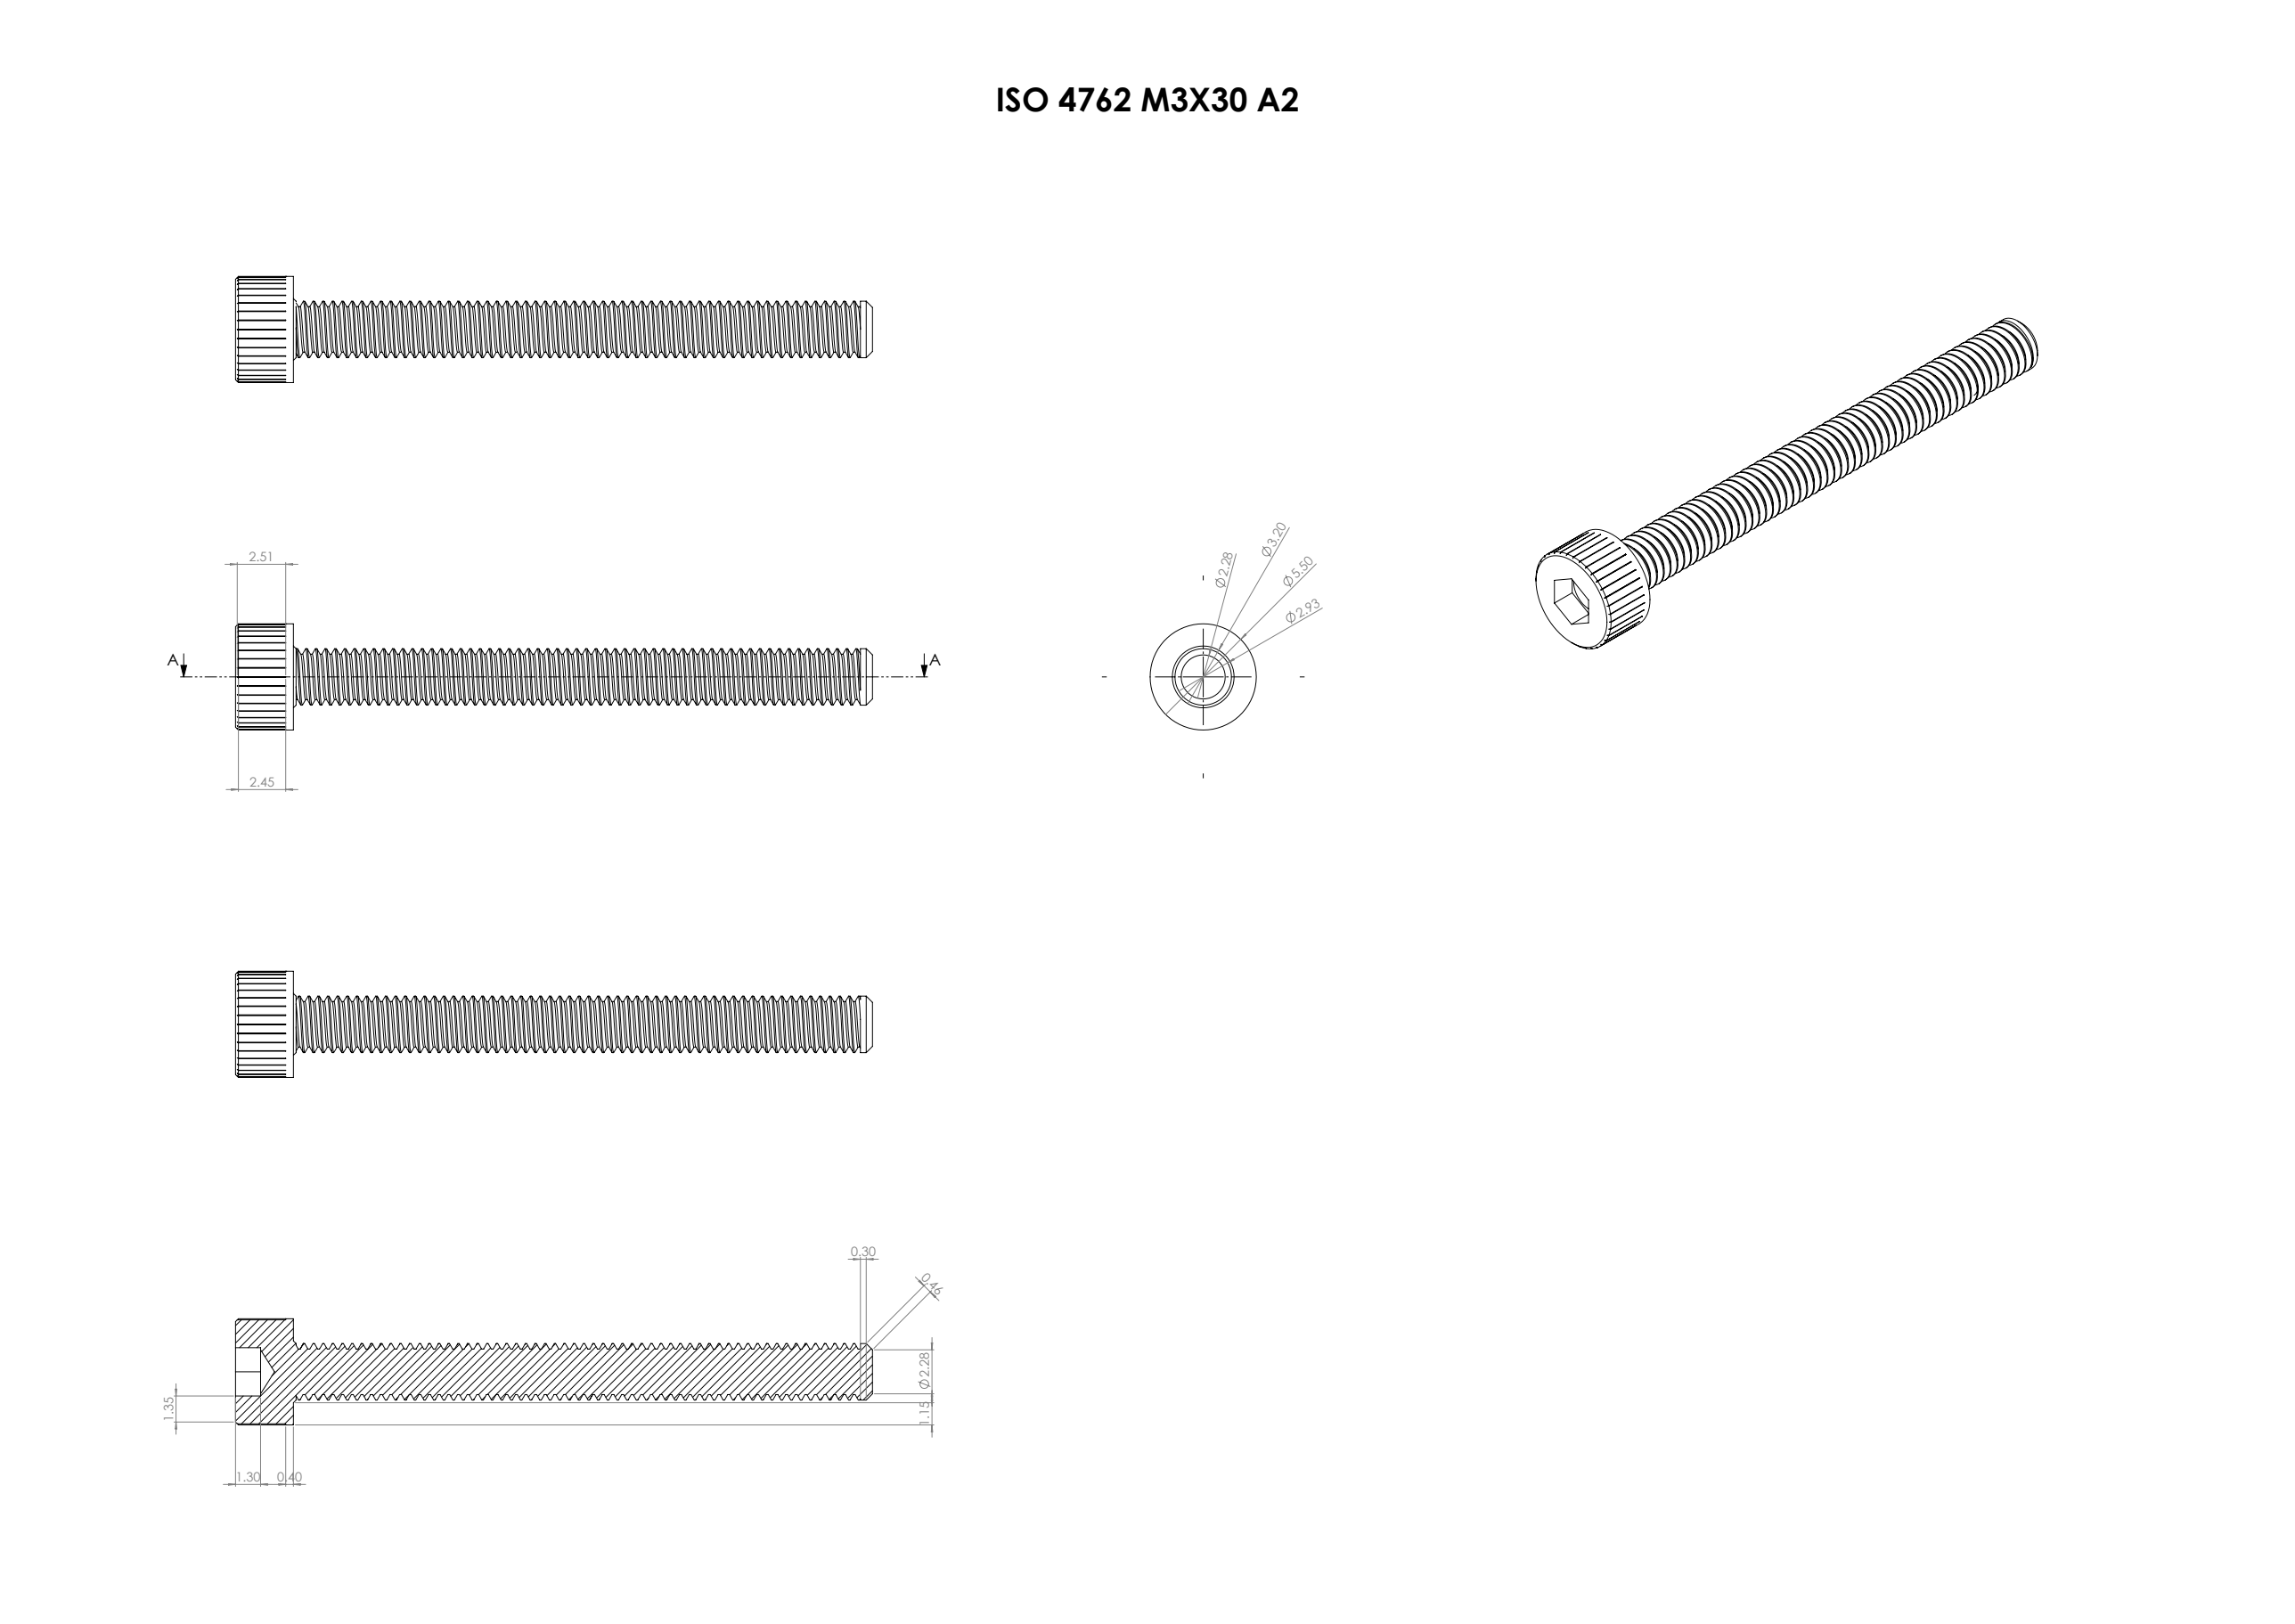
ISO-10303-21;
HEADER;
/* Generated by software containing ST-Developer
 * from STEP Tools, Inc. (www.steptools.com) 
 */

FILE_DESCRIPTION(
/* description */ (''),
/* implementation_level */ '2;1');

FILE_NAME(
/* name */ '15_ISO_4762_M3x30_A2.step',
/* time_stamp */ '2026-10-19T22:59:19-07:00',
/* author */ (''),
/* organization */ (''),
/* preprocessor_version */ 'ST-DEVELOPER v20.2',
/* originating_system */ 'Autodesk Translation Framework v15.15.0.0',
/* authorisation */ '');

FILE_SCHEMA (('AUTOMOTIVE_DESIGN { 1 0 10303 214 3 1 1 }'));
ENDSEC;

DATA;
#10=MECHANICAL_DESIGN_GEOMETRIC_PRESENTATION_REPRESENTATION('',(#925),#53650);
#219=(
BOUNDED_CURVE()
B_SPLINE_CURVE(2,(#49244,#49245,#49246),.UNSPECIFIED.,.F.,.F.)
B_SPLINE_CURVE_WITH_KNOTS((3,3),(0.,0.00848409808460555),.UNSPECIFIED.)
CURVE()
GEOMETRIC_REPRESENTATION_ITEM()
RATIONAL_B_SPLINE_CURVE((1.,1.00016582969981,1.00020138402525))
REPRESENTATION_ITEM('')
);
#220=(
BOUNDED_CURVE()
B_SPLINE_CURVE(2,(#49250,#49251,#49252),.UNSPECIFIED.,.F.,.F.)
B_SPLINE_CURVE_WITH_KNOTS((3,3),(0.0131150022108642,0.0215991002954745),
 .UNSPECIFIED.)
CURVE()
GEOMETRIC_REPRESENTATION_ITEM()
RATIONAL_B_SPLINE_CURVE((1.0002013840307,1.00016582970429,1.))
REPRESENTATION_ITEM('')
);
#221=(
BOUNDED_CURVE()
B_SPLINE_CURVE(2,(#49265,#49266,#49267),.UNSPECIFIED.,.F.,.F.)
B_SPLINE_CURVE_WITH_KNOTS((3,3),(0.,0.0084840980845983),.UNSPECIFIED.)
CURVE()
GEOMETRIC_REPRESENTATION_ITEM()
RATIONAL_B_SPLINE_CURVE((1.,1.00016582970166,1.00020138402749))
REPRESENTATION_ITEM('')
);
#222=(
BOUNDED_CURVE()
B_SPLINE_CURVE(2,(#49271,#49272,#49273),.UNSPECIFIED.,.F.,.F.)
B_SPLINE_CURVE_WITH_KNOTS((3,3),(0.0131150022108621,0.0215991002954745),
 .UNSPECIFIED.)
CURVE()
GEOMETRIC_REPRESENTATION_ITEM()
RATIONAL_B_SPLINE_CURVE((1.00020138404061,1.00016582971246,1.))
REPRESENTATION_ITEM('')
);
#223=(
BOUNDED_CURVE()
B_SPLINE_CURVE(2,(#49286,#49287,#49288),.UNSPECIFIED.,.F.,.F.)
B_SPLINE_CURVE_WITH_KNOTS((3,3),(0.,0.0084840980847528),.UNSPECIFIED.)
CURVE()
GEOMETRIC_REPRESENTATION_ITEM()
RATIONAL_B_SPLINE_CURVE((1.,1.00016582970549,1.00020138403215))
REPRESENTATION_ITEM('')
);
#224=(
BOUNDED_CURVE()
B_SPLINE_CURVE(2,(#49292,#49293,#49294),.UNSPECIFIED.,.F.,.F.)
B_SPLINE_CURVE_WITH_KNOTS((3,3),(0.0131150022108369,0.0215991002954744),
 .UNSPECIFIED.)
CURVE()
GEOMETRIC_REPRESENTATION_ITEM()
RATIONAL_B_SPLINE_CURVE((1.00020138403309,1.00016582970627,1.))
REPRESENTATION_ITEM('')
);
#225=(
BOUNDED_CURVE()
B_SPLINE_CURVE(2,(#49307,#49308,#49309),.UNSPECIFIED.,.F.,.F.)
B_SPLINE_CURVE_WITH_KNOTS((3,3),(0.,0.00848409808456441),.UNSPECIFIED.)
CURVE()
GEOMETRIC_REPRESENTATION_ITEM()
RATIONAL_B_SPLINE_CURVE((1.,1.00016582971128,1.00020138403918))
REPRESENTATION_ITEM('')
);
#226=(
BOUNDED_CURVE()
B_SPLINE_CURVE(2,(#49313,#49314,#49315),.UNSPECIFIED.,.F.,.F.)
B_SPLINE_CURVE_WITH_KNOTS((3,3),(0.0131150022107445,0.0215991002954745),
 .UNSPECIFIED.)
CURVE()
GEOMETRIC_REPRESENTATION_ITEM()
RATIONAL_B_SPLINE_CURVE((1.00020138401994,1.00016582969544,1.))
REPRESENTATION_ITEM('')
);
#227=(
BOUNDED_CURVE()
B_SPLINE_CURVE(2,(#49328,#49329,#49330),.UNSPECIFIED.,.F.,.F.)
B_SPLINE_CURVE_WITH_KNOTS((3,3),(0.,0.00848409808454028),.UNSPECIFIED.)
CURVE()
GEOMETRIC_REPRESENTATION_ITEM()
RATIONAL_B_SPLINE_CURVE((1.,1.00016582970383,1.00020138403013))
REPRESENTATION_ITEM('')
);
#228=(
BOUNDED_CURVE()
B_SPLINE_CURVE(2,(#49334,#49335,#49336),.UNSPECIFIED.,.F.,.F.)
B_SPLINE_CURVE_WITH_KNOTS((3,3),(0.0131150022108609,0.0215991002954744),
 .UNSPECIFIED.)
CURVE()
GEOMETRIC_REPRESENTATION_ITEM()
RATIONAL_B_SPLINE_CURVE((1.00020138403313,1.0001658297063,1.))
REPRESENTATION_ITEM('')
);
#229=(
BOUNDED_CURVE()
B_SPLINE_CURVE(2,(#49349,#49350,#49351),.UNSPECIFIED.,.F.,.F.)
B_SPLINE_CURVE_WITH_KNOTS((3,3),(0.,0.00848409808447202),.UNSPECIFIED.)
CURVE()
GEOMETRIC_REPRESENTATION_ITEM()
RATIONAL_B_SPLINE_CURVE((1.,1.00016582970768,1.00020138403481))
REPRESENTATION_ITEM('')
);
#230=(
BOUNDED_CURVE()
B_SPLINE_CURVE(2,(#49355,#49356,#49357),.UNSPECIFIED.,.F.,.F.)
B_SPLINE_CURVE_WITH_KNOTS((3,3),(0.0131150022108224,0.0215991002954744),
 .UNSPECIFIED.)
CURVE()
GEOMETRIC_REPRESENTATION_ITEM()
RATIONAL_B_SPLINE_CURVE((1.00020138403609,1.00016582970874,1.))
REPRESENTATION_ITEM('')
);
#231=(
BOUNDED_CURVE()
B_SPLINE_CURVE(2,(#49370,#49371,#49372),.UNSPECIFIED.,.F.,.F.)
B_SPLINE_CURVE_WITH_KNOTS((3,3),(0.,0.00848409808427833),.UNSPECIFIED.)
CURVE()
GEOMETRIC_REPRESENTATION_ITEM()
RATIONAL_B_SPLINE_CURVE((1.,1.00016582970634,1.00020138403319))
REPRESENTATION_ITEM('')
);
#232=(
BOUNDED_CURVE()
B_SPLINE_CURVE(2,(#49376,#49377,#49378),.UNSPECIFIED.,.F.,.F.)
B_SPLINE_CURVE_WITH_KNOTS((3,3),(0.013115002210556,0.0215991002954744),
 .UNSPECIFIED.)
CURVE()
GEOMETRIC_REPRESENTATION_ITEM()
RATIONAL_B_SPLINE_CURVE((1.00020138403007,1.00016582970378,1.))
REPRESENTATION_ITEM('')
);
#233=(
BOUNDED_CURVE()
B_SPLINE_CURVE(2,(#49391,#49392,#49393),.UNSPECIFIED.,.F.,.F.)
B_SPLINE_CURVE_WITH_KNOTS((3,3),(0.,0.00848409808441644),.UNSPECIFIED.)
CURVE()
GEOMETRIC_REPRESENTATION_ITEM()
RATIONAL_B_SPLINE_CURVE((1.,1.00016582971078,1.00020138403858))
REPRESENTATION_ITEM('')
);
#234=(
BOUNDED_CURVE()
B_SPLINE_CURVE(2,(#49397,#49398,#49399),.UNSPECIFIED.,.F.,.F.)
B_SPLINE_CURVE_WITH_KNOTS((3,3),(0.0131150022111809,0.0215991002954744),
 .UNSPECIFIED.)
CURVE()
GEOMETRIC_REPRESENTATION_ITEM()
RATIONAL_B_SPLINE_CURVE((1.00020138403856,1.00016582971077,1.))
REPRESENTATION_ITEM('')
);
#235=(
BOUNDED_CURVE()
B_SPLINE_CURVE(2,(#49412,#49413,#49414),.UNSPECIFIED.,.F.,.F.)
B_SPLINE_CURVE_WITH_KNOTS((3,3),(0.,0.00848409808461716),.UNSPECIFIED.)
CURVE()
GEOMETRIC_REPRESENTATION_ITEM()
RATIONAL_B_SPLINE_CURVE((1.,1.00016582970495,1.00020138403149))
REPRESENTATION_ITEM('')
);
#236=(
BOUNDED_CURVE()
B_SPLINE_CURVE(2,(#49418,#49419,#49420),.UNSPECIFIED.,.F.,.F.)
B_SPLINE_CURVE_WITH_KNOTS((3,3),(0.0131150022109262,0.0215991002954744),
 .UNSPECIFIED.)
CURVE()
GEOMETRIC_REPRESENTATION_ITEM()
RATIONAL_B_SPLINE_CURVE((1.00020138404239,1.00016582971392,1.))
REPRESENTATION_ITEM('')
);
#237=(
BOUNDED_CURVE()
B_SPLINE_CURVE(2,(#49433,#49434,#49435),.UNSPECIFIED.,.F.,.F.)
B_SPLINE_CURVE_WITH_KNOTS((3,3),(0.,0.00848409808431464),.UNSPECIFIED.)
CURVE()
GEOMETRIC_REPRESENTATION_ITEM()
RATIONAL_B_SPLINE_CURVE((1.,1.00016582970871,1.00020138403606))
REPRESENTATION_ITEM('')
);
#238=(
BOUNDED_CURVE()
B_SPLINE_CURVE(2,(#49439,#49440,#49441),.UNSPECIFIED.,.F.,.F.)
B_SPLINE_CURVE_WITH_KNOTS((3,3),(0.0131150022106601,0.0215991002954745),
 .UNSPECIFIED.)
CURVE()
GEOMETRIC_REPRESENTATION_ITEM()
RATIONAL_B_SPLINE_CURVE((1.00020138402617,1.00016582970057,1.))
REPRESENTATION_ITEM('')
);
#239=(
BOUNDED_CURVE()
B_SPLINE_CURVE(2,(#49454,#49455,#49456),.UNSPECIFIED.,.F.,.F.)
B_SPLINE_CURVE_WITH_KNOTS((3,3),(0.,0.00848409808479875),.UNSPECIFIED.)
CURVE()
GEOMETRIC_REPRESENTATION_ITEM()
RATIONAL_B_SPLINE_CURVE((1.,1.00016582970535,1.00020138403197))
REPRESENTATION_ITEM('')
);
#240=(
BOUNDED_CURVE()
B_SPLINE_CURVE(2,(#49460,#49461,#49462),.UNSPECIFIED.,.F.,.F.)
B_SPLINE_CURVE_WITH_KNOTS((3,3),(0.0131150022108306,0.0215991002954744),
 .UNSPECIFIED.)
CURVE()
GEOMETRIC_REPRESENTATION_ITEM()
RATIONAL_B_SPLINE_CURVE((1.00020138403405,1.00016582970706,1.))
REPRESENTATION_ITEM('')
);
#241=(
BOUNDED_CURVE()
B_SPLINE_CURVE(2,(#49475,#49476,#49477),.UNSPECIFIED.,.F.,.F.)
B_SPLINE_CURVE_WITH_KNOTS((3,3),(0.,0.0084840980847528),.UNSPECIFIED.)
CURVE()
GEOMETRIC_REPRESENTATION_ITEM()
RATIONAL_B_SPLINE_CURVE((1.,1.00016582970549,1.00020138403215))
REPRESENTATION_ITEM('')
);
#242=(
BOUNDED_CURVE()
B_SPLINE_CURVE(2,(#49481,#49482,#49483),.UNSPECIFIED.,.F.,.F.)
B_SPLINE_CURVE_WITH_KNOTS((3,3),(0.0131150022108369,0.0215991002954744),
 .UNSPECIFIED.)
CURVE()
GEOMETRIC_REPRESENTATION_ITEM()
RATIONAL_B_SPLINE_CURVE((1.00020138403309,1.00016582970627,1.))
REPRESENTATION_ITEM('')
);
#243=(
BOUNDED_CURVE()
B_SPLINE_CURVE(2,(#49496,#49497,#49498),.UNSPECIFIED.,.F.,.F.)
B_SPLINE_CURVE_WITH_KNOTS((3,3),(0.,0.0084840980842322),.UNSPECIFIED.)
CURVE()
GEOMETRIC_REPRESENTATION_ITEM()
RATIONAL_B_SPLINE_CURVE((1.,1.00016582971394,1.00020138404241))
REPRESENTATION_ITEM('')
);
#244=(
BOUNDED_CURVE()
B_SPLINE_CURVE(2,(#49502,#49503,#49504),.UNSPECIFIED.,.F.,.F.)
B_SPLINE_CURVE_WITH_KNOTS((3,3),(0.0131150022105481,0.0215991002954744),
 .UNSPECIFIED.)
CURVE()
GEOMETRIC_REPRESENTATION_ITEM()
RATIONAL_B_SPLINE_CURVE((1.00020138402709,1.00016582970133,1.))
REPRESENTATION_ITEM('')
);
#245=(
BOUNDED_CURVE()
B_SPLINE_CURVE(2,(#49517,#49518,#49519),.UNSPECIFIED.,.F.,.F.)
B_SPLINE_CURVE_WITH_KNOTS((3,3),(0.,0.00848409808414784),.UNSPECIFIED.)
CURVE()
GEOMETRIC_REPRESENTATION_ITEM()
RATIONAL_B_SPLINE_CURVE((1.,1.00016582970969,1.00020138403725))
REPRESENTATION_ITEM('')
);
#246=(
BOUNDED_CURVE()
B_SPLINE_CURVE(2,(#49523,#49524,#49525),.UNSPECIFIED.,.F.,.F.)
B_SPLINE_CURVE_WITH_KNOTS((3,3),(0.0131150022106295,0.0215991002954744),
 .UNSPECIFIED.)
CURVE()
GEOMETRIC_REPRESENTATION_ITEM()
RATIONAL_B_SPLINE_CURVE((1.00020138402686,1.00016582970114,1.))
REPRESENTATION_ITEM('')
);
#247=(
BOUNDED_CURVE()
B_SPLINE_CURVE(2,(#49538,#49539,#49540),.UNSPECIFIED.,.F.,.F.)
B_SPLINE_CURVE_WITH_KNOTS((3,3),(0.,0.00848409808445945),.UNSPECIFIED.)
CURVE()
GEOMETRIC_REPRESENTATION_ITEM()
RATIONAL_B_SPLINE_CURVE((1.,1.00016582971029,1.00020138403798))
REPRESENTATION_ITEM('')
);
#248=(
BOUNDED_CURVE()
B_SPLINE_CURVE(2,(#49544,#49545,#49546),.UNSPECIFIED.,.F.,.F.)
B_SPLINE_CURVE_WITH_KNOTS((3,3),(0.0131150022108553,0.0215991002954744),
 .UNSPECIFIED.)
CURVE()
GEOMETRIC_REPRESENTATION_ITEM()
RATIONAL_B_SPLINE_CURVE((1.00020138402807,1.00016582970213,1.))
REPRESENTATION_ITEM('')
);
#249=(
BOUNDED_CURVE()
B_SPLINE_CURVE(2,(#49559,#49560,#49561),.UNSPECIFIED.,.F.,.F.)
B_SPLINE_CURVE_WITH_KNOTS((3,3),(0.,0.00848409808448244),.UNSPECIFIED.)
CURVE()
GEOMETRIC_REPRESENTATION_ITEM()
RATIONAL_B_SPLINE_CURVE((1.,1.00016582970044,1.00020138402602))
REPRESENTATION_ITEM('')
);
#250=(
BOUNDED_CURVE()
B_SPLINE_CURVE(2,(#49565,#49566,#49567),.UNSPECIFIED.,.F.,.F.)
B_SPLINE_CURVE_WITH_KNOTS((3,3),(0.0131150022107,0.0215991002954745),
 .UNSPECIFIED.)
CURVE()
GEOMETRIC_REPRESENTATION_ITEM()
RATIONAL_B_SPLINE_CURVE((1.00020138402745,1.00016582970163,1.))
REPRESENTATION_ITEM('')
);
#251=(
BOUNDED_CURVE()
B_SPLINE_CURVE(2,(#49580,#49581,#49582),.UNSPECIFIED.,.F.,.F.)
B_SPLINE_CURVE_WITH_KNOTS((3,3),(0.,0.0084840980844404),.UNSPECIFIED.)
CURVE()
GEOMETRIC_REPRESENTATION_ITEM()
RATIONAL_B_SPLINE_CURVE((1.,1.00016582969984,1.00020138402529))
REPRESENTATION_ITEM('')
);
#252=(
BOUNDED_CURVE()
B_SPLINE_CURVE(2,(#49586,#49587,#49588),.UNSPECIFIED.,.F.,.F.)
B_SPLINE_CURVE_WITH_KNOTS((3,3),(0.0131150022109728,0.0215991002954744),
 .UNSPECIFIED.)
CURVE()
GEOMETRIC_REPRESENTATION_ITEM()
RATIONAL_B_SPLINE_CURVE((1.00020138403593,1.0001658297086,1.))
REPRESENTATION_ITEM('')
);
#253=(
BOUNDED_CURVE()
B_SPLINE_CURVE(2,(#49603,#49604,#49605),.UNSPECIFIED.,.F.,.F.)
B_SPLINE_CURVE_WITH_KNOTS((3,3),(0.,0.00848409808461716),.UNSPECIFIED.)
CURVE()
GEOMETRIC_REPRESENTATION_ITEM()
RATIONAL_B_SPLINE_CURVE((1.,1.00016582970494,1.00020138403149))
REPRESENTATION_ITEM('')
);
#254=(
BOUNDED_CURVE()
B_SPLINE_CURVE(2,(#49609,#49610,#49611),.UNSPECIFIED.,.F.,.F.)
B_SPLINE_CURVE_WITH_KNOTS((3,3),(0.0131150022107313,0.0215991002954744),
 .UNSPECIFIED.)
CURVE()
GEOMETRIC_REPRESENTATION_ITEM()
RATIONAL_B_SPLINE_CURVE((1.00020138404435,1.00016582971554,1.))
REPRESENTATION_ITEM('')
);
#255=(
BOUNDED_CURVE()
B_SPLINE_CURVE(2,(#49624,#49625,#49626),.UNSPECIFIED.,.F.,.F.)
B_SPLINE_CURVE_WITH_KNOTS((3,3),(0.,0.0084840980847339),.UNSPECIFIED.)
CURVE()
GEOMETRIC_REPRESENTATION_ITEM()
RATIONAL_B_SPLINE_CURVE((1.,1.00016582970597,1.00020138403273))
REPRESENTATION_ITEM('')
);
#256=(
BOUNDED_CURVE()
B_SPLINE_CURVE(2,(#49630,#49631,#49632),.UNSPECIFIED.,.F.,.F.)
B_SPLINE_CURVE_WITH_KNOTS((3,3),(0.0131150022106966,0.0215991002954744),
 .UNSPECIFIED.)
CURVE()
GEOMETRIC_REPRESENTATION_ITEM()
RATIONAL_B_SPLINE_CURVE((1.00020138403392,1.00016582970695,1.))
REPRESENTATION_ITEM('')
);
#257=(
BOUNDED_CURVE()
B_SPLINE_CURVE(2,(#49645,#49646,#49647),.UNSPECIFIED.,.F.,.F.)
B_SPLINE_CURVE_WITH_KNOTS((3,3),(0.,0.00848409808458664),.UNSPECIFIED.)
CURVE()
GEOMETRIC_REPRESENTATION_ITEM()
RATIONAL_B_SPLINE_CURVE((1.,1.00016582970477,1.00020138403127))
REPRESENTATION_ITEM('')
);
#258=(
BOUNDED_CURVE()
B_SPLINE_CURVE(2,(#49651,#49652,#49653),.UNSPECIFIED.,.F.,.F.)
B_SPLINE_CURVE_WITH_KNOTS((3,3),(0.0131150022108393,0.0215991002954745),
 .UNSPECIFIED.)
CURVE()
GEOMETRIC_REPRESENTATION_ITEM()
RATIONAL_B_SPLINE_CURVE((1.00020138403572,1.00016582970843,1.))
REPRESENTATION_ITEM('')
);
#259=(
BOUNDED_CURVE()
B_SPLINE_CURVE(2,(#49666,#49667,#49668),.UNSPECIFIED.,.F.,.F.)
B_SPLINE_CURVE_WITH_KNOTS((3,3),(0.,0.00848409808463718),.UNSPECIFIED.)
CURVE()
GEOMETRIC_REPRESENTATION_ITEM()
RATIONAL_B_SPLINE_CURVE((1.,1.00016582970055,1.00020138402615))
REPRESENTATION_ITEM('')
);
#260=(
BOUNDED_CURVE()
B_SPLINE_CURVE(2,(#49672,#49673,#49674),.UNSPECIFIED.,.F.,.F.)
B_SPLINE_CURVE_WITH_KNOTS((3,3),(0.013115002211021,0.0215991002954743),
 .UNSPECIFIED.)
CURVE()
GEOMETRIC_REPRESENTATION_ITEM()
RATIONAL_B_SPLINE_CURVE((1.00020138403351,1.00016582970661,1.))
REPRESENTATION_ITEM('')
);
#261=(
BOUNDED_CURVE()
B_SPLINE_CURVE(2,(#49687,#49688,#49689),.UNSPECIFIED.,.F.,.F.)
B_SPLINE_CURVE_WITH_KNOTS((3,3),(0.,0.0084840980842322),.UNSPECIFIED.)
CURVE()
GEOMETRIC_REPRESENTATION_ITEM()
RATIONAL_B_SPLINE_CURVE((1.,1.00016582971394,1.00020138404241))
REPRESENTATION_ITEM('')
);
#262=(
BOUNDED_CURVE()
B_SPLINE_CURVE(2,(#49693,#49694,#49695),.UNSPECIFIED.,.F.,.F.)
B_SPLINE_CURVE_WITH_KNOTS((3,3),(0.0131150022105481,0.0215991002954744),
 .UNSPECIFIED.)
CURVE()
GEOMETRIC_REPRESENTATION_ITEM()
RATIONAL_B_SPLINE_CURVE((1.00020138402709,1.00016582970133,1.))
REPRESENTATION_ITEM('')
);
#263=(
BOUNDED_CURVE()
B_SPLINE_CURVE(2,(#49708,#49709,#49710),.UNSPECIFIED.,.F.,.F.)
B_SPLINE_CURVE_WITH_KNOTS((3,3),(0.,0.00848409808456074),.UNSPECIFIED.)
CURVE()
GEOMETRIC_REPRESENTATION_ITEM()
RATIONAL_B_SPLINE_CURVE((1.,1.00016582970947,1.00020138403699))
REPRESENTATION_ITEM('')
);
#264=(
BOUNDED_CURVE()
B_SPLINE_CURVE(2,(#49714,#49715,#49716),.UNSPECIFIED.,.F.,.F.)
B_SPLINE_CURVE_WITH_KNOTS((3,3),(0.0131150022109338,0.0215991002954745),
 .UNSPECIFIED.)
CURVE()
GEOMETRIC_REPRESENTATION_ITEM()
RATIONAL_B_SPLINE_CURVE((1.00020138403466,1.00016582970756,1.))
REPRESENTATION_ITEM('')
);
#265=(
BOUNDED_CURVE()
B_SPLINE_CURVE(2,(#49729,#49730,#49731),.UNSPECIFIED.,.F.,.F.)
B_SPLINE_CURVE_WITH_KNOTS((3,3),(0.,0.00848409808446819),.UNSPECIFIED.)
CURVE()
GEOMETRIC_REPRESENTATION_ITEM()
RATIONAL_B_SPLINE_CURVE((1.,1.00016582970737,1.00020138403444))
REPRESENTATION_ITEM('')
);
#266=(
BOUNDED_CURVE()
B_SPLINE_CURVE(2,(#49735,#49736,#49737),.UNSPECIFIED.,.F.,.F.)
B_SPLINE_CURVE_WITH_KNOTS((3,3),(0.0131150022107308,0.0215991002954744),
 .UNSPECIFIED.)
CURVE()
GEOMETRIC_REPRESENTATION_ITEM()
RATIONAL_B_SPLINE_CURVE((1.00020138402973,1.0001658297035,1.))
REPRESENTATION_ITEM('')
);
#267=(
BOUNDED_CURVE()
B_SPLINE_CURVE(2,(#49750,#49751,#49752),.UNSPECIFIED.,.F.,.F.)
B_SPLINE_CURVE_WITH_KNOTS((3,3),(0.,0.00848409808448244),.UNSPECIFIED.)
CURVE()
GEOMETRIC_REPRESENTATION_ITEM()
RATIONAL_B_SPLINE_CURVE((1.,1.00016582970044,1.00020138402602))
REPRESENTATION_ITEM('')
);
#268=(
BOUNDED_CURVE()
B_SPLINE_CURVE(2,(#49756,#49757,#49758),.UNSPECIFIED.,.F.,.F.)
B_SPLINE_CURVE_WITH_KNOTS((3,3),(0.0131150022107,0.0215991002954745),
 .UNSPECIFIED.)
CURVE()
GEOMETRIC_REPRESENTATION_ITEM()
RATIONAL_B_SPLINE_CURVE((1.00020138402745,1.00016582970163,1.))
REPRESENTATION_ITEM('')
);
#269=(
BOUNDED_CURVE()
B_SPLINE_CURVE(2,(#49771,#49772,#49773),.UNSPECIFIED.,.F.,.F.)
B_SPLINE_CURVE_WITH_KNOTS((3,3),(0.,0.00848409808441086),.UNSPECIFIED.)
CURVE()
GEOMETRIC_REPRESENTATION_ITEM()
RATIONAL_B_SPLINE_CURVE((1.,1.00016582971069,1.00020138403846))
REPRESENTATION_ITEM('')
);
#270=(
BOUNDED_CURVE()
B_SPLINE_CURVE(2,(#49777,#49778,#49779),.UNSPECIFIED.,.F.,.F.)
B_SPLINE_CURVE_WITH_KNOTS((3,3),(0.0131150022109839,0.0215991002954745),
 .UNSPECIFIED.)
CURVE()
GEOMETRIC_REPRESENTATION_ITEM()
RATIONAL_B_SPLINE_CURVE((1.00020138402514,1.00016582969972,1.))
REPRESENTATION_ITEM('')
);
#271=(
BOUNDED_CURVE()
B_SPLINE_CURVE(2,(#49792,#49793,#49794),.UNSPECIFIED.,.F.,.F.)
B_SPLINE_CURVE_WITH_KNOTS((3,3),(0.,0.00848409808461089),.UNSPECIFIED.)
CURVE()
GEOMETRIC_REPRESENTATION_ITEM()
RATIONAL_B_SPLINE_CURVE((1.,1.00016582970996,1.00020138403757))
REPRESENTATION_ITEM('')
);
#272=(
BOUNDED_CURVE()
B_SPLINE_CURVE(2,(#49798,#49799,#49800),.UNSPECIFIED.,.F.,.F.)
B_SPLINE_CURVE_WITH_KNOTS((3,3),(0.0131150022107081,0.0215991002954744),
 .UNSPECIFIED.)
CURVE()
GEOMETRIC_REPRESENTATION_ITEM()
RATIONAL_B_SPLINE_CURVE((1.00020138403464,1.00016582970754,1.))
REPRESENTATION_ITEM('')
);
#273=(
BOUNDED_CURVE()
B_SPLINE_CURVE(2,(#49813,#49814,#49815),.UNSPECIFIED.,.F.,.F.)
B_SPLINE_CURVE_WITH_KNOTS((3,3),(0.,0.00848409808429742),.UNSPECIFIED.)
CURVE()
GEOMETRIC_REPRESENTATION_ITEM()
RATIONAL_B_SPLINE_CURVE((1.,1.00016582971405,1.00020138404255))
REPRESENTATION_ITEM('')
);
#274=(
BOUNDED_CURVE()
B_SPLINE_CURVE(2,(#49819,#49820,#49821),.UNSPECIFIED.,.F.,.F.)
B_SPLINE_CURVE_WITH_KNOTS((3,3),(0.0131150022109026,0.0215991002954744),
 .UNSPECIFIED.)
CURVE()
GEOMETRIC_REPRESENTATION_ITEM()
RATIONAL_B_SPLINE_CURVE((1.00020138403953,1.00016582971157,1.))
REPRESENTATION_ITEM('')
);
#275=(
BOUNDED_CURVE()
B_SPLINE_CURVE(2,(#49834,#49835,#49836),.UNSPECIFIED.,.F.,.F.)
B_SPLINE_CURVE_WITH_KNOTS((3,3),(0.,0.00848409808458664),.UNSPECIFIED.)
CURVE()
GEOMETRIC_REPRESENTATION_ITEM()
RATIONAL_B_SPLINE_CURVE((1.,1.00016582970477,1.00020138403127))
REPRESENTATION_ITEM('')
);
#276=(
BOUNDED_CURVE()
B_SPLINE_CURVE(2,(#49840,#49841,#49842),.UNSPECIFIED.,.F.,.F.)
B_SPLINE_CURVE_WITH_KNOTS((3,3),(0.0131150022108393,0.0215991002954745),
 .UNSPECIFIED.)
CURVE()
GEOMETRIC_REPRESENTATION_ITEM()
RATIONAL_B_SPLINE_CURVE((1.00020138403572,1.00016582970843,1.))
REPRESENTATION_ITEM('')
);
#277=(
BOUNDED_CURVE()
B_SPLINE_CURVE(2,(#49855,#49856,#49857),.UNSPECIFIED.,.F.,.F.)
B_SPLINE_CURVE_WITH_KNOTS((3,3),(0.,0.00848409808472772),.UNSPECIFIED.)
CURVE()
GEOMETRIC_REPRESENTATION_ITEM()
RATIONAL_B_SPLINE_CURVE((1.,1.00016582970133,1.0002013840271))
REPRESENTATION_ITEM('')
);
#278=(
BOUNDED_CURVE()
B_SPLINE_CURVE(2,(#49861,#49862,#49863),.UNSPECIFIED.,.F.,.F.)
B_SPLINE_CURVE_WITH_KNOTS((3,3),(0.0131150022106421,0.0215991002954744),
 .UNSPECIFIED.)
CURVE()
GEOMETRIC_REPRESENTATION_ITEM()
RATIONAL_B_SPLINE_CURVE((1.00020138403214,1.00016582970549,1.))
REPRESENTATION_ITEM('')
);
#279=(
BOUNDED_CURVE()
B_SPLINE_CURVE(2,(#49876,#49877,#49878),.UNSPECIFIED.,.F.,.F.)
B_SPLINE_CURVE_WITH_KNOTS((3,3),(0.,0.00848409808461495),.UNSPECIFIED.)
CURVE()
GEOMETRIC_REPRESENTATION_ITEM()
RATIONAL_B_SPLINE_CURVE((1.,1.00016582970949,1.000201384037))
REPRESENTATION_ITEM('')
);
#280=(
BOUNDED_CURVE()
B_SPLINE_CURVE(2,(#49882,#49883,#49884),.UNSPECIFIED.,.F.,.F.)
B_SPLINE_CURVE_WITH_KNOTS((3,3),(0.0131150022109445,0.0215991002954744),
 .UNSPECIFIED.)
CURVE()
GEOMETRIC_REPRESENTATION_ITEM()
RATIONAL_B_SPLINE_CURVE((1.00020138402523,1.00016582969979,1.))
REPRESENTATION_ITEM('')
);
#281=(
BOUNDED_CURVE()
B_SPLINE_CURVE(2,(#49897,#49898,#49899),.UNSPECIFIED.,.F.,.F.)
B_SPLINE_CURVE_WITH_KNOTS((3,3),(0.,0.00848409808414784),.UNSPECIFIED.)
CURVE()
GEOMETRIC_REPRESENTATION_ITEM()
RATIONAL_B_SPLINE_CURVE((1.,1.00016582970969,1.00020138403725))
REPRESENTATION_ITEM('')
);
#282=(
BOUNDED_CURVE()
B_SPLINE_CURVE(2,(#49903,#49904,#49905),.UNSPECIFIED.,.F.,.F.)
B_SPLINE_CURVE_WITH_KNOTS((3,3),(0.0131150022106295,0.0215991002954744),
 .UNSPECIFIED.)
CURVE()
GEOMETRIC_REPRESENTATION_ITEM()
RATIONAL_B_SPLINE_CURVE((1.00020138402686,1.00016582970114,1.))
REPRESENTATION_ITEM('')
);
#283=(
BOUNDED_CURVE()
B_SPLINE_CURVE(2,(#49918,#49919,#49920),.UNSPECIFIED.,.F.,.F.)
B_SPLINE_CURVE_WITH_KNOTS((3,3),(0.,0.00848409808467215),.UNSPECIFIED.)
CURVE()
GEOMETRIC_REPRESENTATION_ITEM()
RATIONAL_B_SPLINE_CURVE((1.,1.00016582970831,1.00020138403558))
REPRESENTATION_ITEM('')
);
#284=(
BOUNDED_CURVE()
B_SPLINE_CURVE(2,(#49924,#49925,#49926),.UNSPECIFIED.,.F.,.F.)
B_SPLINE_CURVE_WITH_KNOTS((3,3),(0.0131150022106657,0.0215991002954744),
 .UNSPECIFIED.)
CURVE()
GEOMETRIC_REPRESENTATION_ITEM()
RATIONAL_B_SPLINE_CURVE((1.00020138402665,1.00016582970096,1.))
REPRESENTATION_ITEM('')
);
#285=(
BOUNDED_CURVE()
B_SPLINE_CURVE(2,(#49939,#49940,#49941),.UNSPECIFIED.,.F.,.F.)
B_SPLINE_CURVE_WITH_KNOTS((3,3),(0.,0.00848409808448244),.UNSPECIFIED.)
CURVE()
GEOMETRIC_REPRESENTATION_ITEM()
RATIONAL_B_SPLINE_CURVE((1.,1.00016582970044,1.00020138402602))
REPRESENTATION_ITEM('')
);
#286=(
BOUNDED_CURVE()
B_SPLINE_CURVE(2,(#49945,#49946,#49947),.UNSPECIFIED.,.F.,.F.)
B_SPLINE_CURVE_WITH_KNOTS((3,3),(0.0131150022107,0.0215991002954745),
 .UNSPECIFIED.)
CURVE()
GEOMETRIC_REPRESENTATION_ITEM()
RATIONAL_B_SPLINE_CURVE((1.00020138402745,1.00016582970163,1.))
REPRESENTATION_ITEM('')
);
#287=(
BOUNDED_CURVE()
B_SPLINE_CURVE(2,(#49960,#49961,#49962),.UNSPECIFIED.,.F.,.F.)
B_SPLINE_CURVE_WITH_KNOTS((3,3),(0.,0.00848409808462521),.UNSPECIFIED.)
CURVE()
GEOMETRIC_REPRESENTATION_ITEM()
RATIONAL_B_SPLINE_CURVE((1.,1.00016582970203,1.00020138402795))
REPRESENTATION_ITEM('')
);
#288=(
BOUNDED_CURVE()
B_SPLINE_CURVE(2,(#49966,#49967,#49968),.UNSPECIFIED.,.F.,.F.)
B_SPLINE_CURVE_WITH_KNOTS((3,3),(0.0131150022109901,0.0215991002954744),
 .UNSPECIFIED.)
CURVE()
GEOMETRIC_REPRESENTATION_ITEM()
RATIONAL_B_SPLINE_CURVE((1.00020138403892,1.00016582971107,1.))
REPRESENTATION_ITEM('')
);
#289=(
BOUNDED_CURVE()
B_SPLINE_CURVE(2,(#50021,#50022,#50023),.UNSPECIFIED.,.F.,.F.)
B_SPLINE_CURVE_WITH_KNOTS((3,3),(0.,0.0084840980844225),.UNSPECIFIED.)
CURVE()
GEOMETRIC_REPRESENTATION_ITEM()
RATIONAL_B_SPLINE_CURVE((1.,1.00016582970633,1.00020138403317))
REPRESENTATION_ITEM('')
);
#290=(
BOUNDED_CURVE()
B_SPLINE_CURVE(2,(#50025,#50026,#50027),.UNSPECIFIED.,.F.,.F.)
B_SPLINE_CURVE_WITH_KNOTS((3,3),(0.0131150022108769,0.0215991002954744),
 .UNSPECIFIED.)
CURVE()
GEOMETRIC_REPRESENTATION_ITEM()
RATIONAL_B_SPLINE_CURVE((1.00020138402781,1.00016582970192,1.))
REPRESENTATION_ITEM('')
);
#369=B_SPLINE_SURFACE_WITH_KNOTS('',3,3,((#46095,#46096,#46097,#46098,#46099,
#46100,#46101,#46102,#46103,#46104,#46105,#46106,#46107,#46108,#46109,#46110,
#46111,#46112,#46113,#46114,#46115,#46116,#46117,#46118,#46119,#46120,#46121,
#46122,#46123,#46124,#46125,#46126,#46127,#46128,#46129,#46130,#46131,#46132,
#46133,#46134,#46135,#46136,#46137,#46138,#46139,#46140,#46141,#46142,#46143,
#46144,#46145,#46146,#46147,#46148,#46149,#46150,#46151,#46152,#46153,#46154,
#46155,#46156,#46157,#46158,#46159,#46160,#46161,#46162,#46163,#46164,#46165,
#46166,#46167,#46168,#46169,#46170,#46171,#46172,#46173,#46174,#46175,#46176,
#46177,#46178,#46179,#46180,#46181,#46182,#46183,#46184,#46185,#46186,#46187,
#46188,#46189,#46190,#46191,#46192,#46193,#46194,#46195,#46196,#46197,#46198,
#46199,#46200,#46201,#46202,#46203,#46204,#46205,#46206,#46207,#46208,#46209,
#46210,#46211,#46212,#46213,#46214,#46215,#46216,#46217,#46218,#46219,#46220,
#46221,#46222,#46223,#46224,#46225,#46226,#46227,#46228,#46229,#46230,#46231,
#46232,#46233,#46234,#46235,#46236,#46237,#46238,#46239,#46240,#46241,#46242,
#46243,#46244,#46245,#46246,#46247,#46248,#46249,#46250,#46251,#46252,#46253,
#46254,#46255,#46256,#46257,#46258,#46259,#46260,#46261,#46262,#46263,#46264,
#46265,#46266,#46267,#46268,#46269,#46270,#46271,#46272,#46273,#46274,#46275,
#46276,#46277,#46278,#46279,#46280,#46281,#46282,#46283,#46284,#46285,#46286,
#46287,#46288,#46289,#46290,#46291,#46292,#46293,#46294,#46295,#46296,#46297,
#46298,#46299,#46300,#46301,#46302,#46303,#46304,#46305,#46306,#46307,#46308,
#46309,#46310,#46311,#46312,#46313,#46314,#46315,#46316,#46317,#46318,#46319,
#46320,#46321,#46322,#46323,#46324,#46325,#46326,#46327,#46328,#46329,#46330,
#46331,#46332,#46333,#46334,#46335,#46336,#46337,#46338,#46339,#46340,#46341,
#46342,#46343,#46344,#46345,#46346,#46347,#46348,#46349,#46350,#46351,#46352,
#46353,#46354,#46355,#46356,#46357,#46358,#46359,#46360,#46361,#46362,#46363,
#46364,#46365,#46366,#46367,#46368,#46369,#46370,#46371,#46372,#46373,#46374,
#46375,#46376,#46377,#46378,#46379,#46380,#46381,#46382,#46383,#46384,#46385,
#46386,#46387,#46388,#46389,#46390,#46391,#46392,#46393,#46394,#46395,#46396,
#46397,#46398,#46399,#46400,#46401,#46402,#46403,#46404,#46405,#46406,#46407,
#46408,#46409,#46410,#46411,#46412,#46413,#46414,#46415,#46416,#46417,#46418,
#46419,#46420,#46421,#46422,#46423,#46424,#46425,#46426,#46427,#46428,#46429,
#46430,#46431,#46432,#46433,#46434,#46435,#46436,#46437,#46438,#46439,#46440,
#46441,#46442,#46443,#46444,#46445,#46446,#46447,#46448,#46449,#46450,#46451,
#46452,#46453,#46454,#46455,#46456,#46457,#46458,#46459,#46460,#46461,#46462,
#46463,#46464,#46465,#46466,#46467),(#46468,#46469,#46470,#46471,#46472,
#46473,#46474,#46475,#46476,#46477,#46478,#46479,#46480,#46481,#46482,#46483,
#46484,#46485,#46486,#46487,#46488,#46489,#46490,#46491,#46492,#46493,#46494,
#46495,#46496,#46497,#46498,#46499,#46500,#46501,#46502,#46503,#46504,#46505,
#46506,#46507,#46508,#46509,#46510,#46511,#46512,#46513,#46514,#46515,#46516,
#46517,#46518,#46519,#46520,#46521,#46522,#46523,#46524,#46525,#46526,#46527,
#46528,#46529,#46530,#46531,#46532,#46533,#46534,#46535,#46536,#46537,#46538,
#46539,#46540,#46541,#46542,#46543,#46544,#46545,#46546,#46547,#46548,#46549,
#46550,#46551,#46552,#46553,#46554,#46555,#46556,#46557,#46558,#46559,#46560,
#46561,#46562,#46563,#46564,#46565,#46566,#46567,#46568,#46569,#46570,#46571,
#46572,#46573,#46574,#46575,#46576,#46577,#46578,#46579,#46580,#46581,#46582,
#46583,#46584,#46585,#46586,#46587,#46588,#46589,#46590,#46591,#46592,#46593,
#46594,#46595,#46596,#46597,#46598,#46599,#46600,#46601,#46602,#46603,#46604,
#46605,#46606,#46607,#46608,#46609,#46610,#46611,#46612,#46613,#46614,#46615,
#46616,#46617,#46618,#46619,#46620,#46621,#46622,#46623,#46624,#46625,#46626,
#46627,#46628,#46629,#46630,#46631,#46632,#46633,#46634,#46635,#46636,#46637,
#46638,#46639,#46640,#46641,#46642,#46643,#46644,#46645,#46646,#46647,#46648,
#46649,#46650,#46651,#46652,#46653,#46654,#46655,#46656,#46657,#46658,#46659,
#46660,#46661,#46662,#46663,#46664,#46665,#46666,#46667,#46668,#46669,#46670,
#46671,#46672,#46673,#46674,#46675,#46676,#46677,#46678,#46679,#46680,#46681,
#46682,#46683,#46684,#46685,#46686,#46687,#46688,#46689,#46690,#46691,#46692,
#46693,#46694,#46695,#46696,#46697,#46698,#46699,#46700,#46701,#46702,#46703,
#46704,#46705,#46706,#46707,#46708,#46709,#46710,#46711,#46712,#46713,#46714,
#46715,#46716,#46717,#46718,#46719,#46720,#46721,#46722,#46723,#46724,#46725,
#46726,#46727,#46728,#46729,#46730,#46731,#46732,#46733,#46734,#46735,#46736,
#46737,#46738,#46739,#46740,#46741,#46742,#46743,#46744,#46745,#46746,#46747,
#46748,#46749,#46750,#46751,#46752,#46753,#46754,#46755,#46756,#46757,#46758,
#46759,#46760,#46761,#46762,#46763,#46764,#46765,#46766,#46767,#46768,#46769,
#46770,#46771,#46772,#46773,#46774,#46775,#46776,#46777,#46778,#46779,#46780,
#46781,#46782,#46783,#46784,#46785,#46786,#46787,#46788,#46789,#46790,#46791,
#46792,#46793,#46794,#46795,#46796,#46797,#46798,#46799,#46800,#46801,#46802,
#46803,#46804,#46805,#46806,#46807,#46808,#46809,#46810,#46811,#46812,#46813,
#46814,#46815,#46816,#46817,#46818,#46819,#46820,#46821,#46822,#46823,#46824,
#46825,#46826,#46827,#46828,#46829,#46830,#46831,#46832,#46833,#46834,#46835,
#46836,#46837,#46838,#46839,#46840),(#46841,#46842,#46843,#46844,#46845,
#46846,#46847,#46848,#46849,#46850,#46851,#46852,#46853,#46854,#46855,#46856,
#46857,#46858,#46859,#46860,#46861,#46862,#46863,#46864,#46865,#46866,#46867,
#46868,#46869,#46870,#46871,#46872,#46873,#46874,#46875,#46876,#46877,#46878,
#46879,#46880,#46881,#46882,#46883,#46884,#46885,#46886,#46887,#46888,#46889,
#46890,#46891,#46892,#46893,#46894,#46895,#46896,#46897,#46898,#46899,#46900,
#46901,#46902,#46903,#46904,#46905,#46906,#46907,#46908,#46909,#46910,#46911,
#46912,#46913,#46914,#46915,#46916,#46917,#46918,#46919,#46920,#46921,#46922,
#46923,#46924,#46925,#46926,#46927,#46928,#46929,#46930,#46931,#46932,#46933,
#46934,#46935,#46936,#46937,#46938,#46939,#46940,#46941,#46942,#46943,#46944,
#46945,#46946,#46947,#46948,#46949,#46950,#46951,#46952,#46953,#46954,#46955,
#46956,#46957,#46958,#46959,#46960,#46961,#46962,#46963,#46964,#46965,#46966,
#46967,#46968,#46969,#46970,#46971,#46972,#46973,#46974,#46975,#46976,#46977,
#46978,#46979,#46980,#46981,#46982,#46983,#46984,#46985,#46986,#46987,#46988,
#46989,#46990,#46991,#46992,#46993,#46994,#46995,#46996,#46997,#46998,#46999,
#47000,#47001,#47002,#47003,#47004,#47005,#47006,#47007,#47008,#47009,#47010,
#47011,#47012,#47013,#47014,#47015,#47016,#47017,#47018,#47019,#47020,#47021,
#47022,#47023,#47024,#47025,#47026,#47027,#47028,#47029,#47030,#47031,#47032,
#47033,#47034,#47035,#47036,#47037,#47038,#47039,#47040,#47041,#47042,#47043,
#47044,#47045,#47046,#47047,#47048,#47049,#47050,#47051,#47052,#47053,#47054,
#47055,#47056,#47057,#47058,#47059,#47060,#47061,#47062,#47063,#47064,#47065,
#47066,#47067,#47068,#47069,#47070,#47071,#47072,#47073,#47074,#47075,#47076,
#47077,#47078,#47079,#47080,#47081,#47082,#47083,#47084,#47085,#47086,#47087,
#47088,#47089,#47090,#47091,#47092,#47093,#47094,#47095,#47096,#47097,#47098,
#47099,#47100,#47101,#47102,#47103,#47104,#47105,#47106,#47107,#47108,#47109,
#47110,#47111,#47112,#47113,#47114,#47115,#47116,#47117,#47118,#47119,#47120,
#47121,#47122,#47123,#47124,#47125,#47126,#47127,#47128,#47129,#47130,#47131,
#47132,#47133,#47134,#47135,#47136,#47137,#47138,#47139,#47140,#47141,#47142,
#47143,#47144,#47145,#47146,#47147,#47148,#47149,#47150,#47151,#47152,#47153,
#47154,#47155,#47156,#47157,#47158,#47159,#47160,#47161,#47162,#47163,#47164,
#47165,#47166,#47167,#47168,#47169,#47170,#47171,#47172,#47173,#47174,#47175,
#47176,#47177,#47178,#47179,#47180,#47181,#47182,#47183,#47184,#47185,#47186,
#47187,#47188,#47189,#47190,#47191,#47192,#47193,#47194,#47195,#47196,#47197,
#47198,#47199,#47200,#47201,#47202,#47203,#47204,#47205,#47206,#47207,#47208,
#47209,#47210,#47211,#47212,#47213),(#47214,#47215,#47216,#47217,#47218,
#47219,#47220,#47221,#47222,#47223,#47224,#47225,#47226,#47227,#47228,#47229,
#47230,#47231,#47232,#47233,#47234,#47235,#47236,#47237,#47238,#47239,#47240,
#47241,#47242,#47243,#47244,#47245,#47246,#47247,#47248,#47249,#47250,#47251,
#47252,#47253,#47254,#47255,#47256,#47257,#47258,#47259,#47260,#47261,#47262,
#47263,#47264,#47265,#47266,#47267,#47268,#47269,#47270,#47271,#47272,#47273,
#47274,#47275,#47276,#47277,#47278,#47279,#47280,#47281,#47282,#47283,#47284,
#47285,#47286,#47287,#47288,#47289,#47290,#47291,#47292,#47293,#47294,#47295,
#47296,#47297,#47298,#47299,#47300,#47301,#47302,#47303,#47304,#47305,#47306,
#47307,#47308,#47309,#47310,#47311,#47312,#47313,#47314,#47315,#47316,#47317,
#47318,#47319,#47320,#47321,#47322,#47323,#47324,#47325,#47326,#47327,#47328,
#47329,#47330,#47331,#47332,#47333,#47334,#47335,#47336,#47337,#47338,#47339,
#47340,#47341,#47342,#47343,#47344,#47345,#47346,#47347,#47348,#47349,#47350,
#47351,#47352,#47353,#47354,#47355,#47356,#47357,#47358,#47359,#47360,#47361,
#47362,#47363,#47364,#47365,#47366,#47367,#47368,#47369,#47370,#47371,#47372,
#47373,#47374,#47375,#47376,#47377,#47378,#47379,#47380,#47381,#47382,#47383,
#47384,#47385,#47386,#47387,#47388,#47389,#47390,#47391,#47392,#47393,#47394,
#47395,#47396,#47397,#47398,#47399,#47400,#47401,#47402,#47403,#47404,#47405,
#47406,#47407,#47408,#47409,#47410,#47411,#47412,#47413,#47414,#47415,#47416,
#47417,#47418,#47419,#47420,#47421,#47422,#47423,#47424,#47425,#47426,#47427,
#47428,#47429,#47430,#47431,#47432,#47433,#47434,#47435,#47436,#47437,#47438,
#47439,#47440,#47441,#47442,#47443,#47444,#47445,#47446,#47447,#47448,#47449,
#47450,#47451,#47452,#47453,#47454,#47455,#47456,#47457,#47458,#47459,#47460,
#47461,#47462,#47463,#47464,#47465,#47466,#47467,#47468,#47469,#47470,#47471,
#47472,#47473,#47474,#47475,#47476,#47477,#47478,#47479,#47480,#47481,#47482,
#47483,#47484,#47485,#47486,#47487,#47488,#47489,#47490,#47491,#47492,#47493,
#47494,#47495,#47496,#47497,#47498,#47499,#47500,#47501,#47502,#47503,#47504,
#47505,#47506,#47507,#47508,#47509,#47510,#47511,#47512,#47513,#47514,#47515,
#47516,#47517,#47518,#47519,#47520,#47521,#47522,#47523,#47524,#47525,#47526,
#47527,#47528,#47529,#47530,#47531,#47532,#47533,#47534,#47535,#47536,#47537,
#47538,#47539,#47540,#47541,#47542,#47543,#47544,#47545,#47546,#47547,#47548,
#47549,#47550,#47551,#47552,#47553,#47554,#47555,#47556,#47557,#47558,#47559,
#47560,#47561,#47562,#47563,#47564,#47565,#47566,#47567,#47568,#47569,#47570,
#47571,#47572,#47573,#47574,#47575,#47576,#47577,#47578,#47579,#47580,#47581,
#47582,#47583,#47584,#47585,#47586)),.UNSPECIFIED.,.F.,.F.,.F.,(4,4),(4,
1,1,1,1,1,1,1,1,1,1,1,1,1,1,1,1,1,1,1,1,1,1,1,1,1,1,1,1,1,1,1,1,1,1,1,1,
1,1,1,1,1,1,1,1,1,1,1,1,1,1,1,1,1,1,1,1,1,1,1,1,1,1,1,1,1,1,1,1,1,1,1,1,
1,1,1,1,1,1,1,1,1,1,1,1,1,1,1,1,1,1,1,1,1,1,1,1,1,1,1,1,1,1,1,1,1,1,1,1,
1,1,1,1,1,1,1,1,1,1,1,1,1,1,1,1,1,1,1,1,1,1,1,1,1,1,1,1,1,1,1,1,1,1,1,1,
1,1,1,1,1,1,1,1,1,1,1,1,1,1,1,1,1,1,1,1,1,1,1,1,1,1,1,1,1,1,1,1,1,1,1,1,
1,1,1,1,1,1,1,1,1,1,1,1,1,1,1,1,1,1,1,1,1,1,1,1,1,1,1,1,1,1,1,1,1,1,1,1,
1,1,1,1,1,1,1,1,1,1,1,1,1,1,1,1,1,1,1,1,1,1,1,1,1,1,1,1,1,1,1,1,1,1,1,1,
1,1,1,1,1,1,1,1,1,1,1,1,1,1,1,1,1,1,1,1,1,1,1,1,1,1,1,1,1,1,1,1,1,1,1,1,
1,1,1,1,1,1,1,1,1,1,1,1,1,1,1,1,1,1,1,1,1,1,1,1,1,1,1,1,1,1,1,1,1,1,1,1,
1,1,1,1,1,1,1,1,1,1,1,1,1,1,1,1,1,1,1,1,1,1,1,1,1,1,1,1,1,1,1,1,1,1,1,1,
1,1,1,1,1,1,1,1,1,4),(0.,0.0329955678841869),(12.0719473386168,13.0706334181767,
14.0693194977367,15.0680055772966,16.0666916568566,17.0653777364165,18.0640638159765,
19.0627498955364,20.0614359750964,21.0601220546563,22.0588081342163,23.0574942137762,
24.0561802933362,25.0548663728961,26.0535524524561,27.052238532016,28.050924611576,
29.0496106911359,30.0482967706959,31.0469828502558,32.0456689298158,33.0443550093757,
34.0430410889357,35.0417271684956,36.0404132480556,37.0390993276155,38.0377854071755,
39.0364714867355,40.0351575662954,41.0338436458553,42.0325297254153,43.0312158049753,
44.0299018845352,45.0285879640952,46.0272740436551,47.0259601232151,48.024646202775,
49.023332282335,50.0220183618949,51.0207044414549,52.0193905210148,53.0180766005748,
54.0167626801347,55.0154487596947,56.0141348392546,57.0128209188146,58.0115069983745,
59.0101930779345,60.0088791574944,61.0075652370544,62.0062513166143,63.0049373961743,
64.0036234757342,65.0023095552942,66.0009956348541,66.9996817144141,67.998367793974,
68.997053873534,69.9957399530939,70.9944260326539,71.9931121122139,72.9917981917738,
73.9904842713337,74.9891703508937,75.9878564304536,76.9865425100136,77.9852285895736,
78.9839146691335,79.9826007486935,80.9812868282534,81.9799729078134,82.9786589873733,
83.9773450669333,84.9760311464932,85.9747172260532,86.9734033056131,87.9720893851731,
88.970775464733,89.969461544293,90.9681476238529,91.9668337034129,92.9655197829728,
93.9642058625328,94.9628919420927,95.9615780216527,96.9602641012126,97.9589501807726,
98.9576362603325,99.9563223398925,100.955008419452,101.953694499012,102.952380578572,
103.951066658132,104.949752737692,105.948438817252,106.947124896812,107.945810976372,
108.944497055932,109.943183135492,110.941869215052,111.940555294612,112.939241374172,
113.937927453732,114.936613533292,115.935299612852,116.933985692412,117.932671771972,
118.931357851532,119.930043931092,120.928730010651,121.927416090211,122.926102169771,
123.924788249331,124.923474328891,125.922160408451,126.920846488011,127.919532567571,
128.918218647131,129.916904726691,130.915590806251,131.914276885811,132.912962965371,
133.911649044931,134.910335124491,135.909021204051,136.907707283611,137.906393363171,
138.905079442731,139.903765522291,140.90245160185,141.90113768141,142.89982376097,
143.89850984053,144.89719592009,145.89588199965,146.89456807921,147.89325415877,
148.89194023833,149.89062631789,150.88931239745,151.88799847701,152.88668455657,
153.88537063613,154.88405671569,155.88274279525,156.88142887481,157.88011495437,
158.87880103393,159.87748711349,160.87617319305,161.874859272609,162.873545352169,
163.872231431729,164.870917511289,165.869603590849,166.868289670409,167.866975749969,
168.865661829529,169.864347909089,170.863033988649,171.861720068209,172.860406147769,
173.859092227329,174.857778306889,175.856464386449,176.855150466009,177.853836545569,
178.852522625129,179.851208704689,180.849894784249,181.848580863809,182.847266943368,
183.845953022928,184.844639102488,185.843325182048,186.842011261608,187.840697341168,
188.839383420728,189.838069500288,190.836755579848,191.835441659408,192.834127738968,
193.832813818528,194.831499898088,195.830185977648,196.828872057208,197.827558136768,
198.826244216328,199.824930295888,200.823616375448,201.822302455008,202.820988534567,
203.819674614127,204.818360693687,205.817046773247,206.815732852807,207.814418932367,
208.813105011927,209.811791091487,210.810477171047,211.809163250607,212.807849330167,
213.806535409727,214.805221489287,215.803907568847,216.802593648407,217.801279727967,
218.799965807527,219.798651887087,220.797337966647,221.796024046207,222.794710125767,
223.793396205326,224.792082284886,225.790768364446,226.789454444006,227.788140523566,
228.786826603126,229.785512682686,230.784198762246,231.782884841806,232.781570921366,
233.780257000926,234.778943080486,235.777629160046,236.776315239606,237.775001319166,
238.773687398726,239.772373478286,240.771059557846,241.769745637406,242.768431716966,
243.767117796525,244.765803876085,245.764489955645,246.763176035205,247.761862114765,
248.760548194325,249.759234273885,250.757920353445,251.756606433005,252.755292512565,
253.753978592125,254.752664671685,255.751350751245,256.750036830805,257.748722910365,
258.747408989925,259.746095069485,260.744781149045,261.743467228605,262.742153308165,
263.740839387725,264.739525467284,265.738211546844,266.736897626404,267.735583705964,
268.734269785524,269.732955865084,270.731641944644,271.730328024204,272.729014103764,
273.727700183324,274.726386262884,275.725072342444,276.723758422004,277.722444501564,
278.721130581124,279.719816660684,280.718502740244,281.717188819804,282.715874899364,
283.714560978924,284.713247058484,285.711933138043,286.710619217603,287.709305297163,
288.707991376723,289.706677456283,290.705363535843,291.704049615403,292.702735694963,
293.701421774523,294.700107854083,295.698793933643,296.697480013203,297.696166092763,
298.694852172323,299.693538251883,300.692224331443,301.690910411003,302.689596490563,
303.688282570123,304.686968649683,305.685654729243,306.684340808802,307.683026888362,
308.681712967922,309.680399047482,310.679085127042,311.677771206602,312.676457286162,
313.675143365722,314.673829445282,315.672515524842,316.671201604402,317.669887683962,
318.668573763522,319.667259843082,320.665945922642,321.664632002202,322.663318081762,
323.662004161322,324.660690240882,325.659376320442,326.658062400001,327.656748479561,
328.655434559121,329.654120638681,330.652806718241,331.651492797801,332.650178877361,
333.648864956921,334.647551036481,335.646237116041,336.644923195601,337.643609275161,
338.642295354721,339.640981434281,340.639667513841,341.638353593401,342.637039672961,
343.635725752521,344.634411832081,345.633097911641,346.631783991201,347.63047007076,
348.62915615032,349.62784222988,350.62652830944,351.625214389,352.62390046856,
353.62258654812,354.62127262768,355.61995870724,356.6186447868,357.61733086636,
358.61601694592,359.61470302548,360.61338910504,361.6120751846,362.61076126416,
363.60944734372,364.60813342328,365.60681950284,366.6055055824,367.60419166196,
368.602877741519,369.601563821079,370.600249900639,371.598935980199,372.597622059759,
373.596308139319,374.594994218879,375.593680298439,376.592366377999,377.591052457559,
378.589738537119,379.588424616679,380.587110696239,381.585796775799),
 .UNSPECIFIED.);
#370=B_SPLINE_SURFACE_WITH_KNOTS('',3,3,((#47724,#47725,#47726,#47727,#47728,
#47729,#47730,#47731,#47732,#47733,#47734,#47735,#47736,#47737,#47738,#47739,
#47740,#47741,#47742,#47743,#47744,#47745,#47746,#47747,#47748,#47749,#47750,
#47751,#47752,#47753,#47754,#47755,#47756,#47757,#47758,#47759,#47760,#47761,
#47762,#47763,#47764,#47765,#47766,#47767,#47768,#47769,#47770,#47771,#47772,
#47773,#47774,#47775,#47776,#47777,#47778,#47779,#47780,#47781,#47782,#47783,
#47784,#47785,#47786,#47787,#47788,#47789,#47790,#47791,#47792,#47793,#47794,
#47795,#47796,#47797,#47798,#47799,#47800,#47801,#47802,#47803,#47804,#47805,
#47806,#47807,#47808,#47809,#47810,#47811,#47812,#47813,#47814,#47815,#47816,
#47817,#47818,#47819,#47820,#47821,#47822,#47823,#47824,#47825,#47826,#47827,
#47828,#47829,#47830,#47831,#47832,#47833,#47834,#47835,#47836,#47837,#47838,
#47839,#47840,#47841,#47842,#47843,#47844,#47845,#47846,#47847,#47848,#47849,
#47850,#47851,#47852,#47853,#47854,#47855,#47856,#47857,#47858,#47859,#47860,
#47861,#47862,#47863,#47864,#47865,#47866,#47867,#47868,#47869,#47870,#47871,
#47872,#47873,#47874,#47875,#47876,#47877,#47878,#47879,#47880,#47881,#47882,
#47883,#47884,#47885,#47886,#47887,#47888,#47889,#47890,#47891,#47892,#47893,
#47894,#47895,#47896,#47897,#47898,#47899,#47900,#47901,#47902,#47903,#47904,
#47905,#47906,#47907,#47908,#47909,#47910,#47911,#47912,#47913,#47914,#47915,
#47916,#47917,#47918,#47919,#47920,#47921,#47922,#47923,#47924,#47925,#47926,
#47927,#47928,#47929,#47930,#47931,#47932,#47933,#47934,#47935,#47936,#47937,
#47938,#47939,#47940,#47941,#47942,#47943,#47944,#47945,#47946,#47947,#47948,
#47949,#47950,#47951,#47952,#47953,#47954,#47955,#47956,#47957,#47958,#47959,
#47960,#47961,#47962,#47963,#47964,#47965,#47966,#47967,#47968,#47969,#47970,
#47971,#47972,#47973,#47974,#47975,#47976,#47977,#47978,#47979,#47980,#47981,
#47982,#47983,#47984,#47985,#47986,#47987,#47988,#47989,#47990,#47991,#47992,
#47993,#47994,#47995,#47996,#47997,#47998,#47999,#48000,#48001,#48002,#48003,
#48004,#48005,#48006,#48007,#48008,#48009,#48010,#48011,#48012,#48013,#48014,
#48015,#48016,#48017,#48018,#48019,#48020,#48021,#48022,#48023,#48024,#48025,
#48026,#48027,#48028,#48029,#48030,#48031,#48032,#48033,#48034,#48035,#48036,
#48037,#48038,#48039,#48040,#48041,#48042,#48043,#48044,#48045,#48046,#48047,
#48048,#48049,#48050,#48051,#48052,#48053,#48054,#48055,#48056,#48057,#48058,
#48059,#48060,#48061,#48062,#48063,#48064,#48065,#48066,#48067,#48068,#48069,
#48070,#48071,#48072,#48073,#48074,#48075,#48076,#48077,#48078,#48079,#48080,
#48081,#48082,#48083,#48084,#48085,#48086,#48087,#48088,#48089,#48090,#48091,
#48092,#48093,#48094,#48095,#48096),(#48097,#48098,#48099,#48100,#48101,
#48102,#48103,#48104,#48105,#48106,#48107,#48108,#48109,#48110,#48111,#48112,
#48113,#48114,#48115,#48116,#48117,#48118,#48119,#48120,#48121,#48122,#48123,
#48124,#48125,#48126,#48127,#48128,#48129,#48130,#48131,#48132,#48133,#48134,
#48135,#48136,#48137,#48138,#48139,#48140,#48141,#48142,#48143,#48144,#48145,
#48146,#48147,#48148,#48149,#48150,#48151,#48152,#48153,#48154,#48155,#48156,
#48157,#48158,#48159,#48160,#48161,#48162,#48163,#48164,#48165,#48166,#48167,
#48168,#48169,#48170,#48171,#48172,#48173,#48174,#48175,#48176,#48177,#48178,
#48179,#48180,#48181,#48182,#48183,#48184,#48185,#48186,#48187,#48188,#48189,
#48190,#48191,#48192,#48193,#48194,#48195,#48196,#48197,#48198,#48199,#48200,
#48201,#48202,#48203,#48204,#48205,#48206,#48207,#48208,#48209,#48210,#48211,
#48212,#48213,#48214,#48215,#48216,#48217,#48218,#48219,#48220,#48221,#48222,
#48223,#48224,#48225,#48226,#48227,#48228,#48229,#48230,#48231,#48232,#48233,
#48234,#48235,#48236,#48237,#48238,#48239,#48240,#48241,#48242,#48243,#48244,
#48245,#48246,#48247,#48248,#48249,#48250,#48251,#48252,#48253,#48254,#48255,
#48256,#48257,#48258,#48259,#48260,#48261,#48262,#48263,#48264,#48265,#48266,
#48267,#48268,#48269,#48270,#48271,#48272,#48273,#48274,#48275,#48276,#48277,
#48278,#48279,#48280,#48281,#48282,#48283,#48284,#48285,#48286,#48287,#48288,
#48289,#48290,#48291,#48292,#48293,#48294,#48295,#48296,#48297,#48298,#48299,
#48300,#48301,#48302,#48303,#48304,#48305,#48306,#48307,#48308,#48309,#48310,
#48311,#48312,#48313,#48314,#48315,#48316,#48317,#48318,#48319,#48320,#48321,
#48322,#48323,#48324,#48325,#48326,#48327,#48328,#48329,#48330,#48331,#48332,
#48333,#48334,#48335,#48336,#48337,#48338,#48339,#48340,#48341,#48342,#48343,
#48344,#48345,#48346,#48347,#48348,#48349,#48350,#48351,#48352,#48353,#48354,
#48355,#48356,#48357,#48358,#48359,#48360,#48361,#48362,#48363,#48364,#48365,
#48366,#48367,#48368,#48369,#48370,#48371,#48372,#48373,#48374,#48375,#48376,
#48377,#48378,#48379,#48380,#48381,#48382,#48383,#48384,#48385,#48386,#48387,
#48388,#48389,#48390,#48391,#48392,#48393,#48394,#48395,#48396,#48397,#48398,
#48399,#48400,#48401,#48402,#48403,#48404,#48405,#48406,#48407,#48408,#48409,
#48410,#48411,#48412,#48413,#48414,#48415,#48416,#48417,#48418,#48419,#48420,
#48421,#48422,#48423,#48424,#48425,#48426,#48427,#48428,#48429,#48430,#48431,
#48432,#48433,#48434,#48435,#48436,#48437,#48438,#48439,#48440,#48441,#48442,
#48443,#48444,#48445,#48446,#48447,#48448,#48449,#48450,#48451,#48452,#48453,
#48454,#48455,#48456,#48457,#48458,#48459,#48460,#48461,#48462,#48463,#48464,
#48465,#48466,#48467,#48468,#48469),(#48470,#48471,#48472,#48473,#48474,
#48475,#48476,#48477,#48478,#48479,#48480,#48481,#48482,#48483,#48484,#48485,
#48486,#48487,#48488,#48489,#48490,#48491,#48492,#48493,#48494,#48495,#48496,
#48497,#48498,#48499,#48500,#48501,#48502,#48503,#48504,#48505,#48506,#48507,
#48508,#48509,#48510,#48511,#48512,#48513,#48514,#48515,#48516,#48517,#48518,
#48519,#48520,#48521,#48522,#48523,#48524,#48525,#48526,#48527,#48528,#48529,
#48530,#48531,#48532,#48533,#48534,#48535,#48536,#48537,#48538,#48539,#48540,
#48541,#48542,#48543,#48544,#48545,#48546,#48547,#48548,#48549,#48550,#48551,
#48552,#48553,#48554,#48555,#48556,#48557,#48558,#48559,#48560,#48561,#48562,
#48563,#48564,#48565,#48566,#48567,#48568,#48569,#48570,#48571,#48572,#48573,
#48574,#48575,#48576,#48577,#48578,#48579,#48580,#48581,#48582,#48583,#48584,
#48585,#48586,#48587,#48588,#48589,#48590,#48591,#48592,#48593,#48594,#48595,
#48596,#48597,#48598,#48599,#48600,#48601,#48602,#48603,#48604,#48605,#48606,
#48607,#48608,#48609,#48610,#48611,#48612,#48613,#48614,#48615,#48616,#48617,
#48618,#48619,#48620,#48621,#48622,#48623,#48624,#48625,#48626,#48627,#48628,
#48629,#48630,#48631,#48632,#48633,#48634,#48635,#48636,#48637,#48638,#48639,
#48640,#48641,#48642,#48643,#48644,#48645,#48646,#48647,#48648,#48649,#48650,
#48651,#48652,#48653,#48654,#48655,#48656,#48657,#48658,#48659,#48660,#48661,
#48662,#48663,#48664,#48665,#48666,#48667,#48668,#48669,#48670,#48671,#48672,
#48673,#48674,#48675,#48676,#48677,#48678,#48679,#48680,#48681,#48682,#48683,
#48684,#48685,#48686,#48687,#48688,#48689,#48690,#48691,#48692,#48693,#48694,
#48695,#48696,#48697,#48698,#48699,#48700,#48701,#48702,#48703,#48704,#48705,
#48706,#48707,#48708,#48709,#48710,#48711,#48712,#48713,#48714,#48715,#48716,
#48717,#48718,#48719,#48720,#48721,#48722,#48723,#48724,#48725,#48726,#48727,
#48728,#48729,#48730,#48731,#48732,#48733,#48734,#48735,#48736,#48737,#48738,
#48739,#48740,#48741,#48742,#48743,#48744,#48745,#48746,#48747,#48748,#48749,
#48750,#48751,#48752,#48753,#48754,#48755,#48756,#48757,#48758,#48759,#48760,
#48761,#48762,#48763,#48764,#48765,#48766,#48767,#48768,#48769,#48770,#48771,
#48772,#48773,#48774,#48775,#48776,#48777,#48778,#48779,#48780,#48781,#48782,
#48783,#48784,#48785,#48786,#48787,#48788,#48789,#48790,#48791,#48792,#48793,
#48794,#48795,#48796,#48797,#48798,#48799,#48800,#48801,#48802,#48803,#48804,
#48805,#48806,#48807,#48808,#48809,#48810,#48811,#48812,#48813,#48814,#48815,
#48816,#48817,#48818,#48819,#48820,#48821,#48822,#48823,#48824,#48825,#48826,
#48827,#48828,#48829,#48830,#48831,#48832,#48833,#48834,#48835,#48836,#48837,
#48838,#48839,#48840,#48841,#48842),(#48843,#48844,#48845,#48846,#48847,
#48848,#48849,#48850,#48851,#48852,#48853,#48854,#48855,#48856,#48857,#48858,
#48859,#48860,#48861,#48862,#48863,#48864,#48865,#48866,#48867,#48868,#48869,
#48870,#48871,#48872,#48873,#48874,#48875,#48876,#48877,#48878,#48879,#48880,
#48881,#48882,#48883,#48884,#48885,#48886,#48887,#48888,#48889,#48890,#48891,
#48892,#48893,#48894,#48895,#48896,#48897,#48898,#48899,#48900,#48901,#48902,
#48903,#48904,#48905,#48906,#48907,#48908,#48909,#48910,#48911,#48912,#48913,
#48914,#48915,#48916,#48917,#48918,#48919,#48920,#48921,#48922,#48923,#48924,
#48925,#48926,#48927,#48928,#48929,#48930,#48931,#48932,#48933,#48934,#48935,
#48936,#48937,#48938,#48939,#48940,#48941,#48942,#48943,#48944,#48945,#48946,
#48947,#48948,#48949,#48950,#48951,#48952,#48953,#48954,#48955,#48956,#48957,
#48958,#48959,#48960,#48961,#48962,#48963,#48964,#48965,#48966,#48967,#48968,
#48969,#48970,#48971,#48972,#48973,#48974,#48975,#48976,#48977,#48978,#48979,
#48980,#48981,#48982,#48983,#48984,#48985,#48986,#48987,#48988,#48989,#48990,
#48991,#48992,#48993,#48994,#48995,#48996,#48997,#48998,#48999,#49000,#49001,
#49002,#49003,#49004,#49005,#49006,#49007,#49008,#49009,#49010,#49011,#49012,
#49013,#49014,#49015,#49016,#49017,#49018,#49019,#49020,#49021,#49022,#49023,
#49024,#49025,#49026,#49027,#49028,#49029,#49030,#49031,#49032,#49033,#49034,
#49035,#49036,#49037,#49038,#49039,#49040,#49041,#49042,#49043,#49044,#49045,
#49046,#49047,#49048,#49049,#49050,#49051,#49052,#49053,#49054,#49055,#49056,
#49057,#49058,#49059,#49060,#49061,#49062,#49063,#49064,#49065,#49066,#49067,
#49068,#49069,#49070,#49071,#49072,#49073,#49074,#49075,#49076,#49077,#49078,
#49079,#49080,#49081,#49082,#49083,#49084,#49085,#49086,#49087,#49088,#49089,
#49090,#49091,#49092,#49093,#49094,#49095,#49096,#49097,#49098,#49099,#49100,
#49101,#49102,#49103,#49104,#49105,#49106,#49107,#49108,#49109,#49110,#49111,
#49112,#49113,#49114,#49115,#49116,#49117,#49118,#49119,#49120,#49121,#49122,
#49123,#49124,#49125,#49126,#49127,#49128,#49129,#49130,#49131,#49132,#49133,
#49134,#49135,#49136,#49137,#49138,#49139,#49140,#49141,#49142,#49143,#49144,
#49145,#49146,#49147,#49148,#49149,#49150,#49151,#49152,#49153,#49154,#49155,
#49156,#49157,#49158,#49159,#49160,#49161,#49162,#49163,#49164,#49165,#49166,
#49167,#49168,#49169,#49170,#49171,#49172,#49173,#49174,#49175,#49176,#49177,
#49178,#49179,#49180,#49181,#49182,#49183,#49184,#49185,#49186,#49187,#49188,
#49189,#49190,#49191,#49192,#49193,#49194,#49195,#49196,#49197,#49198,#49199,
#49200,#49201,#49202,#49203,#49204,#49205,#49206,#49207,#49208,#49209,#49210,
#49211,#49212,#49213,#49214,#49215)),.UNSPECIFIED.,.F.,.F.,.F.,(4,4),(4,
1,1,1,1,1,1,1,1,1,1,1,1,1,1,1,1,1,1,1,1,1,1,1,1,1,1,1,1,1,1,1,1,1,1,1,1,
1,1,1,1,1,1,1,1,1,1,1,1,1,1,1,1,1,1,1,1,1,1,1,1,1,1,1,1,1,1,1,1,1,1,1,1,
1,1,1,1,1,1,1,1,1,1,1,1,1,1,1,1,1,1,1,1,1,1,1,1,1,1,1,1,1,1,1,1,1,1,1,1,
1,1,1,1,1,1,1,1,1,1,1,1,1,1,1,1,1,1,1,1,1,1,1,1,1,1,1,1,1,1,1,1,1,1,1,1,
1,1,1,1,1,1,1,1,1,1,1,1,1,1,1,1,1,1,1,1,1,1,1,1,1,1,1,1,1,1,1,1,1,1,1,1,
1,1,1,1,1,1,1,1,1,1,1,1,1,1,1,1,1,1,1,1,1,1,1,1,1,1,1,1,1,1,1,1,1,1,1,1,
1,1,1,1,1,1,1,1,1,1,1,1,1,1,1,1,1,1,1,1,1,1,1,1,1,1,1,1,1,1,1,1,1,1,1,1,
1,1,1,1,1,1,1,1,1,1,1,1,1,1,1,1,1,1,1,1,1,1,1,1,1,1,1,1,1,1,1,1,1,1,1,1,
1,1,1,1,1,1,1,1,1,1,1,1,1,1,1,1,1,1,1,1,1,1,1,1,1,1,1,1,1,1,1,1,1,1,1,1,
1,1,1,1,1,1,1,1,1,1,1,1,1,1,1,1,1,1,1,1,1,1,1,1,1,1,1,1,1,1,1,1,1,1,1,1,
1,1,1,1,1,1,1,1,1,4),(0.,0.0329955678841869),(15.385850931809,16.3845370113689,
17.3832230909289,18.3819091704888,19.3805952500488,20.3792813296087,21.3779674091687,
22.3766534887286,23.3753395682886,24.3740256478485,25.3727117274085,26.3713978069684,
27.3700838865284,28.3687699660883,29.3674560456483,30.3661421252082,31.3648282047682,
32.3635142843282,33.3622003638881,34.3608864434481,35.359572523008,36.358258602568,
37.3569446821279,38.3556307616879,39.3543168412478,40.3530029208078,41.3516890003677,
42.3503750799277,43.3490611594876,44.3477472390476,45.3464333186075,46.3451193981675,
47.3438054777274,48.3424915572874,49.3411776368473,50.3398637164073,51.3385497959672,
52.3372358755272,53.3359219550871,54.3346080346471,55.333294114207,56.331980193767,
57.3306662733269,58.3293523528869,59.3280384324468,60.3267245120068,61.3254105915667,
62.3240966711267,63.3227827506866,64.3214688302466,65.3201549098065,66.3188409893665,
67.3175270689264,68.3162131484864,69.3148992280463,70.3135853076063,71.3122713871662,
72.3109574667262,73.3096435462861,74.3083296258461,75.307015705406,76.305701784966,
77.3043878645259,78.3030739440859,79.3017600236459,80.3004461032058,81.2991321827658,
82.2978182623257,83.2965043418857,84.2951904214456,85.2938765010056,86.2925625805655,
87.2912486601255,88.2899347396854,89.2886208192454,90.2873068988053,91.2859929783653,
92.2846790579252,93.2833651374852,94.2820512170451,95.2807372966051,96.279423376165,
97.278109455725,98.2767955352849,99.2754816148449,100.274167694405,101.272853773965,
102.271539853525,103.270225933085,104.268912012645,105.267598092205,106.266284171765,
107.264970251324,108.263656330884,109.262342410444,110.261028490004,111.259714569564,
112.258400649124,113.257086728684,114.255772808244,115.254458887804,116.253144967364,
117.251831046924,118.250517126484,119.249203206044,120.247889285604,121.246575365164,
122.245261444724,123.243947524284,124.242633603844,125.241319683404,126.240005762964,
127.238691842524,128.237377922083,129.236064001643,130.234750081203,131.233436160763,
132.232122240323,133.230808319883,134.229494399443,135.228180479003,136.226866558563,
137.225552638123,138.224238717683,139.222924797243,140.221610876803,141.220296956363,
142.218983035923,143.217669115483,144.216355195043,145.215041274603,146.213727354163,
147.212413433723,148.211099513282,149.209785592842,150.208471672402,151.207157751962,
152.205843831522,153.204529911082,154.203215990642,155.201902070202,156.200588149762,
157.199274229322,158.197960308882,159.196646388442,160.195332468002,161.194018547562,
162.192704627122,163.191390706682,164.190076786242,165.188762865802,166.187448945362,
167.186135024922,168.184821104482,169.183507184041,170.182193263601,171.180879343161,
172.179565422721,173.178251502281,174.176937581841,175.175623661401,176.174309740961,
177.172995820521,178.171681900081,179.170367979641,180.169054059201,181.167740138761,
182.166426218321,183.165112297881,184.163798377441,185.162484457001,186.161170536561,
187.159856616121,188.158542695681,189.15722877524,190.1559148548,191.15460093436,
192.15328701392,193.15197309348,194.15065917304,195.1493452526,196.14803133216,
197.14671741172,198.14540349128,199.14408957084,200.1427756504,201.14146172996,
202.14014780952,203.13883388908,204.13751996864,205.1362060482,206.13489212776,
207.13357820732,208.13226428688,209.130950366439,210.129636445999,211.128322525559,
212.127008605119,213.125694684679,214.124380764239,215.123066843799,216.121752923359,
217.120439002919,218.119125082479,219.117811162039,220.116497241599,221.115183321159,
222.113869400719,223.112555480279,224.111241559839,225.109927639399,226.108613718959,
227.107299798519,228.105985878079,229.104671957639,230.103358037198,231.102044116758,
232.100730196318,233.099416275878,234.098102355438,235.096788434998,236.095474514558,
237.094160594118,238.092846673678,239.091532753238,240.090218832798,241.088904912358,
242.087590991918,243.086277071478,244.084963151038,245.083649230598,246.082335310158,
247.081021389718,248.079707469278,249.078393548838,250.077079628397,251.075765707957,
252.074451787517,253.073137867077,254.071823946637,255.070510026197,256.069196105757,
257.067882185317,258.066568264877,259.065254344437,260.063940423997,261.062626503557,
262.061312583117,263.059998662677,264.058684742237,265.057370821797,266.056056901357,
267.054742980917,268.053429060477,269.052115140037,270.050801219597,271.049487299156,
272.048173378716,273.046859458276,274.045545537836,275.044231617396,276.042917696956,
277.041603776516,278.040289856076,279.038975935636,280.037662015196,281.036348094756,
282.035034174316,283.033720253876,284.032406333436,285.031092412996,286.029778492556,
287.028464572116,288.027150651676,289.025836731236,290.024522810796,291.023208890355,
292.021894969915,293.020581049475,294.019267129035,295.017953208595,296.016639288155,
297.015325367715,298.014011447275,299.012697526835,300.011383606395,301.010069685955,
302.008755765515,303.007441845075,304.006127924635,305.004814004195,306.003500083755,
307.002186163315,308.000872242875,308.999558322435,309.998244401995,310.996930481555,
311.995616561114,312.994302640674,313.992988720234,314.991674799794,315.990360879354,
316.989046958914,317.987733038474,318.986419118034,319.985105197594,320.983791277154,
321.982477356714,322.981163436274,323.979849515834,324.978535595394,325.977221674954,
326.975907754514,327.974593834074,328.973279913634,329.971965993194,330.970652072754,
331.969338152313,332.968024231873,333.966710311433,334.965396390993,335.964082470553,
336.962768550113,337.961454629673,338.960140709233,339.958826788793,340.957512868353,
341.956198947913,342.954885027473,343.953571107033,344.952257186593,345.950943266153,
346.949629345713,347.948315425273,348.947001504833,349.945687584393,350.944373663953,
351.943059743512,352.941745823072,353.940431902632,354.939117982192,355.937804061752,
356.936490141312,357.935176220872,358.933862300432,359.932548379992,360.931234459552,
361.929920539112,362.928606618672,363.927292698232,364.925978777792,365.924664857352,
366.923350936912,367.922037016472,368.920723096032,369.919409175592,370.918095255152,
371.916781334712,372.915467414271,373.914153493831,374.912839573391,375.911525652951,
376.910211732511,377.908897812071,378.907583891631,379.906269971191,380.904956050751,
381.903642130311,382.902328209871,383.901014289431,384.899700368991),
 .UNSPECIFIED.);
#555=B_SPLINE_CURVE_WITH_KNOTS('',3,(#41667,#41668,#41669,#41670,#41671,
#41672,#41673,#41674,#41675,#41676,#41677,#41678,#41679,#41680,#41681,#41682),
 .UNSPECIFIED.,.F.,.F.,(4,3,3,3,3,4),(-6.60529764332032,-5.99211647735971,
-4.99343039779975,-3.9947443182398,-2.99605823867985,-2.07317267331967),
 .UNSPECIFIED.);
#556=B_SPLINE_CURVE_WITH_KNOTS('',3,(#41690,#41691,#41692,#41693,#41694,
#41695,#41696,#41697,#41698,#41699,#41700,#41701,#41702),.UNSPECIFIED.,
 .F.,.F.,(4,3,3,3,4),(0.,0.998686079559959,1.99737215911992,2.99605823867988,
3.63601592933386),.UNSPECIFIED.);
#557=B_SPLINE_CURVE_WITH_KNOTS('',3,(#41707,#41708,#41709,#41710,#41711,
#41712,#41713,#41714,#41715,#41716,#41717,#41718,#41719,#41720,#41721,#41722,
#41723,#41724,#41725,#41726,#41727,#41728),.UNSPECIFIED.,.F.,.F.,(4,3,3,
3,3,3,3,4),(-12.8884829504999,-11.9842329547194,-10.9855468751595,-9.98686079559951,
-8.98817471603956,-7.98948863647961,-6.99080255691966,-6.60529764332032),
 .UNSPECIFIED.);
#558=B_SPLINE_CURVE_WITH_KNOTS('',3,(#41729,#41730,#41731,#41732,#41733,
#41734,#41735,#41736,#41737,#41738,#41739,#41740,#41741,#41742,#41743,#41744,
#41745,#41746,#41747,#41748,#41749,#41750),.UNSPECIFIED.,.F.,.F.,(4,3,3,
3,3,3,3,4),(3.63601592933386,3.99474431823983,4.99343039779978,5.99211647735973,
6.99080255691967,7.98948863647962,8.98817471603956,9.91920123651348),
 .UNSPECIFIED.);
#559=B_SPLINE_CURVE_WITH_KNOTS('',3,(#41755,#41756,#41757,#41758,#41759,
#41760,#41761,#41762,#41763,#41764,#41765,#41766,#41767,#41768,#41769,#41770,
#41771,#41772,#41773,#41774,#41775,#41776,#41777,#41778,#41779),
 .UNSPECIFIED.,.F.,.F.,(4,3,3,3,3,3,3,3,4),(-19.1716682576795,-18.9750355116391,
-17.9763494320791,-16.9776633525192,-15.9789772729592,-14.9802911933993,
-13.9816051138393,-12.9829190342794,-12.8884829504999),.UNSPECIFIED.);
#560=B_SPLINE_CURVE_WITH_KNOTS('',3,(#41780,#41781,#41782,#41783,#41784,
#41785,#41786,#41787,#41788,#41789,#41790,#41791,#41792,#41793,#41794,#41795,
#41796,#41797,#41798,#41799,#41800,#41801,#41802,#41803,#41804),
 .UNSPECIFIED.,.F.,.F.,(4,3,3,3,3,3,3,3,4),(9.91920123651348,9.9868607955995,
10.9855468751595,11.9842329547194,12.9829190342794,13.9816051138393,14.9802911933993,
15.9789772729592,16.202386543693),.UNSPECIFIED.);
#561=B_SPLINE_CURVE_WITH_KNOTS('',3,(#41809,#41810,#41811,#41812,#41813,
#41814,#41815,#41816,#41817,#41818,#41819,#41820,#41821,#41822,#41823,#41824,
#41825,#41826,#41827,#41828,#41829,#41830),.UNSPECIFIED.,.F.,.F.,(4,3,3,
3,3,3,3,4),(-25.4548535648591,-24.9671519889988,-23.9684659094388,-22.9697798298789,
-21.9710937503189,-20.972407670759,-19.973721591199,-19.1716682576795),
 .UNSPECIFIED.);
#562=B_SPLINE_CURVE_WITH_KNOTS('',3,(#41831,#41832,#41833,#41834,#41835,
#41836,#41837,#41838,#41839,#41840,#41841,#41842,#41843,#41844,#41845,#41846,
#41847,#41848,#41849,#41850,#41851,#41852),.UNSPECIFIED.,.F.,.F.,(4,3,3,
3,3,3,3,4),(16.202386543693,16.9776633525192,17.9763494320791,18.9750355116391,
19.973721591199,20.972407670759,21.9710937503189,22.4855718508726),
 .UNSPECIFIED.);
#563=B_SPLINE_CURVE_WITH_KNOTS('',3,(#41857,#41858,#41859,#41860,#41861,
#41862,#41863,#41864,#41865,#41866,#41867,#41868,#41869,#41870,#41871,#41872,
#41873,#41874,#41875,#41876,#41877,#41878),.UNSPECIFIED.,.F.,.F.,(4,3,3,
3,3,3,3,4),(-31.7380388720387,-30.9592684663585,-29.9605823867985,-28.9618963072386,
-27.9632102276786,-26.9645241481187,-25.9658380685587,-25.4548535648591),
 .UNSPECIFIED.);
#564=B_SPLINE_CURVE_WITH_KNOTS('',3,(#41879,#41880,#41881,#41882,#41883,
#41884,#41885,#41886,#41887,#41888,#41889,#41890,#41891,#41892,#41893,#41894,
#41895,#41896,#41897,#41898,#41899,#41900),.UNSPECIFIED.,.F.,.F.,(4,3,3,
3,3,3,3,4),(22.4855718508726,22.9697798298789,23.9684659094388,24.9671519889988,
25.9658380685587,26.9645241481187,27.9632102276786,28.7687571580522),
 .UNSPECIFIED.);
#565=B_SPLINE_CURVE_WITH_KNOTS('',3,(#41905,#41906,#41907,#41908,#41909,
#41910,#41911,#41912,#41913,#41914,#41915,#41916,#41917,#41918,#41919,#41920,
#41921,#41922,#41923,#41924,#41925,#41926,#41927,#41928,#41929),
 .UNSPECIFIED.,.F.,.F.,(4,3,3,3,3,3,3,3,4),(-38.0212241792183,-37.9500710232781,
-36.9513849437182,-35.9526988641582,-34.9540127845983,-33.9553267050383,
-32.9566406254784,-31.9579545459184,-31.7380388720387),.UNSPECIFIED.);
#566=B_SPLINE_CURVE_WITH_KNOTS('',3,(#41930,#41931,#41932,#41933,#41934,
#41935,#41936,#41937,#41938,#41939,#41940,#41941,#41942,#41943,#41944,#41945,
#41946,#41947,#41948,#41949,#41950,#41951,#41952,#41953,#41954),
 .UNSPECIFIED.,.F.,.F.,(4,3,3,3,3,3,3,3,4),(28.7687571580522,28.9618963072386,
29.9605823867985,30.9592684663585,31.9579545459184,32.9566406254784,33.9553267050383,
34.9540127845983,35.0519424652318),.UNSPECIFIED.);
#567=B_SPLINE_CURVE_WITH_KNOTS('',3,(#41959,#41960,#41961,#41962,#41963,
#41964,#41965,#41966,#41967,#41968,#41969,#41970,#41971,#41972,#41973,#41974,
#41975,#41976,#41977,#41978,#41979,#41980),.UNSPECIFIED.,.F.,.F.,(4,3,3,
3,3,3,3,4),(-44.3044094863979,-43.9421875006378,-42.9435014210779,-41.9448153415179,
-40.946129261958,-39.947443182398,-38.9487571028381,-38.0212241792183),
 .UNSPECIFIED.);
#568=B_SPLINE_CURVE_WITH_KNOTS('',3,(#41981,#41982,#41983,#41984,#41985,
#41986,#41987,#41988,#41989,#41990,#41991,#41992,#41993,#41994,#41995,#41996,
#41997,#41998,#41999,#42000,#42001,#42002),.UNSPECIFIED.,.F.,.F.,(4,3,3,
3,3,3,3,4),(35.0519424652318,35.9526988641582,36.9513849437182,37.9500710232781,
38.9487571028381,39.947443182398,40.946129261958,41.3351277724114),
 .UNSPECIFIED.);
#569=B_SPLINE_CURVE_WITH_KNOTS('',3,(#42007,#42008,#42009,#42010,#42011,
#42012,#42013,#42014,#42015,#42016,#42017,#42018,#42019,#42020,#42021,#42022,
#42023,#42024,#42025,#42026,#42027,#42028),.UNSPECIFIED.,.F.,.F.,(4,3,3,
3,3,3,3,4),(-50.5875947935774,-49.9343039779976,-48.9356178984376,-47.9369318188777,
-46.9382457393177,-45.9395596597578,-44.9408735801978,-44.3044094863979),
 .UNSPECIFIED.);
#570=B_SPLINE_CURVE_WITH_KNOTS('',3,(#42029,#42030,#42031,#42032,#42033,
#42034,#42035,#42036,#42037,#42038,#42039,#42040,#42041,#42042,#42043,#42044,
#42045,#42046,#42047,#42048,#42049,#42050),.UNSPECIFIED.,.F.,.F.,(4,3,3,
3,3,3,3,4),(41.3351277724114,41.9448153415179,42.9435014210779,43.9421875006379,
44.9408735801978,45.9395596597578,46.9382457393177,47.618313079591),
 .UNSPECIFIED.);
#571=B_SPLINE_CURVE_WITH_KNOTS('',3,(#42055,#42056,#42057,#42058,#42059,
#42060,#42061,#42062,#42063,#42064,#42065,#42066,#42067,#42068,#42069,#42070,
#42071,#42072,#42073,#42074,#42075,#42076),.UNSPECIFIED.,.F.,.F.,(4,3,3,
3,3,3,3,4),(-56.8707801007571,-55.9264204553573,-54.9277343757973,-53.9290482962374,
-52.9303622166774,-51.9316761371175,-50.9329900575575,-50.5875947935774),
 .UNSPECIFIED.);
#572=B_SPLINE_CURVE_WITH_KNOTS('',3,(#42077,#42078,#42079,#42080,#42081,
#42082,#42083,#42084,#42085,#42086,#42087,#42088,#42089,#42090,#42091,#42092,
#42093,#42094,#42095,#42096,#42097,#42098),.UNSPECIFIED.,.F.,.F.,(4,3,3,
3,3,3,3,4),(47.618313079591,47.9369318188777,48.9356178984376,49.9343039779976,
50.9329900575575,51.9316761371175,52.9303622166774,53.9014983867706),
 .UNSPECIFIED.);
#573=B_SPLINE_CURVE_WITH_KNOTS('',3,(#42103,#42104,#42105,#42106,#42107,
#42108,#42109,#42110,#42111,#42112,#42113,#42114,#42115,#42116,#42117,#42118,
#42119,#42120,#42121,#42122,#42123,#42124,#42125,#42126,#42127),
 .UNSPECIFIED.,.F.,.F.,(4,3,3,3,3,3,3,3,4),(-63.1539654079367,-62.9172230122769,
-61.918536932717,-60.919850853157,-59.9211647735971,-58.9224786940371,-57.9237926144772,
-56.9251065349172,-56.8707801007571),.UNSPECIFIED.);
#574=B_SPLINE_CURVE_WITH_KNOTS('',3,(#42128,#42129,#42130,#42131,#42132,
#42133,#42134,#42135,#42136,#42137,#42138,#42139,#42140,#42141,#42142,#42143,
#42144,#42145,#42146,#42147,#42148,#42149,#42150,#42151,#42152),
 .UNSPECIFIED.,.F.,.F.,(4,3,3,3,3,3,3,3,4),(53.9014983867706,53.9290482962374,
54.9277343757973,55.9264204553573,56.9251065349172,57.9237926144772,58.9224786940371,
59.9211647735971,60.1846836939502),.UNSPECIFIED.);
#575=B_SPLINE_CURVE_WITH_KNOTS('',3,(#42157,#42158,#42159,#42160,#42161,
#42162,#42163,#42164,#42165,#42166,#42167,#42168,#42169,#42170,#42171,#42172,
#42173,#42174,#42175,#42176,#42177,#42178),.UNSPECIFIED.,.F.,.F.,(4,3,3,
3,3,3,3,4),(-69.4371507151162,-68.9093394896366,-67.9106534100767,-66.9119673305167,
-65.9132812509568,-64.9145951713968,-63.9159090918369,-63.1539654079367),
 .UNSPECIFIED.);
#576=B_SPLINE_CURVE_WITH_KNOTS('',3,(#42179,#42180,#42181,#42182,#42183,
#42184,#42185,#42186,#42187,#42188,#42189,#42190,#42191,#42192,#42193,#42194,
#42195,#42196,#42197,#42198,#42199,#42200),.UNSPECIFIED.,.F.,.F.,(4,3,3,
3,3,3,3,4),(60.1846836939502,60.919850853157,61.918536932717,62.9172230122769,
63.9159090918369,64.9145951713968,65.9132812509568,66.4678690011298),
 .UNSPECIFIED.);
#577=B_SPLINE_CURVE_WITH_KNOTS('',3,(#42205,#42206,#42207,#42208,#42209,
#42210,#42211,#42212,#42213,#42214,#42215,#42216,#42217,#42218,#42219,#42220,
#42221,#42222,#42223,#42224,#42225,#42226),.UNSPECIFIED.,.F.,.F.,(4,3,3,
3,3,3,3,4),(-75.7203360222958,-74.9014559669963,-73.9027698874364,-72.9040838078764,
-71.9053977283165,-70.9067116487565,-69.9080255691966,-69.4371507151162),
 .UNSPECIFIED.);
#578=B_SPLINE_CURVE_WITH_KNOTS('',3,(#42227,#42228,#42229,#42230,#42231,
#42232,#42233,#42234,#42235,#42236,#42237,#42238,#42239,#42240,#42241,#42242,
#42243,#42244,#42245,#42246,#42247,#42248),.UNSPECIFIED.,.F.,.F.,(4,3,3,
3,3,3,3,4),(66.4678690011298,66.9119673305167,67.9106534100767,68.9093394896366,
69.9080255691966,70.9067116487565,71.9053977283165,72.7510543083093),
 .UNSPECIFIED.);
#579=B_SPLINE_CURVE_WITH_KNOTS('',3,(#42253,#42254,#42255,#42256,#42257,
#42258,#42259,#42260,#42261,#42262,#42263,#42264,#42265,#42266,#42267,#42268,
#42269,#42270,#42271,#42272,#42273,#42274,#42275,#42276,#42277),
 .UNSPECIFIED.,.F.,.F.,(4,3,3,3,3,3,3,3,4),(-82.0035213294754,-81.892258523916,
-80.8935724443561,-79.8948863647961,-78.8962002852361,-77.8975142056762,
-76.8988281261162,-75.9001420465563,-75.7203360222958),.UNSPECIFIED.);
#580=B_SPLINE_CURVE_WITH_KNOTS('',3,(#42278,#42279,#42280,#42281,#42282,
#42283,#42284,#42285,#42286,#42287,#42288,#42289,#42290,#42291,#42292,#42293,
#42294,#42295,#42296,#42297,#42298,#42299,#42300,#42301,#42302),
 .UNSPECIFIED.,.F.,.F.,(4,3,3,3,3,3,3,3,4),(72.7510543083093,72.9040838078765,
73.9027698874364,74.9014559669964,75.9001420465563,76.8988281261163,77.8975142056762,
78.8962002852362,79.034239615489),.UNSPECIFIED.);
#581=B_SPLINE_CURVE_WITH_KNOTS('',3,(#42307,#42308,#42309,#42310,#42311,
#42312,#42313,#42314,#42315,#42316,#42317,#42318,#42319,#42320,#42321,#42322,
#42323,#42324,#42325,#42326,#42327,#42328),.UNSPECIFIED.,.F.,.F.,(4,3,3,
3,3,3,3,4),(-88.286706636655,-87.8843750012757,-86.8856889217157,-85.8870028421558,
-84.8883167625958,-83.8896306830359,-82.8909446034759,-82.0035213294754),
 .UNSPECIFIED.);
#582=B_SPLINE_CURVE_WITH_KNOTS('',3,(#42329,#42330,#42331,#42332,#42333,
#42334,#42335,#42336,#42337,#42338,#42339,#42340,#42341,#42342,#42343,#42344,
#42345,#42346,#42347,#42348,#42349,#42350),.UNSPECIFIED.,.F.,.F.,(4,3,3,
3,3,3,3,4),(79.034239615489,79.8948863647961,80.8935724443561,81.892258523916,
82.890944603476,83.8896306830359,84.8883167625959,85.3174249226685),
 .UNSPECIFIED.);
#583=B_SPLINE_CURVE_WITH_KNOTS('',3,(#42355,#42356,#42357,#42358,#42359,
#42360,#42361,#42362,#42363,#42364,#42365,#42366,#42367,#42368,#42369,#42370,
#42371,#42372,#42373,#42374,#42375,#42376),.UNSPECIFIED.,.F.,.F.,(4,3,3,
3,3,3,3,4),(-94.5698919438346,-93.8764914786354,-92.8778053990754,-91.8791193195155,
-90.8804332399556,-89.8817471603956,-88.8830610808356,-88.286706636655),
 .UNSPECIFIED.);
#584=B_SPLINE_CURVE_WITH_KNOTS('',3,(#42377,#42378,#42379,#42380,#42381,
#42382,#42383,#42384,#42385,#42386,#42387,#42388,#42389,#42390,#42391,#42392,
#42393,#42394,#42395,#42396,#42397,#42398),.UNSPECIFIED.,.F.,.F.,(4,3,3,
3,3,3,3,4),(85.3174249226685,85.8870028421558,86.8856889217158,87.8843750012757,
88.8830610808357,89.8817471603956,90.8804332399556,91.6006102298481),
 .UNSPECIFIED.);
#585=B_SPLINE_CURVE_WITH_KNOTS('',3,(#42403,#42404,#42405,#42406,#42407,
#42408,#42409,#42410,#42411,#42412,#42413,#42414,#42415,#42416,#42417,#42418,
#42419,#42420,#42421,#42422,#42423,#42424),.UNSPECIFIED.,.F.,.F.,(4,3,3,
3,3,3,3,4),(-100.853077251014,-99.8686079559951,-98.8699218764352,-97.8712357968752,
-96.8725497173153,-95.8738636377553,-94.8751775581954,-94.5698919438346),
 .UNSPECIFIED.);
#586=B_SPLINE_CURVE_WITH_KNOTS('',3,(#42425,#42426,#42427,#42428,#42429,
#42430,#42431,#42432,#42433,#42434,#42435,#42436,#42437,#42438,#42439,#42440,
#42441,#42442,#42443,#42444,#42445,#42446,#42447,#42448,#42449),
 .UNSPECIFIED.,.F.,.F.,(4,3,3,3,3,3,3,3,4),(91.6006102298481,91.8791193195155,
92.8778053990755,93.8764914786354,94.8751775581954,95.8738636377553,96.8725497173153,
97.8712357968752,97.8837955370278),.UNSPECIFIED.);
#587=B_SPLINE_CURVE_WITH_KNOTS('',3,(#42454,#42455,#42456,#42457,#42458,
#42459,#42460,#42461,#42462,#42463,#42464,#42465,#42466,#42467,#42468,#42469,
#42470,#42471,#42472,#42473,#42474,#42475,#42476,#42477,#42478),
 .UNSPECIFIED.,.F.,.F.,(4,3,3,3,3,3,3,3,4),(-107.136262558194,-106.859410512915,
-105.860724433355,-104.862038353795,-103.863352274235,-102.864666194675,
-101.865980115115,-100.867294035555,-100.853077251014),.UNSPECIFIED.);
#588=B_SPLINE_CURVE_WITH_KNOTS('',3,(#42479,#42480,#42481,#42482,#42483,
#42484,#42485,#42486,#42487,#42488,#42489,#42490,#42491,#42492,#42493,#42494,
#42495,#42496,#42497,#42498,#42499,#42500),.UNSPECIFIED.,.F.,.F.,(4,3,3,
3,3,3,3,4),(97.8837955370278,98.8699218764352,99.8686079559951,100.867294035555,
101.865980115115,102.864666194675,103.863352274235,104.166980844207),
 .UNSPECIFIED.);
#589=B_SPLINE_CURVE_WITH_KNOTS('',3,(#42505,#42506,#42507,#42508,#42509,
#42510,#42511,#42512,#42513,#42514,#42515,#42516,#42517,#42518,#42519,#42520,
#42521,#42522,#42523,#42524,#42525,#42526),.UNSPECIFIED.,.F.,.F.,(4,3,3,
3,3,3,3,4),(-113.419447865373,-112.851526990274,-111.852840910715,-110.854154831155,
-109.855468751595,-108.856782672035,-107.858096592475,-107.136262558194),
 .UNSPECIFIED.);
#590=B_SPLINE_CURVE_WITH_KNOTS('',3,(#42527,#42528,#42529,#42530,#42531,
#42532,#42533,#42534,#42535,#42536,#42537,#42538,#42539,#42540,#42541,#42542,
#42543,#42544,#42545,#42546,#42547,#42548),.UNSPECIFIED.,.F.,.F.,(4,3,3,
3,3,3,3,4),(104.166980844207,104.862038353795,105.860724433355,106.859410512915,
107.858096592475,108.856782672035,109.855468751595,110.450166151387),
 .UNSPECIFIED.);
#591=B_SPLINE_CURVE_WITH_KNOTS('',3,(#42553,#42554,#42555,#42556,#42557,
#42558,#42559,#42560,#42561,#42562,#42563,#42564,#42565,#42566,#42567,#42568,
#42569,#42570,#42571,#42572,#42573,#42574),.UNSPECIFIED.,.F.,.F.,(4,3,3,
3,3,3,3,4),(-119.702633172553,-118.843643467634,-117.844957388074,-116.846271308514,
-115.847585228954,-114.848899149394,-113.850213069834,-113.419447865373),
 .UNSPECIFIED.);
#592=B_SPLINE_CURVE_WITH_KNOTS('',3,(#42575,#42576,#42577,#42578,#42579,
#42580,#42581,#42582,#42583,#42584,#42585,#42586,#42587,#42588,#42589,#42590,
#42591,#42592,#42593,#42594,#42595,#42596),.UNSPECIFIED.,.F.,.F.,(4,3,3,
3,3,3,3,4),(110.450166151387,110.854154831155,111.852840910715,112.851526990275,
113.850213069834,114.848899149394,115.847585228954,116.733351458567),
 .UNSPECIFIED.);
#593=B_SPLINE_CURVE_WITH_KNOTS('',3,(#42601,#42602,#42603,#42604,#42605,
#42606,#42607,#42608,#42609,#42610,#42611,#42612,#42613,#42614,#42615,#42616,
#42617,#42618,#42619,#42620,#42621,#42622,#42623,#42624,#42625),
 .UNSPECIFIED.,.F.,.F.,(4,3,3,3,3,3,3,3,4),(-125.985818479733,-125.834446024554,
-124.835759944994,-123.837073865434,-122.838387785874,-121.839701706314,
-120.841015626754,-119.842329547194,-119.702633172553),.UNSPECIFIED.);
#594=B_SPLINE_CURVE_WITH_KNOTS('',3,(#42626,#42627,#42628,#42629,#42630,
#42631,#42632,#42633,#42634,#42635,#42636,#42637,#42638,#42639,#42640,#42641,
#42642,#42643,#42644,#42645,#42646,#42647,#42648,#42649,#42650),
 .UNSPECIFIED.,.F.,.F.,(4,3,3,3,3,3,3,3,4),(116.733351458567,116.846271308514,
117.844957388074,118.843643467634,119.842329547194,120.841015626754,121.839701706314,
122.838387785874,123.016536765746),.UNSPECIFIED.);
#595=B_SPLINE_CURVE_WITH_KNOTS('',3,(#42655,#42656,#42657,#42658,#42659,
#42660,#42661,#42662,#42663,#42664,#42665,#42666,#42667,#42668,#42669,#42670,
#42671,#42672,#42673,#42674,#42675,#42676),.UNSPECIFIED.,.F.,.F.,(4,3,3,
3,3,3,3,4),(-132.269003786912,-131.826562501914,-130.827876422354,-129.829190342794,
-128.830504263234,-127.831818183674,-126.833132104114,-125.985818479733),
 .UNSPECIFIED.);
#596=B_SPLINE_CURVE_WITH_KNOTS('',3,(#42677,#42678,#42679,#42680,#42681,
#42682,#42683,#42684,#42685,#42686,#42687,#42688,#42689,#42690,#42691,#42692,
#42693,#42694,#42695,#42696,#42697,#42698),.UNSPECIFIED.,.F.,.F.,(4,3,3,
3,3,3,3,4),(123.016536765746,123.837073865434,124.835759944994,125.834446024554,
126.833132104114,127.831818183674,128.830504263234,129.299722072926),
 .UNSPECIFIED.);
#597=B_SPLINE_CURVE_WITH_KNOTS('',3,(#42703,#42704,#42705,#42706,#42707,
#42708,#42709,#42710,#42711,#42712,#42713,#42714,#42715,#42716,#42717,#42718,
#42719,#42720,#42721,#42722,#42723,#42724),.UNSPECIFIED.,.F.,.F.,(4,3,3,
3,3,3,3,4),(-138.552189094092,-137.818678979273,-136.819992899713,-135.821306820153,
-134.822620740593,-133.823934661033,-132.825248581473,-132.269003786912),
 .UNSPECIFIED.);
#598=B_SPLINE_CURVE_WITH_KNOTS('',3,(#42725,#42726,#42727,#42728,#42729,
#42730,#42731,#42732,#42733,#42734,#42735,#42736,#42737,#42738,#42739,#42740,
#42741,#42742,#42743,#42744,#42745,#42746),.UNSPECIFIED.,.F.,.F.,(4,3,3,
3,3,3,3,4),(129.299722072926,129.829190342794,130.827876422354,131.826562501914,
132.825248581474,133.823934661033,134.822620740593,135.582907380105),
 .UNSPECIFIED.);
#599=B_SPLINE_CURVE_WITH_KNOTS('',3,(#42751,#42752,#42753,#42754,#42755,
#42756,#42757,#42758,#42759,#42760,#42761,#42762,#42763,#42764,#42765,#42766,
#42767,#42768,#42769,#42770,#42771,#42772,#42773,#42774,#42775),
 .UNSPECIFIED.,.F.,.F.,(4,3,3,3,3,3,3,3,4),(-144.835374401271,-144.809481536193,
-143.810795456633,-142.812109377073,-141.813423297513,-140.814737217953,
-139.816051138393,-138.817365058833,-138.552189094092),.UNSPECIFIED.);
#600=B_SPLINE_CURVE_WITH_KNOTS('',3,(#42776,#42777,#42778,#42779,#42780,
#42781,#42782,#42783,#42784,#42785,#42786,#42787,#42788,#42789,#42790,#42791,
#42792,#42793,#42794,#42795,#42796,#42797,#42798,#42799,#42800),
 .UNSPECIFIED.,.F.,.F.,(4,3,3,3,3,3,3,3,4),(135.582907380105,135.821306820153,
136.819992899713,137.818678979273,138.817365058833,139.816051138393,140.814737217953,
141.813423297513,141.866092687285),.UNSPECIFIED.);
#601=B_SPLINE_CURVE_WITH_KNOTS('',3,(#42805,#42806,#42807,#42808,#42809,
#42810,#42811,#42812,#42813,#42814,#42815,#42816,#42817,#42818,#42819,#42820,
#42821,#42822,#42823,#42824,#42825,#42826),.UNSPECIFIED.,.F.,.F.,(4,3,3,
3,3,3,3,4),(-151.118559708451,-150.801598013553,-149.802911933993,-148.804225854433,
-147.805539774873,-146.806853695313,-145.808167615753,-144.835374401271),
 .UNSPECIFIED.);
#602=B_SPLINE_CURVE_WITH_KNOTS('',3,(#42827,#42828,#42829,#42830,#42831,
#42832,#42833,#42834,#42835,#42836,#42837,#42838,#42839,#42840,#42841,#42842,
#42843,#42844,#42845,#42846,#42847,#42848),.UNSPECIFIED.,.F.,.F.,(4,3,3,
3,3,3,3,4),(141.866092687285,142.812109377073,143.810795456633,144.809481536193,
145.808167615753,146.806853695313,147.805539774873,148.149277994464),
 .UNSPECIFIED.);
#603=B_SPLINE_CURVE_WITH_KNOTS('',3,(#42853,#42854,#42855,#42856,#42857,
#42858,#42859,#42860,#42861,#42862,#42863,#42864,#42865,#42866,#42867,#42868,
#42869,#42870,#42871,#42872,#42873,#42874),.UNSPECIFIED.,.F.,.F.,(4,3,3,
3,3,3,3,4),(-157.40174501563,-156.793714490912,-155.795028411352,-154.796342331792,
-153.797656252232,-152.798970172673,-151.800284093113,-151.118559708451),
 .UNSPECIFIED.);
#604=B_SPLINE_CURVE_WITH_KNOTS('',3,(#42875,#42876,#42877,#42878,#42879,
#42880,#42881,#42882,#42883,#42884,#42885,#42886,#42887,#42888,#42889,#42890,
#42891,#42892,#42893,#42894,#42895,#42896),.UNSPECIFIED.,.F.,.F.,(4,3,3,
3,3,3,3,4),(148.149277994464,148.804225854433,149.802911933993,150.801598013553,
151.800284093113,152.798970172673,153.797656252233,154.432463301644),
 .UNSPECIFIED.);
#605=B_SPLINE_CURVE_WITH_KNOTS('',3,(#42901,#42902,#42903,#42904,#42905,
#42906,#42907,#42908,#42909,#42910,#42911,#42912,#42913,#42914,#42915,#42916,
#42917,#42918,#42919,#42920,#42921,#42922),.UNSPECIFIED.,.F.,.F.,(4,3,3,
3,3,3,3,4),(-163.68493032281,-162.785830968272,-161.787144888712,-160.788458809152,
-159.789772729592,-158.791086650032,-157.792400570472,-157.40174501563),
 .UNSPECIFIED.);
#606=B_SPLINE_CURVE_WITH_KNOTS('',3,(#42923,#42924,#42925,#42926,#42927,
#42928,#42929,#42930,#42931,#42932,#42933,#42934,#42935,#42936,#42937,#42938,
#42939,#42940,#42941,#42942,#42943,#42944),.UNSPECIFIED.,.F.,.F.,(4,3,3,
3,3,3,3,4),(154.432463301644,154.796342331793,155.795028411352,156.793714490912,
157.792400570472,158.791086650032,159.789772729592,160.715648608824),
 .UNSPECIFIED.);
#607=B_SPLINE_CURVE_WITH_KNOTS('',3,(#42949,#42950,#42951,#42952,#42953,
#42954,#42955,#42956,#42957,#42958,#42959,#42960,#42961,#42962,#42963,#42964,
#42965,#42966,#42967,#42968,#42969,#42970,#42971,#42972,#42973),
 .UNSPECIFIED.,.F.,.F.,(4,3,3,3,3,3,3,3,4),(-169.96811562999,-169.776633525192,
-168.777947445632,-167.779261366072,-166.780575286512,-165.781889206952,
-164.783203127392,-163.784517047832,-163.68493032281),.UNSPECIFIED.);
#608=B_SPLINE_CURVE_WITH_KNOTS('',3,(#42974,#42975,#42976,#42977,#42978,
#42979,#42980,#42981,#42982,#42983,#42984,#42985,#42986,#42987,#42988,#42989,
#42990,#42991,#42992,#42993,#42994,#42995,#42996,#42997,#42998),
 .UNSPECIFIED.,.F.,.F.,(4,3,3,3,3,3,3,3,4),(160.715648608824,160.788458809152,
161.787144888712,162.785830968272,163.784517047832,164.783203127392,165.781889206952,
166.780575286512,166.998833916003),.UNSPECIFIED.);
#609=B_SPLINE_CURVE_WITH_KNOTS('',3,(#43003,#43004,#43005,#43006,#43007,
#43008,#43009,#43010,#43011,#43012,#43013,#43014,#43015,#43016,#43017,#43018,
#43019,#43020,#43021,#43022,#43023,#43024),.UNSPECIFIED.,.F.,.F.,(4,3,3,
3,3,3,3,4),(-176.251300937169,-175.768750002551,-174.770063922991,-173.771377843432,
-172.772691763872,-171.774005684312,-170.775319604752,-169.96811562999),
 .UNSPECIFIED.);
#610=B_SPLINE_CURVE_WITH_KNOTS('',3,(#43025,#43026,#43027,#43028,#43029,
#43030,#43031,#43032,#43033,#43034,#43035,#43036,#43037,#43038,#43039,#43040,
#43041,#43042,#43043,#43044,#43045,#43046),.UNSPECIFIED.,.F.,.F.,(4,3,3,
3,3,3,3,4),(166.998833916003,167.779261366072,168.777947445632,169.776633525192,
170.775319604752,171.774005684312,172.772691763872,173.282019223183),
 .UNSPECIFIED.);
#611=B_SPLINE_CURVE_WITH_KNOTS('',3,(#43051,#43052,#43053,#43054,#43055,
#43056,#43057,#43058,#43059,#43060,#43061,#43062,#43063,#43064,#43065,#43066,
#43067,#43068,#43069,#43070,#43071,#43072),.UNSPECIFIED.,.F.,.F.,(4,3,3,
3,3,3,3,4),(-182.534486244349,-181.760866479911,-180.762180400351,-179.763494320791,
-178.764808241231,-177.766122161671,-176.767436082111,-176.251300937169),
 .UNSPECIFIED.);
#612=B_SPLINE_CURVE_WITH_KNOTS('',3,(#43073,#43074,#43075,#43076,#43077,
#43078,#43079,#43080,#43081,#43082,#43083,#43084,#43085,#43086,#43087,#43088,
#43089,#43090,#43091,#43092,#43093,#43094),.UNSPECIFIED.,.F.,.F.,(4,3,3,
3,3,3,3,4),(173.282019223183,173.771377843432,174.770063922992,175.768750002551,
176.767436082111,177.766122161671,178.764808241231,179.565204530362),
 .UNSPECIFIED.);
#613=B_SPLINE_CURVE_WITH_KNOTS('',3,(#43099,#43100,#43101,#43102,#43103,
#43104,#43105,#43106,#43107,#43108,#43109,#43110,#43111,#43112,#43113,#43114,
#43115,#43116,#43117,#43118,#43119,#43120,#43121,#43122,#43123),
 .UNSPECIFIED.,.F.,.F.,(4,3,3,3,3,3,3,3,4),(-188.817671551528,-188.751669036831,
-187.752982957271,-186.754296877711,-185.755610798151,-184.756924718591,
-183.758238639031,-182.759552559471,-182.534486244349),.UNSPECIFIED.);
#614=B_SPLINE_CURVE_WITH_KNOTS('',3,(#43124,#43125,#43126,#43127,#43128,
#43129,#43130,#43131,#43132,#43133,#43134,#43135,#43136,#43137,#43138,#43139,
#43140,#43141,#43142,#43143,#43144,#43145,#43146,#43147,#43148),
 .UNSPECIFIED.,.F.,.F.,(4,3,3,3,3,3,3,3,4),(179.565204530362,179.763494320791,
180.762180400351,181.760866479911,182.759552559471,183.758238639031,184.756924718591,
185.755610798151,185.848389837542),.UNSPECIFIED.);
#615=B_SPLINE_CURVE_WITH_KNOTS('',3,(#43153,#43154,#43155,#43156,#43157,
#43158,#43159,#43160,#43161,#43162,#43163,#43164,#43165,#43166,#43167,#43168,
#43169,#43170,#43171,#43172,#43173,#43174),.UNSPECIFIED.,.F.,.F.,(4,3,3,
3,3,3,3,4),(-195.100856858708,-194.74378551419,-193.745099434631,-192.746413355071,
-191.747727275511,-190.749041195951,-189.750355116391,-188.817671551528),
 .UNSPECIFIED.);
#616=B_SPLINE_CURVE_WITH_KNOTS('',3,(#43175,#43176,#43177,#43178,#43179,
#43180,#43181,#43182,#43183,#43184,#43185,#43186,#43187,#43188,#43189,#43190,
#43191,#43192,#43193,#43194,#43195,#43196),.UNSPECIFIED.,.F.,.F.,(4,3,3,
3,3,3,3,4),(185.848389837542,186.754296877711,187.752982957271,188.751669036831,
189.750355116391,190.749041195951,191.747727275511,192.131575144721),
 .UNSPECIFIED.);
#617=B_SPLINE_CURVE_WITH_KNOTS('',3,(#43201,#43202,#43203,#43204,#43205,
#43206,#43207,#43208,#43209,#43210,#43211,#43212,#43213,#43214,#43215,#43216,
#43217,#43218,#43219,#43220,#43221,#43222),.UNSPECIFIED.,.F.,.F.,(4,3,3,
3,3,3,3,4),(-201.384042165887,-200.73590199155,-199.73721591199,-198.73852983243,
-197.73984375287,-196.74115767331,-195.74247159375,-195.100856858708),
 .UNSPECIFIED.);
#618=B_SPLINE_CURVE_WITH_KNOTS('',3,(#43223,#43224,#43225,#43226,#43227,
#43228,#43229,#43230,#43231,#43232,#43233,#43234,#43235,#43236,#43237,#43238,
#43239,#43240,#43241,#43242,#43243,#43244),.UNSPECIFIED.,.F.,.F.,(4,3,3,
3,3,3,3,4),(192.131575144721,192.746413355071,193.745099434631,194.743785514191,
195.74247159375,196.74115767331,197.73984375287,198.414760451901),
 .UNSPECIFIED.);
#619=B_SPLINE_CURVE_WITH_KNOTS('',3,(#43249,#43250,#43251,#43252,#43253,
#43254,#43255,#43256,#43257,#43258,#43259,#43260,#43261,#43262,#43263,#43264,
#43265,#43266,#43267,#43268,#43269,#43270),.UNSPECIFIED.,.F.,.F.,(4,3,3,
3,3,3,3,4),(-207.667227473067,-206.72801846891,-205.72933238935,-204.73064630979,
-203.73196023023,-202.73327415067,-201.73458807111,-201.384042165887),
 .UNSPECIFIED.);
#620=B_SPLINE_CURVE_WITH_KNOTS('',3,(#43271,#43272,#43273,#43274,#43275,
#43276,#43277,#43278,#43279,#43280,#43281,#43282,#43283,#43284,#43285,#43286,
#43287,#43288,#43289,#43290,#43291,#43292),.UNSPECIFIED.,.F.,.F.,(4,3,3,
3,3,3,3,4),(198.414760451901,198.73852983243,199.73721591199,200.73590199155,
201.73458807111,202.73327415067,203.73196023023,204.69794575908),
 .UNSPECIFIED.);
#621=B_SPLINE_CURVE_WITH_KNOTS('',3,(#43297,#43298,#43299,#43300,#43301,
#43302,#43303,#43304,#43305,#43306,#43307,#43308,#43309,#43310,#43311,#43312,
#43313,#43314,#43315,#43316,#43317,#43318,#43319,#43320,#43321),
 .UNSPECIFIED.,.F.,.F.,(4,3,3,3,3,3,3,3,4),(-213.950412780246,-213.71882102583,
-212.72013494627,-211.72144886671,-210.72276278715,-209.72407670759,-208.72539062803,
-207.72670454847,-207.667227473067),.UNSPECIFIED.);
#622=B_SPLINE_CURVE_WITH_KNOTS('',3,(#43322,#43323,#43324,#43325,#43326,
#43327,#43328,#43329,#43330,#43331,#43332,#43333,#43334,#43335,#43336,#43337,
#43338,#43339,#43340,#43341,#43342,#43343,#43344,#43345,#43346),
 .UNSPECIFIED.,.F.,.F.,(4,3,3,3,3,3,3,3,4),(204.69794575908,204.73064630979,
205.72933238935,206.72801846891,207.72670454847,208.72539062803,209.72407670759,
210.72276278715,210.98113106626),.UNSPECIFIED.);
#623=B_SPLINE_CURVE_WITH_KNOTS('',3,(#43351,#43352,#43353,#43354,#43355,
#43356,#43357,#43358,#43359,#43360,#43361,#43362,#43363,#43364,#43365,#43366,
#43367,#43368,#43369,#43370,#43371,#43372),.UNSPECIFIED.,.F.,.F.,(4,3,3,
3,3,3,3,4),(-220.233598087426,-219.710937503189,-218.712251423629,-217.713565344069,
-216.714879264509,-215.716193184949,-214.717507105389,-213.950412780246),
 .UNSPECIFIED.);
#624=B_SPLINE_CURVE_WITH_KNOTS('',3,(#43373,#43374,#43375,#43376,#43377,
#43378,#43379,#43380,#43381,#43382,#43383,#43384,#43385,#43386,#43387,#43388,
#43389,#43390,#43391,#43392,#43393,#43394),.UNSPECIFIED.,.F.,.F.,(4,3,3,
3,3,3,3,4),(210.98113106626,211.72144886671,212.72013494627,213.71882102583,
214.71750710539,215.71619318495,216.714879264509,217.26431637344),
 .UNSPECIFIED.);
#625=B_SPLINE_CURVE_WITH_KNOTS('',3,(#43399,#43400,#43401,#43402,#43403,
#43404,#43405,#43406,#43407,#43408,#43409,#43410,#43411,#43412,#43413,#43414,
#43415,#43416,#43417,#43418,#43419,#43420),.UNSPECIFIED.,.F.,.F.,(4,3,3,
3,3,3,3,4),(-226.516783394606,-225.703053980549,-224.704367900989,-223.705681821429,
-222.706995741869,-221.708309662309,-220.709623582749,-220.233598087426),
 .UNSPECIFIED.);
#626=B_SPLINE_CURVE_WITH_KNOTS('',3,(#43421,#43422,#43423,#43424,#43425,
#43426,#43427,#43428,#43429,#43430,#43431,#43432,#43433,#43434,#43435,#43436,
#43437,#43438,#43439,#43440,#43441,#43442),.UNSPECIFIED.,.F.,.F.,(4,3,3,
3,3,3,3,4),(217.26431637344,217.713565344069,218.712251423629,219.710937503189,
220.709623582749,221.708309662309,222.706995741869,223.547501680619),
 .UNSPECIFIED.);
#627=B_SPLINE_CURVE_WITH_KNOTS('',3,(#43447,#43448,#43449,#43450,#43451,
#43452,#43453,#43454,#43455,#43456,#43457,#43458,#43459,#43460,#43461,#43462,
#43463,#43464,#43465,#43466,#43467,#43468,#43469,#43470,#43471),
 .UNSPECIFIED.,.F.,.F.,(4,3,3,3,3,3,3,3,4),(-232.799968701785,-232.693856537469,
-231.695170457909,-230.696484378349,-229.697798298789,-228.699112219229,
-227.700426139669,-226.701740060109,-226.516783394606),.UNSPECIFIED.);
#628=B_SPLINE_CURVE_WITH_KNOTS('',3,(#43472,#43473,#43474,#43475,#43476,
#43477,#43478,#43479,#43480,#43481,#43482,#43483,#43484,#43485,#43486,#43487,
#43488,#43489,#43490,#43491,#43492,#43493,#43494,#43495,#43496),
 .UNSPECIFIED.,.F.,.F.,(4,3,3,3,3,3,3,3,4),(223.547501680619,223.705681821429,
224.704367900989,225.703053980549,226.701740060109,227.700426139669,228.699112219229,
229.697798298789,229.830686987799),.UNSPECIFIED.);
#629=B_SPLINE_CURVE_WITH_KNOTS('',3,(#43501,#43502,#43503,#43504,#43505,
#43506,#43507,#43508,#43509,#43510,#43511,#43512,#43513,#43514,#43515,#43516,
#43517,#43518,#43519,#43520,#43521,#43522),.UNSPECIFIED.,.F.,.F.,(4,3,3,
3,3,3,3,4),(-239.083154008965,-238.685973014828,-237.687286935268,-236.688600855708,
-235.689914776148,-234.691228696589,-233.692542617029,-232.799968701785),
 .UNSPECIFIED.);
#630=B_SPLINE_CURVE_WITH_KNOTS('',3,(#43523,#43524,#43525,#43526,#43527,
#43528,#43529,#43530,#43531,#43532,#43533,#43534,#43535,#43536,#43537,#43538,
#43539,#43540,#43541,#43542,#43543,#43544),.UNSPECIFIED.,.F.,.F.,(4,3,3,
3,3,3,3,4),(229.830686987799,230.696484378349,231.695170457909,232.693856537469,
233.692542617029,234.691228696589,235.689914776149,236.113872294978),
 .UNSPECIFIED.);
#631=B_SPLINE_CURVE_WITH_KNOTS('',3,(#43549,#43550,#43551,#43552,#43553,
#43554,#43555,#43556,#43557,#43558,#43559,#43560,#43561,#43562,#43563,#43564,
#43565,#43566,#43567,#43568,#43569,#43570),.UNSPECIFIED.,.F.,.F.,(4,3,3,
3,3,3,3,4),(-245.366339316144,-244.678089492188,-243.679403412628,-242.680717333068,
-241.682031253508,-240.683345173948,-239.684659094388,-239.083154008965),
 .UNSPECIFIED.);
#632=B_SPLINE_CURVE_WITH_KNOTS('',3,(#43571,#43572,#43573,#43574,#43575,
#43576,#43577,#43578,#43579,#43580,#43581,#43582,#43583,#43584,#43585,#43586,
#43587,#43588,#43589,#43590,#43591,#43592),.UNSPECIFIED.,.F.,.F.,(4,3,3,
3,3,3,3,4),(236.113872294978,236.688600855709,237.687286935268,238.685973014828,
239.684659094388,240.683345173948,241.682031253508,242.397057602158),
 .UNSPECIFIED.);
#633=B_SPLINE_CURVE_WITH_KNOTS('',3,(#43597,#43598,#43599,#43600,#43601,
#43602,#43603,#43604,#43605,#43606,#43607,#43608,#43609,#43610,#43611,#43612,
#43613,#43614,#43615,#43616,#43617,#43618),.UNSPECIFIED.,.F.,.F.,(4,3,3,
3,3,3,3,4),(-251.649524623324,-250.670205969548,-249.671519889988,-248.672833810428,
-247.674147730868,-246.675461651308,-245.676775571748,-245.366339316144),
 .UNSPECIFIED.);
#634=B_SPLINE_CURVE_WITH_KNOTS('',3,(#43619,#43620,#43621,#43622,#43623,
#43624,#43625,#43626,#43627,#43628,#43629,#43630,#43631,#43632,#43633,#43634,
#43635,#43636,#43637,#43638,#43639,#43640,#43641,#43642,#43643),
 .UNSPECIFIED.,.F.,.F.,(4,3,3,3,3,3,3,3,4),(242.397057602158,242.680717333068,
243.679403412628,244.678089492188,245.676775571748,246.675461651308,247.674147730868,
248.672833810428,248.680242909337),.UNSPECIFIED.);
#635=B_SPLINE_CURVE_WITH_KNOTS('',3,(#43648,#43649,#43650,#43651,#43652,
#43653,#43654,#43655,#43656,#43657,#43658,#43659,#43660,#43661,#43662,#43663,
#43664,#43665,#43666,#43667,#43668,#43669,#43670,#43671,#43672),
 .UNSPECIFIED.,.F.,.F.,(4,3,3,3,3,3,3,3,4),(-257.932709930503,-257.661008526467,
-256.662322446907,-255.663636367347,-254.664950287788,-253.666264208228,
-252.667578128668,-251.668892049108,-251.649524623324),.UNSPECIFIED.);
#636=B_SPLINE_CURVE_WITH_KNOTS('',3,(#43673,#43674,#43675,#43676,#43677,
#43678,#43679,#43680,#43681,#43682,#43683,#43684,#43685,#43686,#43687,#43688,
#43689,#43690,#43691,#43692,#43693,#43694),.UNSPECIFIED.,.F.,.F.,(4,3,3,
3,3,3,3,4),(248.680242909337,249.671519889988,250.670205969548,251.668892049108,
252.667578128668,253.666264208228,254.664950287788,254.963428216517),
 .UNSPECIFIED.);
#637=B_SPLINE_CURVE_WITH_KNOTS('',3,(#43699,#43700,#43701,#43702,#43703,
#43704,#43705,#43706,#43707,#43708,#43709,#43710,#43711,#43712,#43713,#43714,
#43715,#43716,#43717,#43718,#43719,#43720),.UNSPECIFIED.,.F.,.F.,(4,3,3,
3,3,3,3,4),(-264.215895237683,-263.653125003827,-262.654438924267,-261.655752844707,
-260.657066765147,-259.658380685587,-258.659694606027,-257.932709930503),
 .UNSPECIFIED.);
#638=B_SPLINE_CURVE_WITH_KNOTS('',3,(#43721,#43722,#43723,#43724,#43725,
#43726,#43727,#43728,#43729,#43730,#43731,#43732,#43733,#43734,#43735,#43736,
#43737,#43738,#43739,#43740,#43741,#43742),.UNSPECIFIED.,.F.,.F.,(4,3,3,
3,3,3,3,4),(254.963428216517,255.663636367348,256.662322446908,257.661008526468,
258.659694606027,259.658380685587,260.657066765147,261.246613523697),
 .UNSPECIFIED.);
#639=B_SPLINE_CURVE_WITH_KNOTS('',3,(#43747,#43748,#43749,#43750,#43751,
#43752,#43753,#43754,#43755,#43756,#43757,#43758,#43759,#43760,#43761,#43762,
#43763,#43764,#43765,#43766,#43767,#43768),.UNSPECIFIED.,.F.,.F.,(4,3,3,
3,3,3,3,4),(-270.499080544863,-269.645241481187,-268.646555401627,-267.647869322067,
-266.649183242507,-265.650497162947,-264.651811083387,-264.215895237683),
 .UNSPECIFIED.);
#640=B_SPLINE_CURVE_WITH_KNOTS('',3,(#43769,#43770,#43771,#43772,#43773,
#43774,#43775,#43776,#43777,#43778,#43779,#43780,#43781,#43782,#43783,#43784,
#43785,#43786,#43787,#43788,#43789,#43790),.UNSPECIFIED.,.F.,.F.,(4,3,3,
3,3,3,3,4),(261.246613523697,261.655752844707,262.654438924267,263.653125003827,
264.651811083387,265.650497162947,266.649183242507,267.529798830876),
 .UNSPECIFIED.);
#641=B_SPLINE_CURVE_WITH_KNOTS('',3,(#43795,#43796,#43797,#43798,#43799,
#43800,#43801,#43802,#43803,#43804,#43805,#43806,#43807,#43808,#43809,#43810,
#43811,#43812,#43813,#43814,#43815,#43816,#43817,#43818,#43819),
 .UNSPECIFIED.,.F.,.F.,(4,3,3,3,3,3,3,3,4),(-276.782265852042,-276.636044038106,
-275.637357958546,-274.638671878987,-273.639985799427,-272.641299719867,
-271.642613640307,-270.643927560747,-270.499080544863),.UNSPECIFIED.);
#642=B_SPLINE_CURVE_WITH_KNOTS('',3,(#43820,#43821,#43822,#43823,#43824,
#43825,#43826,#43827,#43828,#43829,#43830,#43831,#43832,#43833,#43834,#43835,
#43836,#43837,#43838,#43839,#43840,#43841,#43842,#43843,#43844),
 .UNSPECIFIED.,.F.,.F.,(4,3,3,3,3,3,3,3,4),(267.529798830876,267.647869322067,
268.646555401627,269.645241481187,270.643927560747,271.642613640307,272.641299719867,
273.639985799427,273.812984138056),.UNSPECIFIED.);
#643=B_SPLINE_CURVE_WITH_KNOTS('',3,(#43849,#43850,#43851,#43852,#43853,
#43854,#43855,#43856,#43857,#43858,#43859,#43860,#43861,#43862,#43863,#43864,
#43865,#43866,#43867,#43868,#43869,#43870),.UNSPECIFIED.,.F.,.F.,(4,3,3,
3,3,3,3,4),(-283.065451159222,-282.628160515466,-281.629474435906,-280.630788356346,
-279.632102276786,-278.633416197226,-277.634730117666,-276.782265852042),
 .UNSPECIFIED.);
#644=B_SPLINE_CURVE_WITH_KNOTS('',3,(#43871,#43872,#43873,#43874,#43875,
#43876,#43877,#43878,#43879,#43880,#43881,#43882,#43883,#43884,#43885,#43886,
#43887,#43888,#43889,#43890,#43891,#43892),.UNSPECIFIED.,.F.,.F.,(4,3,3,
3,3,3,3,4),(273.812984138056,274.638671878987,275.637357958547,276.636044038107,
277.634730117666,278.633416197226,279.632102276786,280.096169445235),
 .UNSPECIFIED.);
#645=B_SPLINE_CURVE_WITH_KNOTS('',3,(#43897,#43898,#43899,#43900,#43901,
#43902,#43903,#43904,#43905,#43906,#43907,#43908,#43909,#43910,#43911,#43912,
#43913,#43914,#43915,#43916,#43917,#43918),.UNSPECIFIED.,.F.,.F.,(4,3,3,
3,3,3,3,4),(-289.348636466401,-288.620276992826,-287.621590913266,-286.622904833706,
-285.624218754146,-284.625532674586,-283.626846595026,-283.065451159222),
 .UNSPECIFIED.);
#646=B_SPLINE_CURVE_WITH_KNOTS('',3,(#43919,#43920,#43921,#43922,#43923,
#43924,#43925,#43926,#43927,#43928,#43929,#43930,#43931,#43932,#43933,#43934,
#43935,#43936,#43937,#43938,#43939,#43940),.UNSPECIFIED.,.F.,.F.,(4,3,3,
3,3,3,3,4),(280.096169445235,280.630788356346,281.629474435906,282.628160515466,
283.626846595026,284.625532674586,285.624218754146,286.379354752415),
 .UNSPECIFIED.);
#647=B_SPLINE_CURVE_WITH_KNOTS('',3,(#43945,#43946,#43947,#43948,#43949,
#43950,#43951,#43952,#43953,#43954,#43955,#43956,#43957,#43958,#43959,#43960,
#43961,#43962,#43963,#43964,#43965,#43966,#43967,#43968,#43969),
 .UNSPECIFIED.,.F.,.F.,(4,3,3,3,3,3,3,3,4),(-295.631821773581,-295.611079549746,
-294.612393470186,-293.613707390626,-292.615021311066,-291.616335231506,
-290.617649151946,-289.618963072386,-289.348636466401),.UNSPECIFIED.);
#648=B_SPLINE_CURVE_WITH_KNOTS('',3,(#43970,#43971,#43972,#43973,#43974,
#43975,#43976,#43977,#43978,#43979,#43980,#43981,#43982,#43983,#43984,#43985,
#43986,#43987,#43988,#43989,#43990,#43991,#43992,#43993,#43994),
 .UNSPECIFIED.,.F.,.F.,(4,3,3,3,3,3,3,3,4),(286.379354752415,286.622904833706,
287.621590913266,288.620276992826,289.618963072386,290.617649151946,291.616335231506,
292.615021311066,292.662540059594),.UNSPECIFIED.);
#649=B_SPLINE_CURVE_WITH_KNOTS('',3,(#43999,#44000,#44001,#44002,#44003,
#44004,#44005,#44006,#44007,#44008,#44009,#44010,#44011,#44012,#44013,#44014,
#44015,#44016,#44017,#44018,#44019,#44020),.UNSPECIFIED.,.F.,.F.,(4,3,3,
3,3,3,3,4),(-301.91500708076,-301.603196027105,-300.604509947545,-299.605823867985,
-298.607137788425,-297.608451708865,-296.609765629305,-295.631821773581),
 .UNSPECIFIED.);
#650=B_SPLINE_CURVE_WITH_KNOTS('',3,(#44021,#44022,#44023,#44024,#44025,
#44026,#44027,#44028,#44029,#44030,#44031,#44032,#44033,#44034,#44035,#44036,
#44037,#44038,#44039,#44040,#44041,#44042),.UNSPECIFIED.,.F.,.F.,(4,3,3,
3,3,3,3,4),(292.662540059594,293.613707390626,294.612393470186,295.611079549746,
296.609765629306,297.608451708865,298.607137788425,298.945725366774),
 .UNSPECIFIED.);
#651=B_SPLINE_CURVE_WITH_KNOTS('',3,(#44047,#44048,#44049,#44050,#44051,
#44052,#44053,#44054,#44055,#44056,#44057,#44058,#44059,#44060,#44061,#44062,
#44063,#44064,#44065,#44066,#44067,#44068),.UNSPECIFIED.,.F.,.F.,(4,3,3,
3,3,3,3,4),(-308.19819238794,-307.595312504465,-306.596626424905,-305.597940345345,
-304.599254265785,-303.600568186225,-302.601882106665,-301.91500708076),
 .UNSPECIFIED.);
#652=B_SPLINE_CURVE_WITH_KNOTS('',3,(#44069,#44070,#44071,#44072,#44073,
#44074,#44075,#44076,#44077,#44078,#44079,#44080,#44081,#44082,#44083,#44084,
#44085,#44086,#44087,#44088,#44089,#44090),.UNSPECIFIED.,.F.,.F.,(4,3,3,
3,3,3,3,4),(298.945725366774,299.605823867985,300.604509947545,301.603196027105,
302.601882106665,303.600568186225,304.599254265785,305.228910673953),
 .UNSPECIFIED.);
#653=B_SPLINE_CURVE_WITH_KNOTS('',3,(#44095,#44096,#44097,#44098,#44099,
#44100,#44101,#44102,#44103,#44104,#44105,#44106,#44107,#44108,#44109,#44110,
#44111,#44112,#44113,#44114,#44115,#44116),.UNSPECIFIED.,.F.,.F.,(4,3,3,
3,3,3,3,4),(-314.481377695119,-313.587428981825,-312.588742902265,-311.590056822705,
-310.591370743145,-309.592684663585,-308.593998584025,-308.19819238794),
 .UNSPECIFIED.);
#654=B_SPLINE_CURVE_WITH_KNOTS('',3,(#44117,#44118,#44119,#44120,#44121,
#44122,#44123,#44124,#44125,#44126,#44127,#44128,#44129,#44130,#44131,#44132,
#44133,#44134,#44135,#44136,#44137,#44138),.UNSPECIFIED.,.F.,.F.,(4,3,3,
3,3,3,3,4),(305.228910673953,305.597940345345,306.596626424905,307.595312504465,
308.593998584025,309.592684663585,310.591370743145,311.512095981133),
 .UNSPECIFIED.);
#655=B_SPLINE_CURVE_WITH_KNOTS('',3,(#44143,#44144,#44145,#44146,#44147,
#44148,#44149,#44150,#44151,#44152,#44153,#44154,#44155,#44156,#44157,#44158,
#44159,#44160,#44161,#44162,#44163,#44164,#44165,#44166,#44167),
 .UNSPECIFIED.,.F.,.F.,(4,3,3,3,3,3,3,3,4),(-320.764563002299,-320.578231538744,
-319.579545459184,-318.580859379624,-317.582173300064,-316.583487220505,
-315.584801140945,-314.586115061385,-314.481377695119),.UNSPECIFIED.);
#656=B_SPLINE_CURVE_WITH_KNOTS('',3,(#44168,#44169,#44170,#44171,#44172,
#44173,#44174,#44175,#44176,#44177,#44178,#44179,#44180,#44181,#44182,#44183,
#44184,#44185,#44186,#44187,#44188,#44189,#44190,#44191,#44192),
 .UNSPECIFIED.,.F.,.F.,(4,3,3,3,3,3,3,3,4),(311.512095981133,311.590056822705,
312.588742902265,313.587428981825,314.586115061385,315.584801140945,316.583487220505,
317.582173300065,317.795281288313),.UNSPECIFIED.);
#657=B_SPLINE_CURVE_WITH_KNOTS('',3,(#44197,#44198,#44199,#44200,#44201,
#44202,#44203,#44204,#44205,#44206,#44207,#44208,#44209,#44210,#44211,#44212,
#44213,#44214,#44215,#44216,#44217,#44218),.UNSPECIFIED.,.F.,.F.,(4,3,3,
3,3,3,3,4),(-327.047748309479,-326.570348016104,-325.571661936544,-324.572975856984,
-323.574289777424,-322.575603697864,-321.576917618304,-320.764563002299),
 .UNSPECIFIED.);
#658=B_SPLINE_CURVE_WITH_KNOTS('',3,(#44219,#44220,#44221,#44222,#44223,
#44224,#44225,#44226,#44227,#44228,#44229,#44230,#44231,#44232,#44233,#44234,
#44235,#44236,#44237,#44238,#44239,#44240),.UNSPECIFIED.,.F.,.F.,(4,3,3,
3,3,3,3,4),(317.795281288313,318.580859379625,319.579545459185,320.578231538744,
321.576917618304,322.575603697864,323.574289777424,324.078466595492),
 .UNSPECIFIED.);
#659=B_SPLINE_CURVE_WITH_KNOTS('',3,(#44245,#44246,#44247,#44248,#44249,
#44250,#44251,#44252,#44253,#44254,#44255,#44256,#44257,#44258,#44259,#44260,
#44261,#44262,#44263,#44264,#44265,#44266),.UNSPECIFIED.,.F.,.F.,(4,3,3,
3,3,3,3,4),(-333.330933616658,-332.562464493464,-331.563778413904,-330.565092334344,
-329.566406254784,-328.567720175224,-327.569034095664,-327.047748309479),
 .UNSPECIFIED.);
#660=B_SPLINE_CURVE_WITH_KNOTS('',3,(#44267,#44268,#44269,#44270,#44271,
#44272,#44273,#44274,#44275,#44276,#44277,#44278,#44279,#44280,#44281,#44282,
#44283,#44284,#44285,#44286,#44287,#44288),.UNSPECIFIED.,.F.,.F.,(4,3,3,
3,3,3,3,4),(324.078466595492,324.572975856984,325.571661936544,326.570348016104,
327.569034095664,328.567720175224,329.566406254784,330.361651902672),
 .UNSPECIFIED.);
#661=B_SPLINE_CURVE_WITH_KNOTS('',3,(#44293,#44294,#44295,#44296,#44297,
#44298,#44299,#44300,#44301,#44302,#44303,#44304,#44305,#44306,#44307,#44308,
#44309,#44310,#44311,#44312,#44313,#44314,#44315,#44316,#44317),
 .UNSPECIFIED.,.F.,.F.,(4,3,3,3,3,3,3,3,4),(-339.614118923838,-339.553267050383,
-338.554580970823,-337.555894891264,-336.557208811704,-335.558522732144,
-334.559836652584,-333.561150573024,-333.330933616658),.UNSPECIFIED.);
#662=B_SPLINE_CURVE_WITH_KNOTS('',3,(#44318,#44319,#44320,#44321,#44322,
#44323,#44324,#44325,#44326,#44327,#44328,#44329,#44330,#44331,#44332,#44333,
#44334,#44335,#44336,#44337,#44338,#44339,#44340,#44341,#44342),
 .UNSPECIFIED.,.F.,.F.,(4,3,3,3,3,3,3,3,4),(330.361651902672,330.565092334344,
331.563778413904,332.562464493464,333.561150573024,334.559836652584,335.558522732144,
336.557208811704,336.644837209851),.UNSPECIFIED.);
#663=B_SPLINE_CURVE_WITH_KNOTS('',3,(#44347,#44348,#44349,#44350,#44351,
#44352,#44353,#44354,#44355,#44356,#44357,#44358,#44359,#44360,#44361,#44362,
#44363,#44364,#44365,#44366,#44367,#44368),.UNSPECIFIED.,.F.,.F.,(4,3,3,
3,3,3,3,4),(-345.897304231017,-345.545383527743,-344.546697448183,-343.548011368623,
-342.549325289063,-341.550639209503,-340.551953129943,-339.614118923838),
 .UNSPECIFIED.);
#664=B_SPLINE_CURVE_WITH_KNOTS('',3,(#44369,#44370,#44371,#44372,#44373,
#44374,#44375,#44376,#44377,#44378,#44379,#44380,#44381,#44382,#44383,#44384,
#44385,#44386,#44387,#44388,#44389,#44390),.UNSPECIFIED.,.F.,.F.,(4,3,3,
3,3,3,3,4),(336.644837209851,337.555894891264,338.554580970824,339.553267050384,
340.551953129944,341.550639209503,342.549325289063,342.928022517031),
 .UNSPECIFIED.);
#665=B_SPLINE_CURVE_WITH_KNOTS('',3,(#44395,#44396,#44397,#44398,#44399,
#44400,#44401,#44402,#44403,#44404,#44405,#44406,#44407,#44408,#44409,#44410,
#44411,#44412,#44413,#44414,#44415,#44416),.UNSPECIFIED.,.F.,.F.,(4,3,3,
3,3,3,3,4),(-352.180489538197,-351.537500005103,-350.538813925543,-349.540127845983,
-348.541441766423,-347.542755686863,-346.544069607303,-345.897304231017),
 .UNSPECIFIED.);
#666=B_SPLINE_CURVE_WITH_KNOTS('',3,(#44417,#44418,#44419,#44420,#44421,
#44422,#44423,#44424,#44425,#44426,#44427,#44428,#44429,#44430,#44431,#44432,
#44433,#44434,#44435,#44436,#44437,#44438),.UNSPECIFIED.,.F.,.F.,(4,3,3,
3,3,3,3,4),(342.928022517031,343.548011368623,344.546697448183,345.545383527743,
346.544069607303,347.542755686863,348.541441766423,349.21120782421),
 .UNSPECIFIED.);
#667=B_SPLINE_CURVE_WITH_KNOTS('',3,(#44443,#44444,#44445,#44446,#44447,
#44448,#44449,#44450,#44451,#44452,#44453,#44454,#44455,#44456,#44457,#44458,
#44459,#44460,#44461,#44462,#44463,#44464),.UNSPECIFIED.,.F.,.F.,(4,3,3,
3,3,3,3,4),(-358.463674845376,-357.529616482463,-356.530930402903,-355.532244323343,
-354.533558243783,-353.534872164223,-352.536186084663,-352.180489538197),
 .UNSPECIFIED.);
#668=B_SPLINE_CURVE_WITH_KNOTS('',3,(#44465,#44466,#44467,#44468,#44469,
#44470,#44471,#44472,#44473,#44474,#44475,#44476,#44477,#44478,#44479,#44480,
#44481,#44482,#44483,#44484,#44485,#44486),.UNSPECIFIED.,.F.,.F.,(4,3,3,
3,3,3,3,4),(349.21120782421,349.540127845983,350.538813925543,351.537500005103,
352.536186084663,353.534872164223,354.533558243783,355.49439313139),
 .UNSPECIFIED.);
#669=B_SPLINE_CURVE_WITH_KNOTS('',3,(#44491,#44492,#44493,#44494,#44495,
#44496,#44497,#44498,#44499,#44500,#44501,#44502,#44503,#44504,#44505,#44506,
#44507,#44508,#44509,#44510,#44511,#44512,#44513,#44514,#44515),
 .UNSPECIFIED.,.F.,.F.,(4,3,3,3,3,3,3,3,4),(-364.746860152556,-364.520419039382,
-363.521732959822,-362.523046880262,-361.524360800702,-360.525674721142,
-359.526988641582,-358.528302562022,-358.463674845376),.UNSPECIFIED.);
#670=B_SPLINE_CURVE_WITH_KNOTS('',3,(#44516,#44517,#44518,#44519,#44520,
#44521,#44522,#44523,#44524,#44525,#44526,#44527,#44528,#44529,#44530,#44531,
#44532,#44533,#44534,#44535,#44536,#44537,#44538,#44539,#44540),
 .UNSPECIFIED.,.F.,.F.,(4,3,3,3,3,3,3,3,4),(355.49439313139,355.532244323343,
356.530930402903,357.529616482463,358.528302562023,359.526988641583,360.525674721143,
361.524360800702,361.77757843857),.UNSPECIFIED.);
#671=B_SPLINE_CURVE_WITH_KNOTS('',3,(#44546,#44547,#44548,#44549,#44550,
#44551),.UNSPECIFIED.,.F.,.F.,(4,1,1,4),(380.132711084365,380.904956050751,
381.903642130311,382.826527695671),.UNSPECIFIED.);
#672=B_SPLINE_CURVE_WITH_KNOTS('',3,(#44554,#44555,#44556,#44557,#44558),
 .UNSPECIFIED.,.F.,.F.,(4,1,4),(380.132711084365,380.587110696239,381.585796775799),
 .UNSPECIFIED.);
#673=B_SPLINE_CURVE_WITH_KNOTS('',3,(#44563,#44564,#44565,#44566,#44567,
#44568,#44569,#44570,#44571,#44572,#44573),.UNSPECIFIED.,.F.,.F.,(4,1,1,
1,1,1,1,1,4),(373.849525777185,373.914153493831,374.912839573391,375.911525652951,
376.910211732511,377.908897812071,378.907583891631,379.906269971191,380.132711084365),
 .UNSPECIFIED.);
#674=B_SPLINE_CURVE_WITH_KNOTS('',3,(#44574,#44575,#44576,#44577,#44578,
#44579,#44580,#44581,#44582,#44583),.UNSPECIFIED.,.F.,.F.,(4,1,1,1,1,1,
1,4),(373.849525777185,374.594994218879,375.593680298439,376.592366377999,
377.591052457559,378.589738537119,379.588424616679,380.132711084365),
 .UNSPECIFIED.);
#675=B_SPLINE_CURVE_WITH_KNOTS('',3,(#44588,#44589,#44590,#44591,#44592,
#44593,#44594,#44595,#44596,#44597),.UNSPECIFIED.,.F.,.F.,(4,1,1,1,1,1,
1,4),(367.566340470006,367.922037016472,368.920723096032,369.919409175592,
370.918095255152,371.916781334712,372.915467414271,373.849525777185),
 .UNSPECIFIED.);
#676=B_SPLINE_CURVE_WITH_KNOTS('',3,(#44598,#44599,#44600,#44601,#44602,
#44603,#44604,#44605,#44606,#44607,#44608),.UNSPECIFIED.,.F.,.F.,(4,1,1,
1,1,1,1,1,4),(367.566340470006,367.60419166196,368.602877741519,369.601563821079,
370.600249900639,371.598935980199,372.597622059759,373.596308139319,373.849525777185),
 .UNSPECIFIED.);
#677=B_SPLINE_CURVE_WITH_KNOTS('',3,(#44613,#44614,#44615,#44616,#44617,
#44618,#44619,#44620,#44621,#44622),.UNSPECIFIED.,.F.,.F.,(4,1,1,1,1,1,
1,4),(361.283155162826,361.929920539112,362.928606618672,363.927292698232,
364.925978777792,365.924664857352,366.923350936912,367.566340470006),
 .UNSPECIFIED.);
#678=B_SPLINE_CURVE_WITH_KNOTS('',3,(#44623,#44624,#44625,#44626,#44627,
#44628,#44629,#44630,#44631,#44632),.UNSPECIFIED.,.F.,.F.,(4,1,1,1,1,1,
1,4),(361.283155162826,361.6120751846,362.61076126416,363.60944734372,364.60813342328,
365.60681950284,366.6055055824,367.566340470006),.UNSPECIFIED.);
#679=B_SPLINE_CURVE_WITH_KNOTS('',3,(#44637,#44638,#44639,#44640,#44641,
#44642,#44643,#44644,#44645,#44646),.UNSPECIFIED.,.F.,.F.,(4,1,1,1,1,1,
1,4),(354.999969855647,355.937804061752,356.936490141312,357.935176220872,
358.933862300432,359.932548379992,360.931234459552,361.283155162826),
 .UNSPECIFIED.);
#680=B_SPLINE_CURVE_WITH_KNOTS('',3,(#44647,#44648,#44649,#44650,#44651,
#44652,#44653,#44654,#44655,#44656),.UNSPECIFIED.,.F.,.F.,(4,1,1,1,1,1,
1,4),(354.999969855647,355.61995870724,356.6186447868,357.61733086636,358.61601694592,
359.61470302548,360.61338910504,361.283155162826),.UNSPECIFIED.);
#681=B_SPLINE_CURVE_WITH_KNOTS('',3,(#44661,#44662,#44663,#44664,#44665,
#44666,#44667,#44668,#44669,#44670,#44671),.UNSPECIFIED.,.F.,.F.,(4,1,1,
1,1,1,1,1,4),(348.716784548467,348.947001504833,349.945687584393,350.944373663953,
351.943059743512,352.941745823072,353.940431902632,354.939117982192,354.999969855647),
 .UNSPECIFIED.);
#682=B_SPLINE_CURVE_WITH_KNOTS('',3,(#44672,#44673,#44674,#44675,#44676,
#44677,#44678,#44679,#44680,#44681),.UNSPECIFIED.,.F.,.F.,(4,1,1,1,1,1,
1,4),(348.716784548467,349.62784222988,350.62652830944,351.625214389,352.62390046856,
353.62258654812,354.62127262768,354.999969855647),.UNSPECIFIED.);
#683=B_SPLINE_CURVE_WITH_KNOTS('',3,(#44686,#44687,#44688,#44689,#44690,
#44691,#44692,#44693,#44694,#44695),.UNSPECIFIED.,.F.,.F.,(4,1,1,1,1,1,
1,4),(342.433599241287,342.954885027473,343.953571107033,344.952257186593,
345.950943266153,346.949629345713,347.948315425273,348.716784548467),
 .UNSPECIFIED.);
#684=B_SPLINE_CURVE_WITH_KNOTS('',3,(#44696,#44697,#44698,#44699,#44700,
#44701,#44702,#44703,#44704,#44705,#44706),.UNSPECIFIED.,.F.,.F.,(4,1,1,
1,1,1,1,1,4),(342.433599241288,342.637039672961,343.635725752521,344.634411832081,
345.633097911641,346.631783991201,347.63047007076,348.62915615032,348.716784548467),
 .UNSPECIFIED.);
#685=B_SPLINE_CURVE_WITH_KNOTS('',3,(#44711,#44712,#44713,#44714,#44715,
#44716,#44717,#44718,#44719,#44720),.UNSPECIFIED.,.F.,.F.,(4,1,1,1,1,1,
1,4),(336.150413934108,336.962768550113,337.961454629673,338.960140709233,
339.958826788793,340.957512868353,341.956198947913,342.433599241287),
 .UNSPECIFIED.);
#686=B_SPLINE_CURVE_WITH_KNOTS('',3,(#44721,#44722,#44723,#44724,#44725,
#44726,#44727,#44728,#44729,#44730),.UNSPECIFIED.,.F.,.F.,(4,1,1,1,1,1,
1,4),(336.150413934108,336.644923195601,337.643609275161,338.642295354721,
339.640981434281,340.639667513841,341.638353593401,342.433599241288),
 .UNSPECIFIED.);
#687=B_SPLINE_CURVE_WITH_KNOTS('',3,(#44735,#44736,#44737,#44738,#44739,
#44740,#44741,#44742,#44743,#44744,#44745),.UNSPECIFIED.,.F.,.F.,(4,1,1,
1,1,1,1,1,4),(329.867228626928,329.971965993194,330.970652072754,331.969338152313,
332.968024231873,333.966710311433,334.965396390993,335.964082470553,336.150413934108),
 .UNSPECIFIED.);
#688=B_SPLINE_CURVE_WITH_KNOTS('',3,(#44746,#44747,#44748,#44749,#44750,
#44751,#44752,#44753,#44754,#44755),.UNSPECIFIED.,.F.,.F.,(4,1,1,1,1,1,
1,4),(329.867228626928,330.652806718241,331.651492797801,332.650178877361,
333.648864956921,334.647551036481,335.646237116041,336.150413934108),
 .UNSPECIFIED.);
#689=B_SPLINE_CURVE_WITH_KNOTS('',3,(#44760,#44761,#44762,#44763,#44764,
#44765,#44766,#44767,#44768,#44769),.UNSPECIFIED.,.F.,.F.,(4,1,1,1,1,1,
1,4),(323.584043319749,323.979849515834,324.978535595394,325.977221674954,
326.975907754514,327.974593834074,328.973279913634,329.867228626928),
 .UNSPECIFIED.);
#690=B_SPLINE_CURVE_WITH_KNOTS('',3,(#44770,#44771,#44772,#44773,#44774,
#44775,#44776,#44777,#44778,#44779,#44780),.UNSPECIFIED.,.F.,.F.,(4,1,1,
1,1,1,1,1,4),(323.584043319749,323.662004161322,324.660690240882,325.659376320442,
326.658062400001,327.656748479561,328.655434559121,329.654120638681,329.867228626928),
 .UNSPECIFIED.);
#691=B_SPLINE_CURVE_WITH_KNOTS('',3,(#44785,#44786,#44787,#44788,#44789,
#44790,#44791,#44792,#44793,#44794),.UNSPECIFIED.,.F.,.F.,(4,1,1,1,1,1,
1,4),(317.300858012569,317.987733038474,318.986419118034,319.985105197594,
320.983791277154,321.982477356714,322.981163436274,323.584043319749),
 .UNSPECIFIED.);
#692=B_SPLINE_CURVE_WITH_KNOTS('',3,(#44795,#44796,#44797,#44798,#44799,
#44800,#44801,#44802,#44803,#44804),.UNSPECIFIED.,.F.,.F.,(4,1,1,1,1,1,
1,4),(317.300858012569,317.669887683962,318.668573763522,319.667259843082,
320.665945922642,321.664632002202,322.663318081762,323.584043319749),
 .UNSPECIFIED.);
#693=B_SPLINE_CURVE_WITH_KNOTS('',3,(#44809,#44810,#44811,#44812,#44813,
#44814,#44815,#44816,#44817,#44818),.UNSPECIFIED.,.F.,.F.,(4,1,1,1,1,1,
1,4),(311.01767270539,311.995616561114,312.994302640674,313.992988720234,
314.991674799794,315.990360879354,316.989046958914,317.300858012569),
 .UNSPECIFIED.);
#694=B_SPLINE_CURVE_WITH_KNOTS('',3,(#44819,#44820,#44821,#44822,#44823,
#44824,#44825,#44826,#44827,#44828),.UNSPECIFIED.,.F.,.F.,(4,1,1,1,1,1,
1,4),(311.01767270539,311.677771206602,312.676457286162,313.675143365722,
314.673829445282,315.672515524842,316.671201604402,317.300858012569),
 .UNSPECIFIED.);
#695=B_SPLINE_CURVE_WITH_KNOTS('',3,(#44833,#44834,#44835,#44836,#44837,
#44838,#44839,#44840,#44841,#44842,#44843),.UNSPECIFIED.,.F.,.F.,(4,1,1,
1,1,1,1,1,4),(304.73448739821,305.004814004195,306.003500083755,307.002186163315,
308.000872242875,308.999558322435,309.998244401995,310.996930481555,311.01767270539),
 .UNSPECIFIED.);
#696=B_SPLINE_CURVE_WITH_KNOTS('',3,(#44844,#44845,#44846,#44847,#44848,
#44849,#44850,#44851,#44852,#44853),.UNSPECIFIED.,.F.,.F.,(4,1,1,1,1,1,
1,4),(304.73448739821,305.685654729243,306.684340808802,307.683026888362,
308.681712967922,309.680399047482,310.679085127042,311.01767270539),
 .UNSPECIFIED.);
#697=B_SPLINE_CURVE_WITH_KNOTS('',3,(#44858,#44859,#44860,#44861,#44862,
#44863,#44864,#44865,#44866,#44867),.UNSPECIFIED.,.F.,.F.,(4,1,1,1,1,1,
1,4),(298.45130209103,299.012697526835,300.011383606395,301.010069685955,
302.008755765515,303.007441845075,304.006127924635,304.73448739821),
 .UNSPECIFIED.);
#698=B_SPLINE_CURVE_WITH_KNOTS('',3,(#44868,#44869,#44870,#44871,#44872,
#44873,#44874,#44875,#44876,#44877,#44878),.UNSPECIFIED.,.F.,.F.,(4,1,1,
1,1,1,1,1,4),(298.451302091031,298.694852172323,299.693538251883,300.692224331443,
301.690910411003,302.689596490563,303.688282570123,304.686968649683,304.73448739821),
 .UNSPECIFIED.);
#699=B_SPLINE_CURVE_WITH_KNOTS('',3,(#44883,#44884,#44885,#44886,#44887,
#44888,#44889,#44890,#44891,#44892),.UNSPECIFIED.,.F.,.F.,(4,1,1,1,1,1,
1,4),(292.168116783851,293.020581049475,294.019267129035,295.017953208595,
296.016639288155,297.015325367715,298.014011447275,298.45130209103),
 .UNSPECIFIED.);
#700=B_SPLINE_CURVE_WITH_KNOTS('',3,(#44893,#44894,#44895,#44896,#44897,
#44898,#44899,#44900,#44901,#44902),.UNSPECIFIED.,.F.,.F.,(4,1,1,1,1,1,
1,4),(292.168116783851,292.702735694963,293.701421774523,294.700107854083,
295.698793933643,296.697480013203,297.696166092763,298.451302091031),
 .UNSPECIFIED.);
#701=B_SPLINE_CURVE_WITH_KNOTS('',3,(#44907,#44908,#44909,#44910,#44911,
#44912,#44913,#44914,#44915,#44916,#44917),.UNSPECIFIED.,.F.,.F.,(4,1,1,
1,1,1,1,1,4),(285.884931476671,286.029778492556,287.028464572116,288.027150651676,
289.025836731236,290.024522810796,291.023208890355,292.021894969915,292.168116783851),
 .UNSPECIFIED.);
#702=B_SPLINE_CURVE_WITH_KNOTS('',3,(#44918,#44919,#44920,#44921,#44922,
#44923,#44924,#44925,#44926,#44927),.UNSPECIFIED.,.F.,.F.,(4,1,1,1,1,1,
1,4),(285.884931476671,286.710619217603,287.709305297163,288.707991376723,
289.706677456283,290.705363535843,291.704049615403,292.168116783851),
 .UNSPECIFIED.);
#703=B_SPLINE_CURVE_WITH_KNOTS('',3,(#44932,#44933,#44934,#44935,#44936,
#44937,#44938,#44939,#44940,#44941),.UNSPECIFIED.,.F.,.F.,(4,1,1,1,1,1,
1,4),(279.601746169492,280.037662015196,281.036348094756,282.035034174316,
283.033720253876,284.032406333436,285.031092412996,285.884931476671),
 .UNSPECIFIED.);
#704=B_SPLINE_CURVE_WITH_KNOTS('',3,(#44942,#44943,#44944,#44945,#44946,
#44947,#44948,#44949,#44950,#44951,#44952),.UNSPECIFIED.,.F.,.F.,(4,1,1,
1,1,1,1,1,4),(279.601746169492,279.719816660684,280.718502740244,281.717188819804,
282.715874899364,283.714560978924,284.713247058484,285.711933138043,285.884931476671),
 .UNSPECIFIED.);
#705=B_SPLINE_CURVE_WITH_KNOTS('',3,(#44957,#44958,#44959,#44960,#44961,
#44962,#44963,#44964,#44965,#44966),.UNSPECIFIED.,.F.,.F.,(4,1,1,1,1,1,
1,4),(273.318560862312,274.045545537836,275.044231617396,276.042917696956,
277.041603776516,278.040289856076,279.038975935636,279.601746169492),
 .UNSPECIFIED.);
#706=B_SPLINE_CURVE_WITH_KNOTS('',3,(#44967,#44968,#44969,#44970,#44971,
#44972,#44973,#44974,#44975,#44976),.UNSPECIFIED.,.F.,.F.,(4,1,1,1,1,1,
1,4),(273.318560862312,273.727700183324,274.726386262884,275.725072342444,
276.723758422004,277.722444501564,278.721130581124,279.601746169492),
 .UNSPECIFIED.);
#707=B_SPLINE_CURVE_WITH_KNOTS('',3,(#44981,#44982,#44983,#44984,#44985,
#44986,#44987,#44988,#44989,#44990,#44991),.UNSPECIFIED.,.F.,.F.,(4,1,1,
1,1,1,1,1,4),(267.035375555133,267.054742980917,268.053429060477,269.052115140037,
270.050801219597,271.049487299156,272.048173378716,273.046859458276,273.318560862312),
 .UNSPECIFIED.);
#708=B_SPLINE_CURVE_WITH_KNOTS('',3,(#44992,#44993,#44994,#44995,#44996,
#44997,#44998,#44999,#45000,#45001),.UNSPECIFIED.,.F.,.F.,(4,1,1,1,1,1,
1,4),(267.035375555133,267.735583705964,268.734269785524,269.732955865084,
270.731641944644,271.730328024204,272.729014103764,273.318560862312),
 .UNSPECIFIED.);
#709=B_SPLINE_CURVE_WITH_KNOTS('',3,(#45006,#45007,#45008,#45009,#45010,
#45011,#45012,#45013,#45014,#45015),.UNSPECIFIED.,.F.,.F.,(4,1,1,1,1,1,
1,4),(260.752190247953,261.062626503557,262.061312583117,263.059998662677,
264.058684742237,265.057370821797,266.056056901357,267.035375555133),
 .UNSPECIFIED.);
#710=B_SPLINE_CURVE_WITH_KNOTS('',3,(#45016,#45017,#45018,#45019,#45020,
#45021,#45022,#45023,#45024,#45025),.UNSPECIFIED.,.F.,.F.,(4,1,1,1,1,1,
1,4),(260.752190247953,261.743467228605,262.742153308165,263.740839387725,
264.739525467284,265.738211546844,266.736897626404,267.035375555133),
 .UNSPECIFIED.);
#711=B_SPLINE_CURVE_WITH_KNOTS('',3,(#45030,#45031,#45032,#45033,#45034,
#45035,#45036,#45037,#45038,#45039),.UNSPECIFIED.,.F.,.F.,(4,1,1,1,1,1,
1,4),(254.469004940773,255.070510026197,256.069196105757,257.067882185317,
258.066568264877,259.065254344437,260.063940423997,260.752190247953),
 .UNSPECIFIED.);
#712=B_SPLINE_CURVE_WITH_KNOTS('',3,(#45040,#45041,#45042,#45043,#45044,
#45045,#45046,#45047,#45048,#45049,#45050),.UNSPECIFIED.,.F.,.F.,(4,1,1,
1,1,1,1,1,4),(254.469004940774,254.752664671685,255.751350751245,256.750036830805,
257.748722910365,258.747408989925,259.746095069485,260.744781149045,260.752190247953),
 .UNSPECIFIED.);
#713=B_SPLINE_CURVE_WITH_KNOTS('',3,(#45055,#45056,#45057,#45058,#45059,
#45060,#45061,#45062,#45063,#45064),.UNSPECIFIED.,.F.,.F.,(4,1,1,1,1,1,
1,4),(248.185819633594,249.078393548838,250.077079628397,251.075765707957,
252.074451787517,253.073137867077,254.071823946637,254.469004940773),
 .UNSPECIFIED.);
#714=B_SPLINE_CURVE_WITH_KNOTS('',3,(#45065,#45066,#45067,#45068,#45069,
#45070,#45071,#45072,#45073,#45074),.UNSPECIFIED.,.F.,.F.,(4,1,1,1,1,1,
1,4),(248.185819633594,248.760548194325,249.759234273885,250.757920353445,
251.756606433005,252.755292512565,253.753978592125,254.469004940774),
 .UNSPECIFIED.);
#715=B_SPLINE_CURVE_WITH_KNOTS('',3,(#45079,#45080,#45081,#45082,#45083,
#45084,#45085,#45086,#45087,#45088,#45089),.UNSPECIFIED.,.F.,.F.,(4,1,1,
1,1,1,1,1,4),(241.902634326414,242.087590991918,243.086277071478,244.084963151038,
245.083649230598,246.082335310158,247.081021389718,248.079707469278,248.185819633594),
 .UNSPECIFIED.);
#716=B_SPLINE_CURVE_WITH_KNOTS('',3,(#45090,#45091,#45092,#45093,#45094,
#45095,#45096,#45097,#45098,#45099),.UNSPECIFIED.,.F.,.F.,(4,1,1,1,1,1,
1,4),(241.902634326415,242.768431716966,243.767117796525,244.765803876085,
245.764489955645,246.763176035205,247.761862114765,248.185819633594),
 .UNSPECIFIED.);
#717=B_SPLINE_CURVE_WITH_KNOTS('',3,(#45104,#45105,#45106,#45107,#45108,
#45109,#45110,#45111,#45112,#45113),.UNSPECIFIED.,.F.,.F.,(4,1,1,1,1,1,
1,4),(235.619449019235,236.095474514558,237.094160594118,238.092846673678,
239.091532753238,240.090218832798,241.088904912358,241.902634326414),
 .UNSPECIFIED.);
#718=B_SPLINE_CURVE_WITH_KNOTS('',3,(#45114,#45115,#45116,#45117,#45118,
#45119,#45120,#45121,#45122,#45123,#45124),.UNSPECIFIED.,.F.,.F.,(4,1,1,
1,1,1,1,1,4),(235.619449019235,235.777629160046,236.776315239606,237.775001319166,
238.773687398726,239.772373478286,240.771059557846,241.769745637406,241.902634326415),
 .UNSPECIFIED.);
#719=B_SPLINE_CURVE_WITH_KNOTS('',3,(#45129,#45130,#45131,#45132,#45133,
#45134,#45135,#45136,#45137,#45138),.UNSPECIFIED.,.F.,.F.,(4,1,1,1,1,1,
1,4),(229.336263712055,230.103358037198,231.102044116758,232.100730196318,
233.099416275878,234.098102355438,235.096788434998,235.619449019235),
 .UNSPECIFIED.);
#720=B_SPLINE_CURVE_WITH_KNOTS('',3,(#45139,#45140,#45141,#45142,#45143,
#45144,#45145,#45146,#45147,#45148),.UNSPECIFIED.,.F.,.F.,(4,1,1,1,1,1,
1,4),(229.336263712055,229.785512682686,230.784198762246,231.782884841806,
232.781570921366,233.780257000926,234.778943080486,235.619449019235),
 .UNSPECIFIED.);
#721=B_SPLINE_CURVE_WITH_KNOTS('',3,(#45153,#45154,#45155,#45156,#45157,
#45158,#45159,#45160,#45161,#45162,#45163),.UNSPECIFIED.,.F.,.F.,(4,1,1,
1,1,1,1,1,4),(223.053078404876,223.112555480279,224.111241559839,225.109927639399,
226.108613718959,227.107299798519,228.105985878079,229.104671957639,229.336263712055),
 .UNSPECIFIED.);
#722=B_SPLINE_CURVE_WITH_KNOTS('',3,(#45164,#45165,#45166,#45167,#45168,
#45169,#45170,#45171,#45172,#45173),.UNSPECIFIED.,.F.,.F.,(4,1,1,1,1,1,
1,4),(223.053078404876,223.793396205326,224.792082284886,225.790768364446,
226.789454444006,227.788140523566,228.786826603126,229.336263712055),
 .UNSPECIFIED.);
#723=B_SPLINE_CURVE_WITH_KNOTS('',3,(#45178,#45179,#45180,#45181,#45182,
#45183,#45184,#45185,#45186,#45187),.UNSPECIFIED.,.F.,.F.,(4,1,1,1,1,1,
1,4),(216.769893097696,217.120439002919,218.119125082479,219.117811162039,
220.116497241599,221.115183321159,222.113869400719,223.053078404876),
 .UNSPECIFIED.);
#724=B_SPLINE_CURVE_WITH_KNOTS('',3,(#45188,#45189,#45190,#45191,#45192,
#45193,#45194,#45195,#45196,#45197,#45198),.UNSPECIFIED.,.F.,.F.,(4,1,1,
1,1,1,1,1,4),(216.769893097696,216.802593648407,217.801279727967,218.799965807527,
219.798651887087,220.797337966647,221.796024046207,222.794710125767,223.053078404876),
 .UNSPECIFIED.);
#725=B_SPLINE_CURVE_WITH_KNOTS('',3,(#45203,#45204,#45205,#45206,#45207,
#45208,#45209,#45210,#45211,#45212),.UNSPECIFIED.,.F.,.F.,(4,1,1,1,1,1,
1,4),(210.486707790517,211.128322525559,212.127008605119,213.125694684679,
214.124380764239,215.123066843799,216.121752923359,216.769893097696),
 .UNSPECIFIED.);
#726=B_SPLINE_CURVE_WITH_KNOTS('',3,(#45213,#45214,#45215,#45216,#45217,
#45218,#45219,#45220,#45221,#45222),.UNSPECIFIED.,.F.,.F.,(4,1,1,1,1,1,
1,4),(210.486707790517,210.810477171047,211.809163250607,212.807849330167,
213.806535409727,214.805221489287,215.803907568847,216.769893097696),
 .UNSPECIFIED.);
#727=B_SPLINE_CURVE_WITH_KNOTS('',3,(#45227,#45228,#45229,#45230,#45231,
#45232,#45233,#45234,#45235,#45236),.UNSPECIFIED.,.F.,.F.,(4,1,1,1,1,1,
1,4),(204.203522483337,205.1362060482,206.13489212776,207.13357820732,208.13226428688,
209.130950366439,210.129636445999,210.486707790517),.UNSPECIFIED.);
#728=B_SPLINE_CURVE_WITH_KNOTS('',3,(#45237,#45238,#45239,#45240,#45241,
#45242,#45243,#45244,#45245,#45246),.UNSPECIFIED.,.F.,.F.,(4,1,1,1,1,1,
1,4),(204.203522483337,204.818360693687,205.817046773247,206.815732852807,
207.814418932367,208.813105011927,209.811791091487,210.486707790517),
 .UNSPECIFIED.);
#729=B_SPLINE_CURVE_WITH_KNOTS('',3,(#45251,#45252,#45253,#45254,#45255,
#45256,#45257,#45258,#45259,#45260,#45261),.UNSPECIFIED.,.F.,.F.,(4,1,1,
1,1,1,1,1,4),(197.920337176157,198.14540349128,199.14408957084,200.1427756504,
201.14146172996,202.14014780952,203.13883388908,204.13751996864,204.203522483337),
 .UNSPECIFIED.);
#730=B_SPLINE_CURVE_WITH_KNOTS('',3,(#45262,#45263,#45264,#45265,#45266,
#45267,#45268,#45269,#45270,#45271),.UNSPECIFIED.,.F.,.F.,(4,1,1,1,1,1,
1,4),(197.920337176158,198.826244216328,199.824930295888,200.823616375448,
201.822302455008,202.820988534567,203.819674614127,204.203522483337),
 .UNSPECIFIED.);
#731=B_SPLINE_CURVE_WITH_KNOTS('',3,(#45276,#45277,#45278,#45279,#45280,
#45281,#45282,#45283,#45284,#45285),.UNSPECIFIED.,.F.,.F.,(4,1,1,1,1,1,
1,4),(191.637151868978,192.15328701392,193.15197309348,194.15065917304,
195.1493452526,196.14803133216,197.14671741172,197.920337176157),
 .UNSPECIFIED.);
#732=B_SPLINE_CURVE_WITH_KNOTS('',3,(#45286,#45287,#45288,#45289,#45290,
#45291,#45292,#45293,#45294,#45295,#45296),.UNSPECIFIED.,.F.,.F.,(4,1,1,
1,1,1,1,1,4),(191.637151868978,191.835441659408,192.834127738968,193.832813818528,
194.831499898088,195.830185977648,196.828872057208,197.827558136768,197.920337176158),
 .UNSPECIFIED.);
#733=B_SPLINE_CURVE_WITH_KNOTS('',3,(#45301,#45302,#45303,#45304,#45305,
#45306,#45307,#45308,#45309,#45310),.UNSPECIFIED.,.F.,.F.,(4,1,1,1,1,1,
1,4),(185.353966561798,186.161170536561,187.159856616121,188.158542695681,
189.15722877524,190.1559148548,191.15460093436,191.637151868978),
 .UNSPECIFIED.);
#734=B_SPLINE_CURVE_WITH_KNOTS('',3,(#45311,#45312,#45313,#45314,#45315,
#45316,#45317,#45318,#45319,#45320),.UNSPECIFIED.,.F.,.F.,(4,1,1,1,1,1,
1,4),(185.353966561798,185.843325182048,186.842011261608,187.840697341168,
188.839383420728,189.838069500288,190.836755579848,191.637151868978),
 .UNSPECIFIED.);
#735=B_SPLINE_CURVE_WITH_KNOTS('',3,(#45325,#45326,#45327,#45328,#45329,
#45330,#45331,#45332,#45333,#45334,#45335),.UNSPECIFIED.,.F.,.F.,(4,1,1,
1,1,1,1,1,4),(179.070781254619,179.170367979641,180.169054059201,181.167740138761,
182.166426218321,183.165112297881,184.163798377441,185.162484457001,185.353966561798),
 .UNSPECIFIED.);
#736=B_SPLINE_CURVE_WITH_KNOTS('',3,(#45336,#45337,#45338,#45339,#45340,
#45341,#45342,#45343,#45344,#45345),.UNSPECIFIED.,.F.,.F.,(4,1,1,1,1,1,
1,4),(179.070781254619,179.851208704689,180.849894784249,181.848580863809,
182.847266943368,183.845953022928,184.844639102488,185.353966561798),
 .UNSPECIFIED.);
#737=B_SPLINE_CURVE_WITH_KNOTS('',3,(#45350,#45351,#45352,#45353,#45354,
#45355,#45356,#45357,#45358,#45359),.UNSPECIFIED.,.F.,.F.,(4,1,1,1,1,1,
1,4),(172.787595947439,173.178251502281,174.176937581841,175.175623661401,
176.174309740961,177.172995820521,178.171681900081,179.070781254619),
 .UNSPECIFIED.);
#738=B_SPLINE_CURVE_WITH_KNOTS('',3,(#45360,#45361,#45362,#45363,#45364,
#45365,#45366,#45367,#45368,#45369,#45370),.UNSPECIFIED.,.F.,.F.,(4,1,1,
1,1,1,1,1,4),(172.787595947439,172.860406147769,173.859092227329,174.857778306889,
175.856464386449,176.855150466009,177.853836545569,178.852522625129,179.070781254619),
 .UNSPECIFIED.);
#739=B_SPLINE_CURVE_WITH_KNOTS('',3,(#45375,#45376,#45377,#45378,#45379,
#45380,#45381,#45382,#45383,#45384),.UNSPECIFIED.,.F.,.F.,(4,1,1,1,1,1,
1,4),(166.50441064026,167.186135024922,168.184821104482,169.183507184041,
170.182193263601,171.180879343161,172.179565422721,172.787595947439),
 .UNSPECIFIED.);
#740=B_SPLINE_CURVE_WITH_KNOTS('',3,(#45385,#45386,#45387,#45388,#45389,
#45390,#45391,#45392,#45393,#45394),.UNSPECIFIED.,.F.,.F.,(4,1,1,1,1,1,
1,4),(166.50441064026,166.868289670409,167.866975749969,168.865661829529,
169.864347909089,170.863033988649,171.861720068209,172.787595947439),
 .UNSPECIFIED.);
#741=B_SPLINE_CURVE_WITH_KNOTS('',3,(#45399,#45400,#45401,#45402,#45403,
#45404,#45405,#45406,#45407,#45408),.UNSPECIFIED.,.F.,.F.,(4,1,1,1,1,1,
1,4),(160.22122533308,161.194018547562,162.192704627122,163.191390706682,
164.190076786242,165.188762865802,166.187448945362,166.50441064026),
 .UNSPECIFIED.);
#742=B_SPLINE_CURVE_WITH_KNOTS('',3,(#45409,#45410,#45411,#45412,#45413,
#45414,#45415,#45416,#45417,#45418),.UNSPECIFIED.,.F.,.F.,(4,1,1,1,1,1,
1,4),(160.22122533308,160.87617319305,161.874859272609,162.873545352169,
163.872231431729,164.870917511289,165.869603590849,166.50441064026),
 .UNSPECIFIED.);
#743=B_SPLINE_CURVE_WITH_KNOTS('',3,(#45423,#45424,#45425,#45426,#45427,
#45428,#45429,#45430,#45431,#45432,#45433),.UNSPECIFIED.,.F.,.F.,(4,1,1,
1,1,1,1,1,4),(153.9380400259,154.203215990642,155.201902070202,156.200588149762,
157.199274229322,158.197960308882,159.196646388442,160.195332468002,160.22122533308),
 .UNSPECIFIED.);
#744=B_SPLINE_CURVE_WITH_KNOTS('',3,(#45434,#45435,#45436,#45437,#45438,
#45439,#45440,#45441,#45442,#45443),.UNSPECIFIED.,.F.,.F.,(4,1,1,1,1,1,
1,4),(153.938040025901,154.88405671569,155.88274279525,156.88142887481,
157.88011495437,158.87880103393,159.87748711349,160.22122533308),
 .UNSPECIFIED.);
#745=B_SPLINE_CURVE_WITH_KNOTS('',3,(#45448,#45449,#45450,#45451,#45452,
#45453,#45454,#45455,#45456,#45457),.UNSPECIFIED.,.F.,.F.,(4,1,1,1,1,1,
1,4),(147.654854718721,148.211099513282,149.209785592842,150.208471672402,
151.207157751962,152.205843831522,153.204529911082,153.9380400259),
 .UNSPECIFIED.);
#746=B_SPLINE_CURVE_WITH_KNOTS('',3,(#45458,#45459,#45460,#45461,#45462,
#45463,#45464,#45465,#45466,#45467,#45468),.UNSPECIFIED.,.F.,.F.,(4,1,1,
1,1,1,1,1,4),(147.654854718721,147.89325415877,148.89194023833,149.89062631789,
150.88931239745,151.88799847701,152.88668455657,153.88537063613,153.938040025901),
 .UNSPECIFIED.);
#747=B_SPLINE_CURVE_WITH_KNOTS('',3,(#45473,#45474,#45475,#45476,#45477,
#45478,#45479,#45480,#45481,#45482),.UNSPECIFIED.,.F.,.F.,(4,1,1,1,1,1,
1,4),(141.371669411541,142.218983035923,143.217669115483,144.216355195043,
145.215041274603,146.213727354163,147.212413433723,147.654854718721),
 .UNSPECIFIED.);
#748=B_SPLINE_CURVE_WITH_KNOTS('',3,(#45483,#45484,#45485,#45486,#45487,
#45488,#45489,#45490,#45491,#45492),.UNSPECIFIED.,.F.,.F.,(4,1,1,1,1,1,
1,4),(141.371669411542,141.90113768141,142.89982376097,143.89850984053,
144.89719592009,145.89588199965,146.89456807921,147.654854718721),
 .UNSPECIFIED.);
#749=B_SPLINE_CURVE_WITH_KNOTS('',3,(#45497,#45498,#45499,#45500,#45501,
#45502,#45503,#45504,#45505,#45506,#45507),.UNSPECIFIED.,.F.,.F.,(4,1,1,
1,1,1,1,1,4),(135.088484104362,135.228180479003,136.226866558563,137.225552638123,
138.224238717683,139.222924797243,140.221610876803,141.220296956363,141.371669411541),
 .UNSPECIFIED.);
#750=B_SPLINE_CURVE_WITH_KNOTS('',3,(#45508,#45509,#45510,#45511,#45512,
#45513,#45514,#45515,#45516,#45517),.UNSPECIFIED.,.F.,.F.,(4,1,1,1,1,1,
1,4),(135.088484104362,135.909021204051,136.907707283611,137.906393363171,
138.905079442731,139.903765522291,140.90245160185,141.371669411542),
 .UNSPECIFIED.);
#751=B_SPLINE_CURVE_WITH_KNOTS('',3,(#45522,#45523,#45524,#45525,#45526,
#45527,#45528,#45529,#45530,#45531),.UNSPECIFIED.,.F.,.F.,(4,1,1,1,1,1,
1,4),(128.805298797182,129.236064001643,130.234750081203,131.233436160763,
132.232122240323,133.230808319883,134.229494399443,135.088484104362),
 .UNSPECIFIED.);
#752=B_SPLINE_CURVE_WITH_KNOTS('',3,(#45532,#45533,#45534,#45535,#45536,
#45537,#45538,#45539,#45540,#45541,#45542),.UNSPECIFIED.,.F.,.F.,(4,1,1,
1,1,1,1,1,4),(128.805298797182,128.918218647131,129.916904726691,130.915590806251,
131.914276885811,132.912962965371,133.911649044931,134.910335124491,135.088484104362),
 .UNSPECIFIED.);
#753=B_SPLINE_CURVE_WITH_KNOTS('',3,(#45547,#45548,#45549,#45550,#45551,
#45552,#45553,#45554,#45555,#45556),.UNSPECIFIED.,.F.,.F.,(4,1,1,1,1,1,
1,4),(122.522113490003,123.243947524284,124.242633603844,125.241319683404,
126.240005762964,127.238691842524,128.237377922083,128.805298797182),
 .UNSPECIFIED.);
#754=B_SPLINE_CURVE_WITH_KNOTS('',3,(#45557,#45558,#45559,#45560,#45561,
#45562,#45563,#45564,#45565,#45566),.UNSPECIFIED.,.F.,.F.,(4,1,1,1,1,1,
1,4),(122.522113490003,122.926102169771,123.924788249331,124.923474328891,
125.922160408451,126.920846488011,127.919532567571,128.805298797182),
 .UNSPECIFIED.);
#755=B_SPLINE_CURVE_WITH_KNOTS('',3,(#45571,#45572,#45573,#45574,#45575,
#45576,#45577,#45578,#45579,#45580,#45581),.UNSPECIFIED.,.F.,.F.,(4,1,1,
1,1,1,1,1,4),(116.238928182823,116.253144967364,117.251831046924,118.250517126484,
119.249203206044,120.247889285604,121.246575365164,122.245261444724,122.522113490003),
 .UNSPECIFIED.);
#756=B_SPLINE_CURVE_WITH_KNOTS('',3,(#45582,#45583,#45584,#45585,#45586,
#45587,#45588,#45589,#45590,#45591),.UNSPECIFIED.,.F.,.F.,(4,1,1,1,1,1,
1,4),(116.238928182823,116.933985692412,117.932671771972,118.931357851532,
119.930043931092,120.928730010651,121.927416090211,122.522113490003),
 .UNSPECIFIED.);
#757=B_SPLINE_CURVE_WITH_KNOTS('',3,(#45596,#45597,#45598,#45599,#45600,
#45601,#45602,#45603,#45604,#45605),.UNSPECIFIED.,.F.,.F.,(4,1,1,1,1,1,
1,4),(109.955742875643,110.261028490004,111.259714569564,112.258400649124,
113.257086728684,114.255772808244,115.254458887804,116.238928182823),
 .UNSPECIFIED.);
#758=B_SPLINE_CURVE_WITH_KNOTS('',3,(#45606,#45607,#45608,#45609,#45610,
#45611,#45612,#45613,#45614,#45615),.UNSPECIFIED.,.F.,.F.,(4,1,1,1,1,1,
1,4),(109.955742875644,110.941869215052,111.940555294612,112.939241374172,
113.937927453732,114.936613533292,115.935299612852,116.238928182823),
 .UNSPECIFIED.);
#759=B_SPLINE_CURVE_WITH_KNOTS('',3,(#45620,#45621,#45622,#45623,#45624,
#45625,#45626,#45627,#45628,#45629),.UNSPECIFIED.,.F.,.F.,(4,1,1,1,1,1,
1,4),(103.672557568464,104.268912012645,105.267598092205,106.266284171765,
107.264970251324,108.263656330884,109.262342410444,109.955742875643),
 .UNSPECIFIED.);
#760=B_SPLINE_CURVE_WITH_KNOTS('',3,(#45630,#45631,#45632,#45633,#45634,
#45635,#45636,#45637,#45638,#45639,#45640),.UNSPECIFIED.,.F.,.F.,(4,1,1,
1,1,1,1,1,4),(103.672557568464,103.951066658132,104.949752737692,105.948438817252,
106.947124896812,107.945810976372,108.944497055932,109.943183135492,109.955742875644),
 .UNSPECIFIED.);
#761=B_SPLINE_CURVE_WITH_KNOTS('',3,(#45645,#45646,#45647,#45648,#45649,
#45650,#45651,#45652,#45653,#45654),.UNSPECIFIED.,.F.,.F.,(4,1,1,1,1,1,
1,4),(97.3893722612842,98.2767955352849,99.2754816148449,100.274167694405,
101.272853773965,102.271539853525,103.270225933085,103.672557568464),
 .UNSPECIFIED.);
#762=B_SPLINE_CURVE_WITH_KNOTS('',3,(#45655,#45656,#45657,#45658,#45659,
#45660,#45661,#45662,#45663,#45664),.UNSPECIFIED.,.F.,.F.,(4,1,1,1,1,1,
1,4),(97.3893722612844,97.9589501807726,98.9576362603325,99.9563223398925,
100.955008419452,101.953694499012,102.952380578572,103.672557568464),
 .UNSPECIFIED.);
#763=B_SPLINE_CURVE_WITH_KNOTS('',3,(#45669,#45670,#45671,#45672,#45673,
#45674,#45675,#45676,#45677,#45678,#45679),.UNSPECIFIED.,.F.,.F.,(4,1,1,
1,1,1,1,1,4),(91.1061869541046,91.2859929783653,92.2846790579252,93.2833651374852,
94.2820512170451,95.2807372966051,96.279423376165,97.278109455725,97.3893722612842),
 .UNSPECIFIED.);
#764=B_SPLINE_CURVE_WITH_KNOTS('',3,(#45680,#45681,#45682,#45683,#45684,
#45685,#45686,#45687,#45688,#45689),.UNSPECIFIED.,.F.,.F.,(4,1,1,1,1,1,
1,4),(91.1061869541048,91.9668337034129,92.9655197829728,93.9642058625328,
94.9628919420927,95.9615780216527,96.9602641012126,97.3893722612844),
 .UNSPECIFIED.);
#765=B_SPLINE_CURVE_WITH_KNOTS('',3,(#45694,#45695,#45696,#45697,#45698,
#45699,#45700,#45701,#45702,#45703),.UNSPECIFIED.,.F.,.F.,(4,1,1,1,1,1,
1,4),(84.8230016469251,85.2938765010056,86.2925625805655,87.2912486601255,
88.2899347396854,89.2886208192454,90.2873068988053,91.1061869541046),
 .UNSPECIFIED.);
#766=B_SPLINE_CURVE_WITH_KNOTS('',3,(#45704,#45705,#45706,#45707,#45708,
#45709,#45710,#45711,#45712,#45713,#45714),.UNSPECIFIED.,.F.,.F.,(4,1,1,
1,1,1,1,1,4),(84.8230016469252,84.9760311464932,85.9747172260532,86.9734033056131,
87.9720893851731,88.970775464733,89.969461544293,90.9681476238529,91.1061869541048),
 .UNSPECIFIED.);
#767=B_SPLINE_CURVE_WITH_KNOTS('',3,(#45719,#45720,#45721,#45722,#45723,
#45724,#45725,#45726,#45727,#45728),.UNSPECIFIED.,.F.,.F.,(4,1,1,1,1,1,
1,4),(78.5398163397455,79.3017600236459,80.3004461032058,81.2991321827658,
82.2978182623257,83.2965043418857,84.2951904214456,84.8230016469251),
 .UNSPECIFIED.);
#768=B_SPLINE_CURVE_WITH_KNOTS('',3,(#45729,#45730,#45731,#45732,#45733,
#45734,#45735,#45736,#45737,#45738),.UNSPECIFIED.,.F.,.F.,(4,1,1,1,1,1,
1,4),(78.5398163397457,78.9839146691335,79.9826007486935,80.9812868282534,
81.9799729078134,82.9786589873733,83.9773450669333,84.8230016469252),
 .UNSPECIFIED.);
#769=B_SPLINE_CURVE_WITH_KNOTS('',3,(#45743,#45744,#45745,#45746,#45747,
#45748,#45749,#45750,#45751,#45752,#45753),.UNSPECIFIED.,.F.,.F.,(4,1,1,
1,1,1,1,1,4),(72.2566310325659,72.3109574667262,73.3096435462861,74.3083296258461,
75.307015705406,76.305701784966,77.3043878645259,78.3030739440859,78.5398163397455),
 .UNSPECIFIED.);
#770=B_SPLINE_CURVE_WITH_KNOTS('',3,(#45754,#45755,#45756,#45757,#45758,
#45759,#45760,#45761,#45762,#45763),.UNSPECIFIED.,.F.,.F.,(4,1,1,1,1,1,
1,4),(72.256631032566,72.9917981917738,73.9904842713337,74.9891703508937,
75.9878564304536,76.9865425100136,77.9852285895736,78.5398163397457),
 .UNSPECIFIED.);
#771=B_SPLINE_CURVE_WITH_KNOTS('',3,(#45768,#45769,#45770,#45771,#45772,
#45773,#45774,#45775,#45776,#45777),.UNSPECIFIED.,.F.,.F.,(4,1,1,1,1,1,
1,4),(65.9734457253862,66.3188409893665,67.3175270689264,68.3162131484864,
69.3148992280463,70.3135853076063,71.3122713871662,72.2566310325659),
 .UNSPECIFIED.);
#772=B_SPLINE_CURVE_WITH_KNOTS('',3,(#45778,#45779,#45780,#45781,#45782,
#45783,#45784,#45785,#45786,#45787,#45788),.UNSPECIFIED.,.F.,.F.,(4,1,1,
1,1,1,1,1,4),(65.9734457253864,66.0009956348541,66.9996817144141,67.998367793974,
68.997053873534,69.9957399530939,70.9944260326539,71.9931121122139,72.256631032566),
 .UNSPECIFIED.);
#773=B_SPLINE_CURVE_WITH_KNOTS('',3,(#45793,#45794,#45795,#45796,#45797,
#45798,#45799,#45800,#45801,#45802),.UNSPECIFIED.,.F.,.F.,(4,1,1,1,1,1,
1,4),(59.6902604182067,60.3267245120068,61.3254105915667,62.3240966711267,
63.3227827506866,64.3214688302466,65.3201549098065,65.9734457253862),
 .UNSPECIFIED.);
#774=B_SPLINE_CURVE_WITH_KNOTS('',3,(#45803,#45804,#45805,#45806,#45807,
#45808,#45809,#45810,#45811,#45812),.UNSPECIFIED.,.F.,.F.,(4,1,1,1,1,1,
1,4),(59.6902604182069,60.0088791574944,61.0075652370544,62.0062513166143,
63.0049373961743,64.0036234757342,65.0023095552942,65.9734457253864),
 .UNSPECIFIED.);
#775=B_SPLINE_CURVE_WITH_KNOTS('',3,(#45817,#45818,#45819,#45820,#45821,
#45822,#45823,#45824,#45825,#45826),.UNSPECIFIED.,.F.,.F.,(4,1,1,1,1,1,
1,4),(53.4070751110271,54.3346080346471,55.333294114207,56.331980193767,
57.3306662733269,58.3293523528869,59.3280384324468,59.6902604182067),
 .UNSPECIFIED.);
#776=B_SPLINE_CURVE_WITH_KNOTS('',3,(#45827,#45828,#45829,#45830,#45831,
#45832,#45833,#45834,#45835,#45836),.UNSPECIFIED.,.F.,.F.,(4,1,1,1,1,1,
1,4),(53.4070751110273,54.0167626801347,55.0154487596947,56.0141348392546,
57.0128209188146,58.0115069983745,59.0101930779345,59.6902604182069),
 .UNSPECIFIED.);
#777=B_SPLINE_CURVE_WITH_KNOTS('',3,(#45841,#45842,#45843,#45844,#45845,
#45846,#45847,#45848,#45849,#45850,#45851),.UNSPECIFIED.,.F.,.F.,(4,1,1,
1,1,1,1,1,4),(47.1238898038475,47.3438054777274,48.3424915572874,49.3411776368473,
50.3398637164073,51.3385497959672,52.3372358755272,53.3359219550871,53.4070751110271),
 .UNSPECIFIED.);
#778=B_SPLINE_CURVE_WITH_KNOTS('',3,(#45852,#45853,#45854,#45855,#45856,
#45857,#45858,#45859,#45860,#45861),.UNSPECIFIED.,.F.,.F.,(4,1,1,1,1,1,
1,4),(47.1238898038477,48.024646202775,49.023332282335,50.0220183618949,
51.0207044414549,52.0193905210148,53.0180766005748,53.4070751110273),
 .UNSPECIFIED.);
#779=B_SPLINE_CURVE_WITH_KNOTS('',3,(#45866,#45867,#45868,#45869,#45870,
#45871,#45872,#45873,#45874,#45875),.UNSPECIFIED.,.F.,.F.,(4,1,1,1,1,1,
1,4),(40.8407044966679,41.3516890003677,42.3503750799277,43.3490611594876,
44.3477472390476,45.3464333186075,46.3451193981675,47.1238898038475),
 .UNSPECIFIED.);
#780=B_SPLINE_CURVE_WITH_KNOTS('',3,(#45876,#45877,#45878,#45879,#45880,
#45881,#45882,#45883,#45884,#45885,#45886),.UNSPECIFIED.,.F.,.F.,(4,1,1,
1,1,1,1,1,4),(40.8407044966681,41.0338436458553,42.0325297254153,43.0312158049753,
44.0299018845352,45.0285879640952,46.0272740436551,47.0259601232151,47.1238898038477),
 .UNSPECIFIED.);
#781=B_SPLINE_CURVE_WITH_KNOTS('',3,(#45891,#45892,#45893,#45894,#45895,
#45896,#45897,#45898,#45899,#45900),.UNSPECIFIED.,.F.,.F.,(4,1,1,1,1,1,
1,4),(34.5575191894883,35.359572523008,36.358258602568,37.3569446821279,
38.3556307616879,39.3543168412478,40.3530029208078,40.8407044966679),
 .UNSPECIFIED.);
#782=B_SPLINE_CURVE_WITH_KNOTS('',3,(#45901,#45902,#45903,#45904,#45905,
#45906,#45907,#45908,#45909,#45910),.UNSPECIFIED.,.F.,.F.,(4,1,1,1,1,1,
1,4),(34.5575191894885,35.0417271684956,36.0404132480556,37.0390993276155,
38.0377854071755,39.0364714867355,40.0351575662954,40.8407044966681),
 .UNSPECIFIED.);
#783=B_SPLINE_CURVE_WITH_KNOTS('',3,(#45915,#45916,#45917,#45918,#45919,
#45920,#45921,#45922,#45923,#45924,#45925),.UNSPECIFIED.,.F.,.F.,(4,1,1,
1,1,1,1,1,4),(28.2743338823087,28.3687699660883,29.3674560456483,30.3661421252082,
31.3648282047682,32.3635142843282,33.3622003638881,34.3608864434481,34.5575191894883),
 .UNSPECIFIED.);
#784=B_SPLINE_CURVE_WITH_KNOTS('',3,(#45926,#45927,#45928,#45929,#45930,
#45931,#45932,#45933,#45934,#45935),.UNSPECIFIED.,.F.,.F.,(4,1,1,1,1,1,
1,4),(28.2743338823089,29.0496106911359,30.0482967706959,31.0469828502558,
32.0456689298158,33.0443550093757,34.0430410889357,34.5575191894885),
 .UNSPECIFIED.);
#785=B_SPLINE_CURVE_WITH_KNOTS('',3,(#45940,#45941,#45942,#45943,#45944,
#45945,#45946,#45947,#45948,#45949),.UNSPECIFIED.,.F.,.F.,(4,1,1,1,1,1,
1,4),(21.9911485751291,22.3766534887286,23.3753395682886,24.3740256478485,
25.3727117274085,26.3713978069684,27.3700838865284,28.2743338823087),
 .UNSPECIFIED.);
#786=B_SPLINE_CURVE_WITH_KNOTS('',3,(#45950,#45951,#45952,#45953,#45954,
#45955,#45956,#45957,#45958,#45959,#45960),.UNSPECIFIED.,.F.,.F.,(4,1,1,
1,1,1,1,1,4),(21.9911485751293,22.0588081342163,23.0574942137762,24.0561802933362,
25.0548663728961,26.0535524524561,27.052238532016,28.050924611576,28.2743338823089),
 .UNSPECIFIED.);
#787=B_SPLINE_CURVE_WITH_KNOTS('',3,(#45965,#45966,#45967,#45968,#45969,
#45970,#45971,#45972,#45973,#45974),.UNSPECIFIED.,.F.,.F.,(4,1,1,1,1,1,
1,4),(15.7079632679496,16.3845370113689,17.3832230909289,18.3819091704888,
19.3805952500488,20.3792813296087,21.3779674091687,21.9911485751291),
 .UNSPECIFIED.);
#788=B_SPLINE_CURVE_WITH_KNOTS('',3,(#45975,#45976,#45977,#45978,#45979,
#45980,#45981,#45982,#45983,#45984),.UNSPECIFIED.,.F.,.F.,(4,1,1,1,1,1,
1,4),(15.7079632679497,16.0666916568566,17.0653777364165,18.0640638159765,
19.0627498955364,20.0614359750964,21.0601220546563,21.9911485751293),
 .UNSPECIFIED.);
#789=B_SPLINE_CURVE_WITH_KNOTS('',3,(#45987,#45988,#45989,#45990,#45991,
#45992,#45993,#45994,#45995,#45996,#45997,#45998,#45999,#46000,#46001,#46002,
#46003,#46004,#46005,#46006,#46007,#46008,#46009,#46010,#46011,#46012,#46013,
#46014,#46015,#46016,#46017,#46018,#46019,#46020,#46021,#46022,#46023,#46024,
#46025,#46026,#46027,#46028,#46029,#46030,#46031,#46032,#46033,#46034,#46035,
#46036,#46037,#46038),.UNSPECIFIED.,.F.,.F.,(4,3,3,3,3,3,3,3,3,3,3,3,3,
3,3,3,3,4),(-0.276631791712715,-0.26755901985898,-0.245786814899969,-0.233874251841385,
-0.212417712774227,-0.201844136596455,-0.173306013186041,-0.162876402370629,
-0.153623752254054,-0.140564570666302,-0.120812346575674,-0.110858182676873,
-0.10074618282354,-0.0755596371176548,-0.0588540251780687,-0.0493417440450129,
-0.0183248504906759,0.),.UNSPECIFIED.);
#790=B_SPLINE_CURVE_WITH_KNOTS('',3,(#46043,#46044,#46045,#46046,#46047,
#46048,#46049,#46050,#46051,#46052,#46053,#46054,#46055,#46056,#46057,#46058,
#46059,#46060,#46061,#46062,#46063,#46064,#46065,#46066,#46067,#46068,#46069,
#46070,#46071,#46072,#46073,#46074,#46075,#46076,#46077,#46078,#46079,#46080,
#46081,#46082,#46083,#46084,#46085,#46086,#46087,#46088,#46089,#46090,#46091,
#46092,#46093,#46094),.UNSPECIFIED.,.F.,.F.,(4,3,3,3,3,3,3,3,3,3,3,3,3,
3,3,3,3,4),(-0.275362278356787,-0.264292581061059,-0.242714596523907,-0.228543028021742,
-0.209227773008753,-0.199395258896952,-0.189100003351452,-0.159713559956535,
-0.147814894797435,-0.139076691589832,-0.125504176784125,-0.103148327528027,
-0.0941264284167034,-0.0661327433935608,-0.0498049250752028,-0.0407969165022222,
-0.0145455879908767,0.),.UNSPECIFIED.);
#791=B_SPLINE_CURVE_WITH_KNOTS('',3,(#47587,#47588,#47589,#47590,#47591,
#47592,#47593,#47594,#47595,#47596,#47597,#47598,#47599,#47600,#47601,#47602,
#47603,#47604,#47605),.UNSPECIFIED.,.F.,.F.,(4,3,3,3,3,3,4),(361.77757843857,
362.523046880262,363.521732959822,364.520419039382,365.519105118942,366.517791198502,
367.440676763862),.UNSPECIFIED.);
#792=B_SPLINE_CURVE_WITH_KNOTS('',3,(#47607,#47608,#47609,#47610,#47611,
#47612,#47613,#47614,#47615,#47616,#47617,#47618,#47619,#47620,#47621,#47622,
#47623,#47624,#47625,#47626,#47627,#47628,#47629,#47630,#47631,#47632,#47633,
#47634,#47635,#47636,#47637,#47638,#47639,#47640,#47641,#47642,#47643,#47644,
#47645,#47646,#47647,#47648,#47649,#47650,#47651,#47652,#47653,#47654,#47655,
#47656,#47657,#47658),.UNSPECIFIED.,.F.,.F.,(4,3,3,3,3,3,3,3,3,3,3,3,3,
3,3,3,3,4),(-0.276631791712692,-0.267559019858928,-0.245786815023485,-0.233874252356153,
-0.21241770641256,-0.201844136492789,-0.173306013103481,-0.162876405863916,
-0.153623758375204,-0.140564570666252,-0.12081234527961,-0.110858177928118,
-0.100746182189666,-0.0755596366422492,-0.058854022142393,-0.04934174195364,
-0.018324847486917,0.),.UNSPECIFIED.);
#793=B_SPLINE_CURVE_WITH_KNOTS('',3,(#47659,#47660,#47661,#47662,#47663),
 .UNSPECIFIED.,.F.,.F.,(4,1,4),(14.1451200119366,15.0680055772966,15.7079632679497),
 .UNSPECIFIED.);
#794=B_SPLINE_CURVE_WITH_KNOTS('',3,(#47666,#47667,#47668,#47669,#47670,
#47671,#47672,#47673,#47674,#47675,#47676,#47677,#47678,#47679,#47680,#47681,
#47682,#47683,#47684,#47685,#47686,#47687,#47688,#47689,#47690,#47691,#47692,
#47693,#47694,#47695,#47696,#47697,#47698,#47699,#47700,#47701,#47702,#47703,
#47704,#47705,#47706,#47707,#47708,#47709,#47710,#47711,#47712,#47713,#47714,
#47715,#47716,#47717),.UNSPECIFIED.,.F.,.F.,(4,3,3,3,3,3,3,3,3,3,3,3,3,
3,3,3,3,4),(-0.275362278356907,-0.264292581061165,-0.242714595883773,-0.22854302749595,
-0.209227769645797,-0.199395250917095,-0.189100000879922,-0.159713556370167,
-0.147814883828647,-0.139076671830681,-0.125504176784174,-0.103148391122983,
-0.0941264875184657,-0.0661328024083947,-0.0498050734898823,-0.0407969659451433,
-0.0145456388647011,0.),.UNSPECIFIED.);
#795=B_SPLINE_CURVE_WITH_KNOTS('',3,(#47720,#47721,#47722,#47723),
 .UNSPECIFIED.,.F.,.F.,(4,4),(15.385850931809,15.7079632679496),
 .UNSPECIFIED.);
#796=B_SPLINE_CURVE_WITH_KNOTS('',3,(#49216,#49217,#49218,#49219,#49220,
#49221,#49222,#49223,#49224,#49225,#49226,#49227,#49228,#49229,#49230,#49231),
 .UNSPECIFIED.,.F.,.F.,(4,3,3,3,3,4),(-369.513849437182,-368.515163357622,
-367.516477278062,-366.517791198502,-365.519105118942,-364.746860152556),
 .UNSPECIFIED.);
#893=SHAPE_REPRESENTATION_RELATIONSHIP('SRR','None',#53738,#909);
#909=ADVANCED_BREP_SHAPE_REPRESENTATION('',(#941),#53648);
#925=STYLED_ITEM('',(#53965),#941);
#941=MANIFOLD_SOLID_BREP('ISO_4762_M3x30_A2',#23317);
#1117=CYLINDRICAL_SURFACE('',#25039,0.14635);
#1118=CYLINDRICAL_SURFACE('',#25043,0.14635);
#1119=CYLINDRICAL_SURFACE('',#25044,0.14635);
#1120=CYLINDRICAL_SURFACE('',#25045,0.14635);
#1121=CYLINDRICAL_SURFACE('',#25046,0.14635);
#1122=CYLINDRICAL_SURFACE('',#25047,0.14635);
#1123=CYLINDRICAL_SURFACE('',#25048,0.14635);
#1124=CYLINDRICAL_SURFACE('',#25049,0.14635);
#1125=CYLINDRICAL_SURFACE('',#25050,0.14635);
#1126=CYLINDRICAL_SURFACE('',#25051,0.14635);
#1127=CYLINDRICAL_SURFACE('',#25052,0.14635);
#1128=CYLINDRICAL_SURFACE('',#25053,0.14635);
#1129=CYLINDRICAL_SURFACE('',#25054,0.14635);
#1130=CYLINDRICAL_SURFACE('',#25055,0.14635);
#1131=CYLINDRICAL_SURFACE('',#25056,0.14635);
#1132=CYLINDRICAL_SURFACE('',#25057,0.14635);
#1133=CYLINDRICAL_SURFACE('',#25058,0.14635);
#1134=CYLINDRICAL_SURFACE('',#25059,0.14635);
#1135=CYLINDRICAL_SURFACE('',#25060,0.14635);
#1136=CYLINDRICAL_SURFACE('',#25061,0.14635);
#1137=CYLINDRICAL_SURFACE('',#25062,0.14635);
#1138=CYLINDRICAL_SURFACE('',#25063,0.14635);
#1139=CYLINDRICAL_SURFACE('',#25064,0.14635);
#1140=CYLINDRICAL_SURFACE('',#25065,0.14635);
#1141=CYLINDRICAL_SURFACE('',#25066,0.14635);
#1142=CYLINDRICAL_SURFACE('',#25067,0.14635);
#1143=CYLINDRICAL_SURFACE('',#25068,0.14635);
#1144=CYLINDRICAL_SURFACE('',#25069,0.14635);
#1145=CYLINDRICAL_SURFACE('',#25070,0.14635);
#1146=CYLINDRICAL_SURFACE('',#25071,0.14635);
#1147=CYLINDRICAL_SURFACE('',#25072,0.14635);
#1148=CYLINDRICAL_SURFACE('',#25073,0.14635);
#1149=CYLINDRICAL_SURFACE('',#25074,0.14635);
#1150=CYLINDRICAL_SURFACE('',#25075,0.14635);
#1151=CYLINDRICAL_SURFACE('',#25076,0.14635);
#1152=CYLINDRICAL_SURFACE('',#25077,0.14635);
#1153=CYLINDRICAL_SURFACE('',#25078,0.14635);
#1154=CYLINDRICAL_SURFACE('',#25079,0.14635);
#1155=CYLINDRICAL_SURFACE('',#25080,0.14635);
#1156=CYLINDRICAL_SURFACE('',#25081,0.14635);
#1157=CYLINDRICAL_SURFACE('',#25082,0.14635);
#1158=CYLINDRICAL_SURFACE('',#25083,0.14635);
#1159=CYLINDRICAL_SURFACE('',#25084,0.14635);
#1160=CYLINDRICAL_SURFACE('',#25085,0.14635);
#1161=CYLINDRICAL_SURFACE('',#25086,0.14635);
#1162=CYLINDRICAL_SURFACE('',#25087,0.14635);
#1163=CYLINDRICAL_SURFACE('',#25088,0.14635);
#1164=CYLINDRICAL_SURFACE('',#25089,0.14635);
#1165=CYLINDRICAL_SURFACE('',#25090,0.14635);
#1166=CYLINDRICAL_SURFACE('',#25091,0.14635);
#1167=CYLINDRICAL_SURFACE('',#25092,0.14635);
#1168=CYLINDRICAL_SURFACE('',#25093,0.14635);
#1169=CYLINDRICAL_SURFACE('',#25094,0.14635);
#1170=CYLINDRICAL_SURFACE('',#25095,0.14635);
#1171=CYLINDRICAL_SURFACE('',#25096,0.14635);
#1172=CYLINDRICAL_SURFACE('',#25097,0.14635);
#1173=CYLINDRICAL_SURFACE('',#25098,0.14635);
#1174=CYLINDRICAL_SURFACE('',#25099,0.14635);
#1175=CYLINDRICAL_SURFACE('',#25100,0.117775);
#1176=CYLINDRICAL_SURFACE('',#25102,0.117775);
#1177=CYLINDRICAL_SURFACE('',#25103,0.117775);
#1178=CYLINDRICAL_SURFACE('',#25104,0.117775);
#1179=CYLINDRICAL_SURFACE('',#25105,0.117775);
#1180=CYLINDRICAL_SURFACE('',#25106,0.117775);
#1181=CYLINDRICAL_SURFACE('',#25107,0.117775);
#1182=CYLINDRICAL_SURFACE('',#25108,0.117775);
#1183=CYLINDRICAL_SURFACE('',#25109,0.117775);
#1184=CYLINDRICAL_SURFACE('',#25110,0.117775);
#1185=CYLINDRICAL_SURFACE('',#25111,0.117775);
#1186=CYLINDRICAL_SURFACE('',#25112,0.117775);
#1187=CYLINDRICAL_SURFACE('',#25113,0.117775);
#1188=CYLINDRICAL_SURFACE('',#25114,0.117775);
#1189=CYLINDRICAL_SURFACE('',#25115,0.117775);
#1190=CYLINDRICAL_SURFACE('',#25116,0.117775);
#1191=CYLINDRICAL_SURFACE('',#25117,0.117775);
#1192=CYLINDRICAL_SURFACE('',#25118,0.117775);
#1193=CYLINDRICAL_SURFACE('',#25119,0.117775);
#1194=CYLINDRICAL_SURFACE('',#25120,0.117775);
#1195=CYLINDRICAL_SURFACE('',#25121,0.117775);
#1196=CYLINDRICAL_SURFACE('',#25122,0.117775);
#1197=CYLINDRICAL_SURFACE('',#25123,0.117775);
#1198=CYLINDRICAL_SURFACE('',#25124,0.117775);
#1199=CYLINDRICAL_SURFACE('',#25125,0.117775);
#1200=CYLINDRICAL_SURFACE('',#25126,0.117775);
#1201=CYLINDRICAL_SURFACE('',#25127,0.117775);
#1202=CYLINDRICAL_SURFACE('',#25128,0.117775);
#1203=CYLINDRICAL_SURFACE('',#25129,0.117775);
#1204=CYLINDRICAL_SURFACE('',#25130,0.117775);
#1205=CYLINDRICAL_SURFACE('',#25131,0.117775);
#1206=CYLINDRICAL_SURFACE('',#25132,0.117775);
#1207=CYLINDRICAL_SURFACE('',#25133,0.117775);
#1208=CYLINDRICAL_SURFACE('',#25134,0.117775);
#1209=CYLINDRICAL_SURFACE('',#25135,0.117775);
#1210=CYLINDRICAL_SURFACE('',#25136,0.117775);
#1211=CYLINDRICAL_SURFACE('',#25137,0.117775);
#1212=CYLINDRICAL_SURFACE('',#25138,0.117775);
#1213=CYLINDRICAL_SURFACE('',#25139,0.117775);
#1214=CYLINDRICAL_SURFACE('',#25140,0.117775);
#1215=CYLINDRICAL_SURFACE('',#25141,0.117775);
#1216=CYLINDRICAL_SURFACE('',#25142,0.117775);
#1217=CYLINDRICAL_SURFACE('',#25143,0.117775);
#1218=CYLINDRICAL_SURFACE('',#25144,0.117775);
#1219=CYLINDRICAL_SURFACE('',#25145,0.117775);
#1220=CYLINDRICAL_SURFACE('',#25146,0.117775);
#1221=CYLINDRICAL_SURFACE('',#25147,0.117775);
#1222=CYLINDRICAL_SURFACE('',#25148,0.117775);
#1223=CYLINDRICAL_SURFACE('',#25149,0.117775);
#1224=CYLINDRICAL_SURFACE('',#25150,0.117775);
#1225=CYLINDRICAL_SURFACE('',#25151,0.117775);
#1226=CYLINDRICAL_SURFACE('',#25152,0.117775);
#1227=CYLINDRICAL_SURFACE('',#25153,0.117775);
#1228=CYLINDRICAL_SURFACE('',#25154,0.117775);
#1229=CYLINDRICAL_SURFACE('',#25155,0.117775);
#1230=CYLINDRICAL_SURFACE('',#25156,0.117775);
#1231=CYLINDRICAL_SURFACE('',#25157,0.117775);
#1232=CYLINDRICAL_SURFACE('',#25158,0.117775);
#1233=CYLINDRICAL_SURFACE('',#25159,0.117775);
#1234=CYLINDRICAL_SURFACE('',#25165,0.117775);
#1235=CYLINDRICAL_SURFACE('',#25307,0.275);
#1236=CYLINDRICAL_SURFACE('',#25363,0.14635);
#1442=FACE_BOUND('',#4885,.T.);
#1443=FACE_BOUND('',#4891,.T.);
#1444=FACE_BOUND('',#4893,.T.);
#1996=PLANE('',#25160);
#1997=PLANE('',#25163);
#1998=PLANE('',#25166);
#1999=PLANE('',#25168);
#2000=PLANE('',#25169);
#2001=PLANE('',#25170);
#2002=PLANE('',#25172);
#2003=PLANE('',#25173);
#2004=PLANE('',#25174);
#2005=PLANE('',#25176);
#2006=PLANE('',#25177);
#2007=PLANE('',#25178);
#2008=PLANE('',#25180);
#2009=PLANE('',#25181);
#2010=PLANE('',#25182);
#2011=PLANE('',#25184);
#2012=PLANE('',#25185);
#2013=PLANE('',#25186);
#2014=PLANE('',#25188);
#2015=PLANE('',#25189);
#2016=PLANE('',#25190);
#2017=PLANE('',#25192);
#2018=PLANE('',#25193);
#2019=PLANE('',#25194);
#2020=PLANE('',#25196);
#2021=PLANE('',#25197);
#2022=PLANE('',#25198);
#2023=PLANE('',#25200);
#2024=PLANE('',#25201);
#2025=PLANE('',#25202);
#2026=PLANE('',#25204);
#2027=PLANE('',#25205);
#2028=PLANE('',#25206);
#2029=PLANE('',#25208);
#2030=PLANE('',#25209);
#2031=PLANE('',#25210);
#2032=PLANE('',#25212);
#2033=PLANE('',#25213);
#2034=PLANE('',#25214);
#2035=PLANE('',#25216);
#2036=PLANE('',#25217);
#2037=PLANE('',#25218);
#2038=PLANE('',#25220);
#2039=PLANE('',#25221);
#2040=PLANE('',#25222);
#2041=PLANE('',#25224);
#2042=PLANE('',#25225);
#2043=PLANE('',#25226);
#2044=PLANE('',#25228);
#2045=PLANE('',#25229);
#2046=PLANE('',#25230);
#2047=PLANE('',#25232);
#2048=PLANE('',#25233);
#2049=PLANE('',#25234);
#2050=PLANE('',#25237);
#2051=PLANE('',#25238);
#2052=PLANE('',#25239);
#2053=PLANE('',#25241);
#2054=PLANE('',#25242);
#2055=PLANE('',#25243);
#2056=PLANE('',#25245);
#2057=PLANE('',#25246);
#2058=PLANE('',#25247);
#2059=PLANE('',#25249);
#2060=PLANE('',#25250);
#2061=PLANE('',#25251);
#2062=PLANE('',#25253);
#2063=PLANE('',#25254);
#2064=PLANE('',#25255);
#2065=PLANE('',#25257);
#2066=PLANE('',#25258);
#2067=PLANE('',#25259);
#2068=PLANE('',#25261);
#2069=PLANE('',#25262);
#2070=PLANE('',#25263);
#2071=PLANE('',#25265);
#2072=PLANE('',#25266);
#2073=PLANE('',#25267);
#2074=PLANE('',#25269);
#2075=PLANE('',#25270);
#2076=PLANE('',#25271);
#2077=PLANE('',#25273);
#2078=PLANE('',#25274);
#2079=PLANE('',#25275);
#2080=PLANE('',#25277);
#2081=PLANE('',#25278);
#2082=PLANE('',#25279);
#2083=PLANE('',#25281);
#2084=PLANE('',#25282);
#2085=PLANE('',#25283);
#2086=PLANE('',#25285);
#2087=PLANE('',#25286);
#2088=PLANE('',#25287);
#2089=PLANE('',#25289);
#2090=PLANE('',#25290);
#2091=PLANE('',#25291);
#2092=PLANE('',#25293);
#2093=PLANE('',#25294);
#2094=PLANE('',#25295);
#2095=PLANE('',#25297);
#2096=PLANE('',#25298);
#2097=PLANE('',#25299);
#2098=PLANE('',#25301);
#2099=PLANE('',#25302);
#2100=PLANE('',#25303);
#2101=PLANE('',#25305);
#2102=PLANE('',#25306);
#2103=PLANE('',#25346);
#2104=PLANE('',#25347);
#2105=PLANE('',#25348);
#2106=PLANE('',#25353);
#2107=PLANE('',#25354);
#2108=PLANE('',#25355);
#2109=PLANE('',#25356);
#2110=PLANE('',#25357);
#2111=PLANE('',#25358);
#2112=PLANE('',#25359);
#2113=PLANE('',#25360);
#2114=PLANE('',#25367);
#2115=PLANE('',#25368);
#3152=FACE_OUTER_BOUND('',#4645,.T.);
#3153=FACE_OUTER_BOUND('',#4646,.T.);
#3154=FACE_OUTER_BOUND('',#4647,.T.);
#3155=FACE_OUTER_BOUND('',#4648,.T.);
#3156=FACE_OUTER_BOUND('',#4649,.T.);
#3157=FACE_OUTER_BOUND('',#4650,.T.);
#3158=FACE_OUTER_BOUND('',#4651,.T.);
#3159=FACE_OUTER_BOUND('',#4652,.T.);
#3160=FACE_OUTER_BOUND('',#4653,.T.);
#3161=FACE_OUTER_BOUND('',#4654,.T.);
#3162=FACE_OUTER_BOUND('',#4655,.T.);
#3163=FACE_OUTER_BOUND('',#4656,.T.);
#3164=FACE_OUTER_BOUND('',#4657,.T.);
#3165=FACE_OUTER_BOUND('',#4658,.T.);
#3166=FACE_OUTER_BOUND('',#4659,.T.);
#3167=FACE_OUTER_BOUND('',#4660,.T.);
#3168=FACE_OUTER_BOUND('',#4661,.T.);
#3169=FACE_OUTER_BOUND('',#4662,.T.);
#3170=FACE_OUTER_BOUND('',#4663,.T.);
#3171=FACE_OUTER_BOUND('',#4664,.T.);
#3172=FACE_OUTER_BOUND('',#4665,.T.);
#3173=FACE_OUTER_BOUND('',#4666,.T.);
#3174=FACE_OUTER_BOUND('',#4667,.T.);
#3175=FACE_OUTER_BOUND('',#4668,.T.);
#3176=FACE_OUTER_BOUND('',#4669,.T.);
#3177=FACE_OUTER_BOUND('',#4670,.T.);
#3178=FACE_OUTER_BOUND('',#4671,.T.);
#3179=FACE_OUTER_BOUND('',#4672,.T.);
#3180=FACE_OUTER_BOUND('',#4673,.T.);
#3181=FACE_OUTER_BOUND('',#4674,.T.);
#3182=FACE_OUTER_BOUND('',#4675,.T.);
#3183=FACE_OUTER_BOUND('',#4676,.T.);
#3184=FACE_OUTER_BOUND('',#4677,.T.);
#3185=FACE_OUTER_BOUND('',#4678,.T.);
#3186=FACE_OUTER_BOUND('',#4679,.T.);
#3187=FACE_OUTER_BOUND('',#4680,.T.);
#3188=FACE_OUTER_BOUND('',#4681,.T.);
#3189=FACE_OUTER_BOUND('',#4682,.T.);
#3190=FACE_OUTER_BOUND('',#4683,.T.);
#3191=FACE_OUTER_BOUND('',#4684,.T.);
#3192=FACE_OUTER_BOUND('',#4685,.T.);
#3193=FACE_OUTER_BOUND('',#4686,.T.);
#3194=FACE_OUTER_BOUND('',#4687,.T.);
#3195=FACE_OUTER_BOUND('',#4688,.T.);
#3196=FACE_OUTER_BOUND('',#4689,.T.);
#3197=FACE_OUTER_BOUND('',#4690,.T.);
#3198=FACE_OUTER_BOUND('',#4691,.T.);
#3199=FACE_OUTER_BOUND('',#4692,.T.);
#3200=FACE_OUTER_BOUND('',#4693,.T.);
#3201=FACE_OUTER_BOUND('',#4694,.T.);
#3202=FACE_OUTER_BOUND('',#4695,.T.);
#3203=FACE_OUTER_BOUND('',#4696,.T.);
#3204=FACE_OUTER_BOUND('',#4697,.T.);
#3205=FACE_OUTER_BOUND('',#4698,.T.);
#3206=FACE_OUTER_BOUND('',#4699,.T.);
#3207=FACE_OUTER_BOUND('',#4700,.T.);
#3208=FACE_OUTER_BOUND('',#4701,.T.);
#3209=FACE_OUTER_BOUND('',#4702,.T.);
#3210=FACE_OUTER_BOUND('',#4703,.T.);
#3211=FACE_OUTER_BOUND('',#4704,.T.);
#3212=FACE_OUTER_BOUND('',#4705,.T.);
#3213=FACE_OUTER_BOUND('',#4706,.T.);
#3214=FACE_OUTER_BOUND('',#4707,.T.);
#3215=FACE_OUTER_BOUND('',#4708,.T.);
#3216=FACE_OUTER_BOUND('',#4709,.T.);
#3217=FACE_OUTER_BOUND('',#4710,.T.);
#3218=FACE_OUTER_BOUND('',#4711,.T.);
#3219=FACE_OUTER_BOUND('',#4712,.T.);
#3220=FACE_OUTER_BOUND('',#4713,.T.);
#3221=FACE_OUTER_BOUND('',#4714,.T.);
#3222=FACE_OUTER_BOUND('',#4715,.T.);
#3223=FACE_OUTER_BOUND('',#4716,.T.);
#3224=FACE_OUTER_BOUND('',#4717,.T.);
#3225=FACE_OUTER_BOUND('',#4718,.T.);
#3226=FACE_OUTER_BOUND('',#4719,.T.);
#3227=FACE_OUTER_BOUND('',#4720,.T.);
#3228=FACE_OUTER_BOUND('',#4721,.T.);
#3229=FACE_OUTER_BOUND('',#4722,.T.);
#3230=FACE_OUTER_BOUND('',#4723,.T.);
#3231=FACE_OUTER_BOUND('',#4724,.T.);
#3232=FACE_OUTER_BOUND('',#4725,.T.);
#3233=FACE_OUTER_BOUND('',#4726,.T.);
#3234=FACE_OUTER_BOUND('',#4727,.T.);
#3235=FACE_OUTER_BOUND('',#4728,.T.);
#3236=FACE_OUTER_BOUND('',#4729,.T.);
#3237=FACE_OUTER_BOUND('',#4730,.T.);
#3238=FACE_OUTER_BOUND('',#4731,.T.);
#3239=FACE_OUTER_BOUND('',#4732,.T.);
#3240=FACE_OUTER_BOUND('',#4733,.T.);
#3241=FACE_OUTER_BOUND('',#4734,.T.);
#3242=FACE_OUTER_BOUND('',#4735,.T.);
#3243=FACE_OUTER_BOUND('',#4736,.T.);
#3244=FACE_OUTER_BOUND('',#4737,.T.);
#3245=FACE_OUTER_BOUND('',#4738,.T.);
#3246=FACE_OUTER_BOUND('',#4739,.T.);
#3247=FACE_OUTER_BOUND('',#4740,.T.);
#3248=FACE_OUTER_BOUND('',#4741,.T.);
#3249=FACE_OUTER_BOUND('',#4742,.T.);
#3250=FACE_OUTER_BOUND('',#4743,.T.);
#3251=FACE_OUTER_BOUND('',#4744,.T.);
#3252=FACE_OUTER_BOUND('',#4745,.T.);
#3253=FACE_OUTER_BOUND('',#4746,.T.);
#3254=FACE_OUTER_BOUND('',#4747,.T.);
#3255=FACE_OUTER_BOUND('',#4748,.T.);
#3256=FACE_OUTER_BOUND('',#4749,.T.);
#3257=FACE_OUTER_BOUND('',#4750,.T.);
#3258=FACE_OUTER_BOUND('',#4751,.T.);
#3259=FACE_OUTER_BOUND('',#4752,.T.);
#3260=FACE_OUTER_BOUND('',#4753,.T.);
#3261=FACE_OUTER_BOUND('',#4754,.T.);
#3262=FACE_OUTER_BOUND('',#4755,.T.);
#3263=FACE_OUTER_BOUND('',#4756,.T.);
#3264=FACE_OUTER_BOUND('',#4757,.T.);
#3265=FACE_OUTER_BOUND('',#4758,.T.);
#3266=FACE_OUTER_BOUND('',#4759,.T.);
#3267=FACE_OUTER_BOUND('',#4760,.T.);
#3268=FACE_OUTER_BOUND('',#4761,.T.);
#3269=FACE_OUTER_BOUND('',#4762,.T.);
#3270=FACE_OUTER_BOUND('',#4763,.T.);
#3271=FACE_OUTER_BOUND('',#4764,.T.);
#3272=FACE_OUTER_BOUND('',#4765,.T.);
#3273=FACE_OUTER_BOUND('',#4766,.T.);
#3274=FACE_OUTER_BOUND('',#4767,.T.);
#3275=FACE_OUTER_BOUND('',#4768,.T.);
#3276=FACE_OUTER_BOUND('',#4769,.T.);
#3277=FACE_OUTER_BOUND('',#4770,.T.);
#3278=FACE_OUTER_BOUND('',#4771,.T.);
#3279=FACE_OUTER_BOUND('',#4772,.T.);
#3280=FACE_OUTER_BOUND('',#4773,.T.);
#3281=FACE_OUTER_BOUND('',#4774,.T.);
#3282=FACE_OUTER_BOUND('',#4775,.T.);
#3283=FACE_OUTER_BOUND('',#4776,.T.);
#3284=FACE_OUTER_BOUND('',#4777,.T.);
#3285=FACE_OUTER_BOUND('',#4778,.T.);
#3286=FACE_OUTER_BOUND('',#4779,.T.);
#3287=FACE_OUTER_BOUND('',#4780,.T.);
#3288=FACE_OUTER_BOUND('',#4781,.T.);
#3289=FACE_OUTER_BOUND('',#4782,.T.);
#3290=FACE_OUTER_BOUND('',#4783,.T.);
#3291=FACE_OUTER_BOUND('',#4784,.T.);
#3292=FACE_OUTER_BOUND('',#4785,.T.);
#3293=FACE_OUTER_BOUND('',#4786,.T.);
#3294=FACE_OUTER_BOUND('',#4787,.T.);
#3295=FACE_OUTER_BOUND('',#4788,.T.);
#3296=FACE_OUTER_BOUND('',#4789,.T.);
#3297=FACE_OUTER_BOUND('',#4790,.T.);
#3298=FACE_OUTER_BOUND('',#4791,.T.);
#3299=FACE_OUTER_BOUND('',#4792,.T.);
#3300=FACE_OUTER_BOUND('',#4793,.T.);
#3301=FACE_OUTER_BOUND('',#4794,.T.);
#3302=FACE_OUTER_BOUND('',#4795,.T.);
#3303=FACE_OUTER_BOUND('',#4796,.T.);
#3304=FACE_OUTER_BOUND('',#4797,.T.);
#3305=FACE_OUTER_BOUND('',#4798,.T.);
#3306=FACE_OUTER_BOUND('',#4799,.T.);
#3307=FACE_OUTER_BOUND('',#4800,.T.);
#3308=FACE_OUTER_BOUND('',#4801,.T.);
#3309=FACE_OUTER_BOUND('',#4802,.T.);
#3310=FACE_OUTER_BOUND('',#4803,.T.);
#3311=FACE_OUTER_BOUND('',#4804,.T.);
#3312=FACE_OUTER_BOUND('',#4805,.T.);
#3313=FACE_OUTER_BOUND('',#4806,.T.);
#3314=FACE_OUTER_BOUND('',#4807,.T.);
#3315=FACE_OUTER_BOUND('',#4808,.T.);
#3316=FACE_OUTER_BOUND('',#4809,.T.);
#3317=FACE_OUTER_BOUND('',#4810,.T.);
#3318=FACE_OUTER_BOUND('',#4811,.T.);
#3319=FACE_OUTER_BOUND('',#4812,.T.);
#3320=FACE_OUTER_BOUND('',#4813,.T.);
#3321=FACE_OUTER_BOUND('',#4814,.T.);
#3322=FACE_OUTER_BOUND('',#4815,.T.);
#3323=FACE_OUTER_BOUND('',#4816,.T.);
#3324=FACE_OUTER_BOUND('',#4817,.T.);
#3325=FACE_OUTER_BOUND('',#4818,.T.);
#3326=FACE_OUTER_BOUND('',#4819,.T.);
#3327=FACE_OUTER_BOUND('',#4820,.T.);
#3328=FACE_OUTER_BOUND('',#4821,.T.);
#3329=FACE_OUTER_BOUND('',#4822,.T.);
#3330=FACE_OUTER_BOUND('',#4823,.T.);
#3331=FACE_OUTER_BOUND('',#4824,.T.);
#3332=FACE_OUTER_BOUND('',#4825,.T.);
#3333=FACE_OUTER_BOUND('',#4826,.T.);
#3334=FACE_OUTER_BOUND('',#4827,.T.);
#3335=FACE_OUTER_BOUND('',#4828,.T.);
#3336=FACE_OUTER_BOUND('',#4829,.T.);
#3337=FACE_OUTER_BOUND('',#4830,.T.);
#3338=FACE_OUTER_BOUND('',#4831,.T.);
#3339=FACE_OUTER_BOUND('',#4832,.T.);
#3340=FACE_OUTER_BOUND('',#4833,.T.);
#3341=FACE_OUTER_BOUND('',#4834,.T.);
#3342=FACE_OUTER_BOUND('',#4835,.T.);
#3343=FACE_OUTER_BOUND('',#4836,.T.);
#3344=FACE_OUTER_BOUND('',#4837,.T.);
#3345=FACE_OUTER_BOUND('',#4838,.T.);
#3346=FACE_OUTER_BOUND('',#4839,.T.);
#3347=FACE_OUTER_BOUND('',#4840,.T.);
#3348=FACE_OUTER_BOUND('',#4841,.T.);
#3349=FACE_OUTER_BOUND('',#4842,.T.);
#3350=FACE_OUTER_BOUND('',#4843,.T.);
#3351=FACE_OUTER_BOUND('',#4844,.T.);
#3352=FACE_OUTER_BOUND('',#4845,.T.);
#3353=FACE_OUTER_BOUND('',#4846,.T.);
#3354=FACE_OUTER_BOUND('',#4847,.T.);
#3355=FACE_OUTER_BOUND('',#4848,.T.);
#3356=FACE_OUTER_BOUND('',#4849,.T.);
#3357=FACE_OUTER_BOUND('',#4850,.T.);
#3358=FACE_OUTER_BOUND('',#4851,.T.);
#3359=FACE_OUTER_BOUND('',#4852,.T.);
#3360=FACE_OUTER_BOUND('',#4853,.T.);
#3361=FACE_OUTER_BOUND('',#4854,.T.);
#3362=FACE_OUTER_BOUND('',#4855,.T.);
#3363=FACE_OUTER_BOUND('',#4856,.T.);
#3364=FACE_OUTER_BOUND('',#4857,.T.);
#3365=FACE_OUTER_BOUND('',#4858,.T.);
#3366=FACE_OUTER_BOUND('',#4859,.T.);
#3367=FACE_OUTER_BOUND('',#4860,.T.);
#3368=FACE_OUTER_BOUND('',#4861,.T.);
#3369=FACE_OUTER_BOUND('',#4862,.T.);
#3370=FACE_OUTER_BOUND('',#4863,.T.);
#3371=FACE_OUTER_BOUND('',#4864,.T.);
#3372=FACE_OUTER_BOUND('',#4865,.T.);
#3373=FACE_OUTER_BOUND('',#4866,.T.);
#3374=FACE_OUTER_BOUND('',#4867,.T.);
#3375=FACE_OUTER_BOUND('',#4868,.T.);
#3376=FACE_OUTER_BOUND('',#4869,.T.);
#3377=FACE_OUTER_BOUND('',#4870,.T.);
#3378=FACE_OUTER_BOUND('',#4871,.T.);
#3379=FACE_OUTER_BOUND('',#4872,.T.);
#3380=FACE_OUTER_BOUND('',#4873,.T.);
#3381=FACE_OUTER_BOUND('',#4874,.T.);
#3382=FACE_OUTER_BOUND('',#4875,.T.);
#3383=FACE_OUTER_BOUND('',#4876,.T.);
#3384=FACE_OUTER_BOUND('',#4877,.T.);
#3385=FACE_OUTER_BOUND('',#4878,.T.);
#3386=FACE_OUTER_BOUND('',#4879,.T.);
#3387=FACE_OUTER_BOUND('',#4880,.T.);
#3388=FACE_OUTER_BOUND('',#4881,.T.);
#3389=FACE_OUTER_BOUND('',#4882,.T.);
#3390=FACE_OUTER_BOUND('',#4883,.T.);
#3391=FACE_OUTER_BOUND('',#4884,.T.);
#3392=FACE_OUTER_BOUND('',#4886,.T.);
#3393=FACE_OUTER_BOUND('',#4887,.T.);
#3394=FACE_OUTER_BOUND('',#4888,.T.);
#3395=FACE_OUTER_BOUND('',#4889,.T.);
#3396=FACE_OUTER_BOUND('',#4890,.T.);
#3397=FACE_OUTER_BOUND('',#4892,.T.);
#4645=EDGE_LOOP('',(#19375,#19376,#19377,#19378,#19379,#19380,#19381,#19382));
#4646=EDGE_LOOP('',(#19383,#19384,#19385,#19386));
#4647=EDGE_LOOP('',(#19387,#19388,#19389,#19390));
#4648=EDGE_LOOP('',(#19391,#19392,#19393,#19394));
#4649=EDGE_LOOP('',(#19395,#19396,#19397,#19398));
#4650=EDGE_LOOP('',(#19399,#19400,#19401,#19402));
#4651=EDGE_LOOP('',(#19403,#19404,#19405,#19406));
#4652=EDGE_LOOP('',(#19407,#19408,#19409,#19410));
#4653=EDGE_LOOP('',(#19411,#19412,#19413,#19414));
#4654=EDGE_LOOP('',(#19415,#19416,#19417,#19418));
#4655=EDGE_LOOP('',(#19419,#19420,#19421,#19422));
#4656=EDGE_LOOP('',(#19423,#19424,#19425,#19426));
#4657=EDGE_LOOP('',(#19427,#19428,#19429,#19430));
#4658=EDGE_LOOP('',(#19431,#19432,#19433,#19434));
#4659=EDGE_LOOP('',(#19435,#19436,#19437,#19438));
#4660=EDGE_LOOP('',(#19439,#19440,#19441,#19442));
#4661=EDGE_LOOP('',(#19443,#19444,#19445,#19446));
#4662=EDGE_LOOP('',(#19447,#19448,#19449,#19450));
#4663=EDGE_LOOP('',(#19451,#19452,#19453,#19454));
#4664=EDGE_LOOP('',(#19455,#19456,#19457,#19458));
#4665=EDGE_LOOP('',(#19459,#19460,#19461,#19462));
#4666=EDGE_LOOP('',(#19463,#19464,#19465,#19466));
#4667=EDGE_LOOP('',(#19467,#19468,#19469,#19470));
#4668=EDGE_LOOP('',(#19471,#19472,#19473,#19474));
#4669=EDGE_LOOP('',(#19475,#19476,#19477,#19478));
#4670=EDGE_LOOP('',(#19479,#19480,#19481,#19482));
#4671=EDGE_LOOP('',(#19483,#19484,#19485,#19486));
#4672=EDGE_LOOP('',(#19487,#19488,#19489,#19490));
#4673=EDGE_LOOP('',(#19491,#19492,#19493,#19494));
#4674=EDGE_LOOP('',(#19495,#19496,#19497,#19498));
#4675=EDGE_LOOP('',(#19499,#19500,#19501,#19502));
#4676=EDGE_LOOP('',(#19503,#19504,#19505,#19506));
#4677=EDGE_LOOP('',(#19507,#19508,#19509,#19510));
#4678=EDGE_LOOP('',(#19511,#19512,#19513,#19514));
#4679=EDGE_LOOP('',(#19515,#19516,#19517,#19518));
#4680=EDGE_LOOP('',(#19519,#19520,#19521,#19522));
#4681=EDGE_LOOP('',(#19523,#19524,#19525,#19526));
#4682=EDGE_LOOP('',(#19527,#19528,#19529,#19530));
#4683=EDGE_LOOP('',(#19531,#19532,#19533,#19534));
#4684=EDGE_LOOP('',(#19535,#19536,#19537,#19538));
#4685=EDGE_LOOP('',(#19539,#19540,#19541,#19542));
#4686=EDGE_LOOP('',(#19543,#19544,#19545,#19546));
#4687=EDGE_LOOP('',(#19547,#19548,#19549,#19550));
#4688=EDGE_LOOP('',(#19551,#19552,#19553,#19554));
#4689=EDGE_LOOP('',(#19555,#19556,#19557,#19558));
#4690=EDGE_LOOP('',(#19559,#19560,#19561,#19562));
#4691=EDGE_LOOP('',(#19563,#19564,#19565,#19566));
#4692=EDGE_LOOP('',(#19567,#19568,#19569,#19570));
#4693=EDGE_LOOP('',(#19571,#19572,#19573,#19574));
#4694=EDGE_LOOP('',(#19575,#19576,#19577,#19578));
#4695=EDGE_LOOP('',(#19579,#19580,#19581,#19582));
#4696=EDGE_LOOP('',(#19583,#19584,#19585,#19586));
#4697=EDGE_LOOP('',(#19587,#19588,#19589,#19590));
#4698=EDGE_LOOP('',(#19591,#19592,#19593,#19594));
#4699=EDGE_LOOP('',(#19595,#19596,#19597,#19598));
#4700=EDGE_LOOP('',(#19599,#19600,#19601,#19602));
#4701=EDGE_LOOP('',(#19603,#19604,#19605,#19606));
#4702=EDGE_LOOP('',(#19607,#19608,#19609,#19610));
#4703=EDGE_LOOP('',(#19611,#19612,#19613,#19614));
#4704=EDGE_LOOP('',(#19615,#19616,#19617,#19618));
#4705=EDGE_LOOP('',(#19619,#19620,#19621,#19622));
#4706=EDGE_LOOP('',(#19623,#19624,#19625,#19626));
#4707=EDGE_LOOP('',(#19627,#19628,#19629,#19630));
#4708=EDGE_LOOP('',(#19631,#19632,#19633,#19634));
#4709=EDGE_LOOP('',(#19635,#19636,#19637,#19638));
#4710=EDGE_LOOP('',(#19639,#19640,#19641,#19642));
#4711=EDGE_LOOP('',(#19643,#19644,#19645,#19646));
#4712=EDGE_LOOP('',(#19647,#19648,#19649,#19650));
#4713=EDGE_LOOP('',(#19651,#19652,#19653,#19654));
#4714=EDGE_LOOP('',(#19655,#19656,#19657,#19658));
#4715=EDGE_LOOP('',(#19659,#19660,#19661,#19662));
#4716=EDGE_LOOP('',(#19663,#19664,#19665,#19666));
#4717=EDGE_LOOP('',(#19667,#19668,#19669,#19670));
#4718=EDGE_LOOP('',(#19671,#19672,#19673,#19674));
#4719=EDGE_LOOP('',(#19675,#19676,#19677,#19678));
#4720=EDGE_LOOP('',(#19679,#19680,#19681,#19682));
#4721=EDGE_LOOP('',(#19683,#19684,#19685,#19686));
#4722=EDGE_LOOP('',(#19687,#19688,#19689,#19690));
#4723=EDGE_LOOP('',(#19691,#19692,#19693,#19694));
#4724=EDGE_LOOP('',(#19695,#19696,#19697,#19698));
#4725=EDGE_LOOP('',(#19699,#19700,#19701,#19702));
#4726=EDGE_LOOP('',(#19703,#19704,#19705,#19706));
#4727=EDGE_LOOP('',(#19707,#19708,#19709,#19710));
#4728=EDGE_LOOP('',(#19711,#19712,#19713,#19714));
#4729=EDGE_LOOP('',(#19715,#19716,#19717,#19718));
#4730=EDGE_LOOP('',(#19719,#19720,#19721,#19722));
#4731=EDGE_LOOP('',(#19723,#19724,#19725,#19726));
#4732=EDGE_LOOP('',(#19727,#19728,#19729,#19730));
#4733=EDGE_LOOP('',(#19731,#19732,#19733,#19734));
#4734=EDGE_LOOP('',(#19735,#19736,#19737,#19738));
#4735=EDGE_LOOP('',(#19739,#19740,#19741,#19742));
#4736=EDGE_LOOP('',(#19743,#19744,#19745,#19746));
#4737=EDGE_LOOP('',(#19747,#19748,#19749,#19750));
#4738=EDGE_LOOP('',(#19751,#19752,#19753,#19754));
#4739=EDGE_LOOP('',(#19755,#19756,#19757,#19758));
#4740=EDGE_LOOP('',(#19759,#19760,#19761,#19762));
#4741=EDGE_LOOP('',(#19763,#19764,#19765,#19766));
#4742=EDGE_LOOP('',(#19767,#19768,#19769,#19770));
#4743=EDGE_LOOP('',(#19771,#19772,#19773,#19774));
#4744=EDGE_LOOP('',(#19775,#19776,#19777,#19778));
#4745=EDGE_LOOP('',(#19779,#19780,#19781,#19782));
#4746=EDGE_LOOP('',(#19783,#19784,#19785,#19786));
#4747=EDGE_LOOP('',(#19787,#19788,#19789,#19790));
#4748=EDGE_LOOP('',(#19791,#19792,#19793,#19794));
#4749=EDGE_LOOP('',(#19795,#19796,#19797,#19798));
#4750=EDGE_LOOP('',(#19799,#19800,#19801,#19802));
#4751=EDGE_LOOP('',(#19803,#19804,#19805,#19806));
#4752=EDGE_LOOP('',(#19807,#19808,#19809,#19810));
#4753=EDGE_LOOP('',(#19811,#19812,#19813,#19814));
#4754=EDGE_LOOP('',(#19815,#19816,#19817,#19818));
#4755=EDGE_LOOP('',(#19819,#19820,#19821,#19822));
#4756=EDGE_LOOP('',(#19823,#19824,#19825,#19826));
#4757=EDGE_LOOP('',(#19827,#19828,#19829,#19830));
#4758=EDGE_LOOP('',(#19831,#19832,#19833,#19834));
#4759=EDGE_LOOP('',(#19835,#19836,#19837,#19838));
#4760=EDGE_LOOP('',(#19839,#19840,#19841,#19842));
#4761=EDGE_LOOP('',(#19843,#19844,#19845,#19846));
#4762=EDGE_LOOP('',(#19847,#19848,#19849,#19850,#19851));
#4763=EDGE_LOOP('',(#19852,#19853,#19854,#19855,#19856,#19857,#19858,#19859,
#19860,#19861,#19862,#19863,#19864,#19865,#19866,#19867,#19868,#19869,#19870,
#19871,#19872,#19873,#19874,#19875,#19876,#19877,#19878,#19879,#19880,#19881,
#19882,#19883,#19884,#19885,#19886,#19887,#19888,#19889,#19890,#19891,#19892,
#19893,#19894,#19895,#19896,#19897,#19898,#19899,#19900,#19901,#19902,#19903,
#19904,#19905,#19906,#19907,#19908,#19909,#19910,#19911,#19912,#19913,#19914,
#19915,#19916,#19917,#19918,#19919,#19920,#19921,#19922,#19923,#19924,#19925,
#19926,#19927,#19928,#19929,#19930,#19931,#19932,#19933,#19934,#19935,#19936,
#19937,#19938,#19939,#19940,#19941,#19942,#19943,#19944,#19945,#19946,#19947,
#19948,#19949,#19950,#19951,#19952,#19953,#19954,#19955,#19956,#19957,#19958,
#19959,#19960,#19961,#19962,#19963,#19964,#19965,#19966,#19967,#19968,#19969,
#19970,#19971,#19972));
#4764=EDGE_LOOP('',(#19973,#19974,#19975,#19976,#19977));
#4765=EDGE_LOOP('',(#19978,#19979,#19980,#19981));
#4766=EDGE_LOOP('',(#19982,#19983,#19984,#19985,#19986,#19987,#19988,#19989,
#19990,#19991,#19992,#19993,#19994,#19995,#19996,#19997,#19998,#19999,#20000,
#20001,#20002,#20003,#20004,#20005,#20006,#20007,#20008,#20009,#20010,#20011,
#20012,#20013,#20014,#20015,#20016,#20017,#20018,#20019,#20020,#20021,#20022,
#20023,#20024,#20025,#20026,#20027,#20028,#20029,#20030,#20031,#20032,#20033,
#20034,#20035,#20036,#20037,#20038,#20039,#20040,#20041,#20042,#20043,#20044,
#20045,#20046,#20047,#20048,#20049,#20050,#20051,#20052,#20053,#20054,#20055,
#20056,#20057,#20058,#20059,#20060,#20061,#20062,#20063,#20064,#20065,#20066,
#20067,#20068,#20069,#20070,#20071,#20072,#20073,#20074,#20075,#20076,#20077,
#20078,#20079,#20080,#20081,#20082,#20083,#20084,#20085,#20086,#20087,#20088,
#20089,#20090,#20091,#20092,#20093,#20094,#20095,#20096,#20097,#20098,#20099,
#20100,#20101,#20102));
#4767=EDGE_LOOP('',(#20103,#20104,#20105));
#4768=EDGE_LOOP('',(#20106,#20107,#20108,#20109));
#4769=EDGE_LOOP('',(#20110,#20111,#20112,#20113));
#4770=EDGE_LOOP('',(#20114,#20115,#20116));
#4771=EDGE_LOOP('',(#20117,#20118,#20119,#20120));
#4772=EDGE_LOOP('',(#20121,#20122,#20123,#20124));
#4773=EDGE_LOOP('',(#20125,#20126,#20127));
#4774=EDGE_LOOP('',(#20128,#20129,#20130,#20131));
#4775=EDGE_LOOP('',(#20132,#20133,#20134,#20135));
#4776=EDGE_LOOP('',(#20136,#20137,#20138));
#4777=EDGE_LOOP('',(#20139,#20140,#20141,#20142));
#4778=EDGE_LOOP('',(#20143,#20144,#20145,#20146));
#4779=EDGE_LOOP('',(#20147,#20148,#20149));
#4780=EDGE_LOOP('',(#20150,#20151,#20152,#20153));
#4781=EDGE_LOOP('',(#20154,#20155,#20156,#20157));
#4782=EDGE_LOOP('',(#20158,#20159,#20160));
#4783=EDGE_LOOP('',(#20161,#20162,#20163,#20164));
#4784=EDGE_LOOP('',(#20165,#20166,#20167,#20168));
#4785=EDGE_LOOP('',(#20169,#20170,#20171));
#4786=EDGE_LOOP('',(#20172,#20173,#20174,#20175));
#4787=EDGE_LOOP('',(#20176,#20177,#20178,#20179));
#4788=EDGE_LOOP('',(#20180,#20181,#20182));
#4789=EDGE_LOOP('',(#20183,#20184,#20185,#20186));
#4790=EDGE_LOOP('',(#20187,#20188,#20189,#20190));
#4791=EDGE_LOOP('',(#20191,#20192,#20193));
#4792=EDGE_LOOP('',(#20194,#20195,#20196,#20197));
#4793=EDGE_LOOP('',(#20198,#20199,#20200,#20201));
#4794=EDGE_LOOP('',(#20202,#20203,#20204));
#4795=EDGE_LOOP('',(#20205,#20206,#20207,#20208));
#4796=EDGE_LOOP('',(#20209,#20210,#20211,#20212));
#4797=EDGE_LOOP('',(#20213,#20214,#20215));
#4798=EDGE_LOOP('',(#20216,#20217,#20218,#20219));
#4799=EDGE_LOOP('',(#20220,#20221,#20222,#20223));
#4800=EDGE_LOOP('',(#20224,#20225,#20226));
#4801=EDGE_LOOP('',(#20227,#20228,#20229,#20230));
#4802=EDGE_LOOP('',(#20231,#20232,#20233,#20234));
#4803=EDGE_LOOP('',(#20235,#20236,#20237));
#4804=EDGE_LOOP('',(#20238,#20239,#20240,#20241));
#4805=EDGE_LOOP('',(#20242,#20243,#20244,#20245));
#4806=EDGE_LOOP('',(#20246,#20247,#20248));
#4807=EDGE_LOOP('',(#20249,#20250,#20251,#20252));
#4808=EDGE_LOOP('',(#20253,#20254,#20255,#20256));
#4809=EDGE_LOOP('',(#20257,#20258,#20259));
#4810=EDGE_LOOP('',(#20260,#20261,#20262,#20263));
#4811=EDGE_LOOP('',(#20264,#20265,#20266,#20267));
#4812=EDGE_LOOP('',(#20268,#20269,#20270));
#4813=EDGE_LOOP('',(#20271,#20272,#20273,#20274));
#4814=EDGE_LOOP('',(#20275,#20276,#20277,#20278));
#4815=EDGE_LOOP('',(#20279,#20280,#20281));
#4816=EDGE_LOOP('',(#20282,#20283,#20284,#20285));
#4817=EDGE_LOOP('',(#20286,#20287,#20288,#20289));
#4818=EDGE_LOOP('',(#20290,#20291,#20292,#20293));
#4819=EDGE_LOOP('',(#20294,#20295,#20296,#20297));
#4820=EDGE_LOOP('',(#20298,#20299,#20300,#20301));
#4821=EDGE_LOOP('',(#20302,#20303,#20304));
#4822=EDGE_LOOP('',(#20305,#20306,#20307,#20308));
#4823=EDGE_LOOP('',(#20309,#20310,#20311,#20312));
#4824=EDGE_LOOP('',(#20313,#20314,#20315));
#4825=EDGE_LOOP('',(#20316,#20317,#20318,#20319));
#4826=EDGE_LOOP('',(#20320,#20321,#20322,#20323));
#4827=EDGE_LOOP('',(#20324,#20325,#20326));
#4828=EDGE_LOOP('',(#20327,#20328,#20329,#20330));
#4829=EDGE_LOOP('',(#20331,#20332,#20333,#20334));
#4830=EDGE_LOOP('',(#20335,#20336,#20337));
#4831=EDGE_LOOP('',(#20338,#20339,#20340,#20341));
#4832=EDGE_LOOP('',(#20342,#20343,#20344,#20345));
#4833=EDGE_LOOP('',(#20346,#20347,#20348));
#4834=EDGE_LOOP('',(#20349,#20350,#20351,#20352));
#4835=EDGE_LOOP('',(#20353,#20354,#20355,#20356));
#4836=EDGE_LOOP('',(#20357,#20358,#20359));
#4837=EDGE_LOOP('',(#20360,#20361,#20362,#20363));
#4838=EDGE_LOOP('',(#20364,#20365,#20366,#20367));
#4839=EDGE_LOOP('',(#20368,#20369,#20370));
#4840=EDGE_LOOP('',(#20371,#20372,#20373,#20374));
#4841=EDGE_LOOP('',(#20375,#20376,#20377,#20378));
#4842=EDGE_LOOP('',(#20379,#20380,#20381));
#4843=EDGE_LOOP('',(#20382,#20383,#20384,#20385));
#4844=EDGE_LOOP('',(#20386,#20387,#20388,#20389));
#4845=EDGE_LOOP('',(#20390,#20391,#20392));
#4846=EDGE_LOOP('',(#20393,#20394,#20395,#20396));
#4847=EDGE_LOOP('',(#20397,#20398,#20399,#20400));
#4848=EDGE_LOOP('',(#20401,#20402,#20403));
#4849=EDGE_LOOP('',(#20404,#20405,#20406,#20407));
#4850=EDGE_LOOP('',(#20408,#20409,#20410,#20411));
#4851=EDGE_LOOP('',(#20412,#20413,#20414));
#4852=EDGE_LOOP('',(#20415,#20416,#20417,#20418));
#4853=EDGE_LOOP('',(#20419,#20420,#20421,#20422));
#4854=EDGE_LOOP('',(#20423,#20424,#20425));
#4855=EDGE_LOOP('',(#20426,#20427,#20428,#20429));
#4856=EDGE_LOOP('',(#20430,#20431,#20432,#20433));
#4857=EDGE_LOOP('',(#20434,#20435,#20436));
#4858=EDGE_LOOP('',(#20437,#20438,#20439,#20440));
#4859=EDGE_LOOP('',(#20441,#20442,#20443,#20444));
#4860=EDGE_LOOP('',(#20445,#20446,#20447));
#4861=EDGE_LOOP('',(#20448,#20449,#20450,#20451));
#4862=EDGE_LOOP('',(#20452,#20453,#20454,#20455));
#4863=EDGE_LOOP('',(#20456,#20457,#20458));
#4864=EDGE_LOOP('',(#20459,#20460,#20461,#20462));
#4865=EDGE_LOOP('',(#20463,#20464,#20465,#20466));
#4866=EDGE_LOOP('',(#20467,#20468,#20469));
#4867=EDGE_LOOP('',(#20470,#20471,#20472,#20473));
#4868=EDGE_LOOP('',(#20474,#20475,#20476,#20477));
#4869=EDGE_LOOP('',(#20478,#20479,#20480));
#4870=EDGE_LOOP('',(#20481,#20482,#20483,#20484));
#4871=EDGE_LOOP('',(#20485,#20486,#20487,#20488));
#4872=EDGE_LOOP('',(#20489,#20490,#20491,#20492,#20493,#20494,#20495,#20496,
#20497,#20498,#20499,#20500,#20501,#20502,#20503,#20504,#20505,#20506,#20507,
#20508,#20509,#20510,#20511,#20512,#20513,#20514,#20515,#20516,#20517,#20518,
#20519,#20520,#20521,#20522,#20523,#20524,#20525,#20526,#20527,#20528,#20529,
#20530,#20531,#20532,#20533,#20534,#20535,#20536,#20537,#20538,#20539,#20540,
#20541,#20542,#20543,#20544,#20545,#20546,#20547,#20548,#20549,#20550,#20551,
#20552,#20553,#20554,#20555,#20556,#20557,#20558,#20559,#20560,#20561,#20562,
#20563,#20564,#20565,#20566,#20567,#20568,#20569,#20570,#20571,#20572,#20573,
#20574,#20575,#20576,#20577,#20578,#20579,#20580,#20581,#20582,#20583,#20584,
#20585,#20586,#20587,#20588,#20589,#20590,#20591,#20592,#20593,#20594,#20595,
#20596,#20597,#20598,#20599,#20600,#20601,#20602,#20603,#20604,#20605,#20606,
#20607,#20608,#20609,#20610,#20611,#20612,#20613,#20614,#20615,#20616,#20617,
#20618,#20619,#20620,#20621,#20622,#20623,#20624,#20625,#20626,#20627,#20628,
#20629,#20630,#20631,#20632,#20633,#20634,#20635,#20636));
#4873=EDGE_LOOP('',(#20637,#20638,#20639,#20640));
#4874=EDGE_LOOP('',(#20641,#20642,#20643,#20644));
#4875=EDGE_LOOP('',(#20645,#20646,#20647));
#4876=EDGE_LOOP('',(#20648,#20649,#20650,#20651,#20652,#20653,#20654,#20655,
#20656,#20657,#20658,#20659,#20660,#20661,#20662,#20663,#20664,#20665,#20666,
#20667,#20668,#20669,#20670,#20671,#20672,#20673,#20674,#20675,#20676,#20677,
#20678,#20679,#20680,#20681,#20682,#20683,#20684,#20685,#20686,#20687,#20688,
#20689,#20690,#20691,#20692,#20693,#20694,#20695,#20696,#20697,#20698,#20699,
#20700,#20701,#20702,#20703,#20704,#20705,#20706,#20707,#20708,#20709,#20710,
#20711,#20712,#20713,#20714,#20715,#20716,#20717,#20718,#20719,#20720,#20721,
#20722,#20723,#20724,#20725,#20726,#20727,#20728,#20729,#20730,#20731,#20732,
#20733,#20734,#20735,#20736,#20737,#20738,#20739,#20740,#20741,#20742,#20743,
#20744,#20745,#20746,#20747,#20748,#20749,#20750,#20751,#20752,#20753,#20754,
#20755,#20756,#20757,#20758));
#4877=EDGE_LOOP('',(#20759,#20760,#20761));
#4878=EDGE_LOOP('',(#20762,#20763,#20764,#20765));
#4879=EDGE_LOOP('',(#20766,#20767,#20768,#20769));
#4880=EDGE_LOOP('',(#20770,#20771,#20772,#20773));
#4881=EDGE_LOOP('',(#20774,#20775,#20776,#20777));
#4882=EDGE_LOOP('',(#20778,#20779,#20780,#20781));
#4883=EDGE_LOOP('',(#20782,#20783,#20784,#20785));
#4884=EDGE_LOOP('',(#20786,#20787,#20788,#20789,#20790,#20791));
#4885=EDGE_LOOP('',(#20792));
#4886=EDGE_LOOP('',(#20793));
#4887=EDGE_LOOP('',(#20794,#20795,#20796,#20797));
#4888=EDGE_LOOP('',(#20798,#20799,#20800,#20801));
#4889=EDGE_LOOP('',(#20802,#20803,#20804,#20805,#20806,#20807));
#4890=EDGE_LOOP('',(#20808));
#4891=EDGE_LOOP('',(#20809));
#4892=EDGE_LOOP('',(#20810));
#4893=EDGE_LOOP('',(#20811,#20812,#20813,#20814,#20815,#20816));
#5680=CIRCLE('',#25040,0.14635);
#5681=CIRCLE('',#25041,0.14635);
#5682=CIRCLE('',#25042,0.14635);
#5683=CIRCLE('',#25101,0.117775);
#5684=CIRCLE('',#25161,0.14635);
#5685=CIRCLE('',#25162,0.14635);
#5686=CIRCLE('',#25164,0.117775);
#5687=CIRCLE('',#25167,0.275);
#5688=CIRCLE('',#25171,0.275);
#5689=CIRCLE('',#25175,0.275);
#5690=CIRCLE('',#25179,0.275);
#5691=CIRCLE('',#25183,0.275);
#5692=CIRCLE('',#25187,0.275);
#5693=CIRCLE('',#25191,0.275);
#5694=CIRCLE('',#25195,0.275);
#5695=CIRCLE('',#25199,0.275);
#5696=CIRCLE('',#25203,0.275);
#5697=CIRCLE('',#25207,0.275);
#5698=CIRCLE('',#25211,0.275);
#5699=CIRCLE('',#25215,0.275);
#5700=CIRCLE('',#25219,0.275);
#5701=CIRCLE('',#25223,0.275);
#5702=CIRCLE('',#25227,0.275);
#5703=CIRCLE('',#25231,0.275);
#5704=CIRCLE('',#25235,0.275);
#5705=CIRCLE('',#25236,0.275);
#5706=CIRCLE('',#25240,0.275);
#5707=CIRCLE('',#25244,0.275);
#5708=CIRCLE('',#25248,0.275);
#5709=CIRCLE('',#25252,0.275);
#5710=CIRCLE('',#25256,0.275);
#5711=CIRCLE('',#25260,0.275);
#5712=CIRCLE('',#25264,0.275);
#5713=CIRCLE('',#25268,0.275);
#5714=CIRCLE('',#25272,0.275);
#5715=CIRCLE('',#25276,0.275);
#5716=CIRCLE('',#25280,0.275);
#5717=CIRCLE('',#25284,0.275);
#5718=CIRCLE('',#25288,0.275);
#5719=CIRCLE('',#25292,0.275);
#5720=CIRCLE('',#25296,0.275);
#5721=CIRCLE('',#25300,0.275);
#5722=CIRCLE('',#25304,0.275);
#5723=CIRCLE('',#25308,0.275);
#5724=CIRCLE('',#25309,0.275);
#5725=CIRCLE('',#25310,0.275);
#5726=CIRCLE('',#25311,0.275);
#5727=CIRCLE('',#25312,0.275);
#5728=CIRCLE('',#25313,0.275);
#5729=CIRCLE('',#25314,0.275);
#5730=CIRCLE('',#25315,0.275);
#5731=CIRCLE('',#25316,0.275);
#5732=CIRCLE('',#25317,0.275);
#5733=CIRCLE('',#25318,0.275);
#5734=CIRCLE('',#25319,0.275);
#5735=CIRCLE('',#25320,0.275);
#5736=CIRCLE('',#25321,0.275);
#5737=CIRCLE('',#25322,0.275);
#5738=CIRCLE('',#25323,0.275);
#5739=CIRCLE('',#25324,0.275);
#5740=CIRCLE('',#25325,0.275);
#5741=CIRCLE('',#25326,0.275);
#5742=CIRCLE('',#25327,0.275);
#5743=CIRCLE('',#25328,0.275);
#5744=CIRCLE('',#25329,0.275);
#5745=CIRCLE('',#25330,0.275);
#5746=CIRCLE('',#25331,0.275);
#5747=CIRCLE('',#25332,0.275);
#5748=CIRCLE('',#25333,0.275);
#5749=CIRCLE('',#25334,0.275);
#5750=CIRCLE('',#25335,0.275);
#5751=CIRCLE('',#25336,0.275);
#5752=CIRCLE('',#25337,0.275);
#5753=CIRCLE('',#25338,0.275);
#5754=CIRCLE('',#25339,0.275);
#5755=CIRCLE('',#25340,0.275);
#5756=CIRCLE('',#25341,0.275);
#5757=CIRCLE('',#25342,0.275);
#5758=CIRCLE('',#25343,0.275);
#5759=CIRCLE('',#25344,0.275);
#5760=CIRCLE('',#25345,0.275);
#5761=CIRCLE('',#25350,0.26);
#5762=CIRCLE('',#25352,0.113891921086774);
#5763=CIRCLE('',#25361,0.114);
#5764=CIRCLE('',#25364,0.14635);
#5765=CIRCLE('',#25366,0.16);
#7135=LINE('',#41665,#8980);
#7136=LINE('',#41686,#8981);
#7137=LINE('',#41706,#8982);
#7138=LINE('',#41754,#8983);
#7139=LINE('',#41808,#8984);
#7140=LINE('',#41856,#8985);
#7141=LINE('',#41904,#8986);
#7142=LINE('',#41958,#8987);
#7143=LINE('',#42006,#8988);
#7144=LINE('',#42054,#8989);
#7145=LINE('',#42102,#8990);
#7146=LINE('',#42156,#8991);
#7147=LINE('',#42204,#8992);
#7148=LINE('',#42252,#8993);
#7149=LINE('',#42306,#8994);
#7150=LINE('',#42354,#8995);
#7151=LINE('',#42402,#8996);
#7152=LINE('',#42453,#8997);
#7153=LINE('',#42504,#8998);
#7154=LINE('',#42552,#8999);
#7155=LINE('',#42600,#9000);
#7156=LINE('',#42654,#9001);
#7157=LINE('',#42702,#9002);
#7158=LINE('',#42750,#9003);
#7159=LINE('',#42804,#9004);
#7160=LINE('',#42852,#9005);
#7161=LINE('',#42900,#9006);
#7162=LINE('',#42948,#9007);
#7163=LINE('',#43002,#9008);
#7164=LINE('',#43050,#9009);
#7165=LINE('',#43098,#9010);
#7166=LINE('',#43152,#9011);
#7167=LINE('',#43200,#9012);
#7168=LINE('',#43248,#9013);
#7169=LINE('',#43296,#9014);
#7170=LINE('',#43350,#9015);
#7171=LINE('',#43398,#9016);
#7172=LINE('',#43446,#9017);
#7173=LINE('',#43500,#9018);
#7174=LINE('',#43548,#9019);
#7175=LINE('',#43596,#9020);
#7176=LINE('',#43647,#9021);
#7177=LINE('',#43698,#9022);
#7178=LINE('',#43746,#9023);
#7179=LINE('',#43794,#9024);
#7180=LINE('',#43848,#9025);
#7181=LINE('',#43896,#9026);
#7182=LINE('',#43944,#9027);
#7183=LINE('',#43998,#9028);
#7184=LINE('',#44046,#9029);
#7185=LINE('',#44094,#9030);
#7186=LINE('',#44142,#9031);
#7187=LINE('',#44196,#9032);
#7188=LINE('',#44244,#9033);
#7189=LINE('',#44292,#9034);
#7190=LINE('',#44346,#9035);
#7191=LINE('',#44394,#9036);
#7192=LINE('',#44442,#9037);
#7193=LINE('',#44490,#9038);
#7194=LINE('',#44544,#9039);
#7195=LINE('',#44562,#9040);
#7196=LINE('',#44587,#9041);
#7197=LINE('',#44612,#9042);
#7198=LINE('',#44636,#9043);
#7199=LINE('',#44660,#9044);
#7200=LINE('',#44685,#9045);
#7201=LINE('',#44710,#9046);
#7202=LINE('',#44734,#9047);
#7203=LINE('',#44759,#9048);
#7204=LINE('',#44784,#9049);
#7205=LINE('',#44808,#9050);
#7206=LINE('',#44832,#9051);
#7207=LINE('',#44857,#9052);
#7208=LINE('',#44882,#9053);
#7209=LINE('',#44906,#9054);
#7210=LINE('',#44931,#9055);
#7211=LINE('',#44956,#9056);
#7212=LINE('',#44980,#9057);
#7213=LINE('',#45005,#9058);
#7214=LINE('',#45029,#9059);
#7215=LINE('',#45054,#9060);
#7216=LINE('',#45078,#9061);
#7217=LINE('',#45103,#9062);
#7218=LINE('',#45128,#9063);
#7219=LINE('',#45152,#9064);
#7220=LINE('',#45177,#9065);
#7221=LINE('',#45202,#9066);
#7222=LINE('',#45226,#9067);
#7223=LINE('',#45250,#9068);
#7224=LINE('',#45275,#9069);
#7225=LINE('',#45300,#9070);
#7226=LINE('',#45324,#9071);
#7227=LINE('',#45349,#9072);
#7228=LINE('',#45374,#9073);
#7229=LINE('',#45398,#9074);
#7230=LINE('',#45422,#9075);
#7231=LINE('',#45447,#9076);
#7232=LINE('',#45472,#9077);
#7233=LINE('',#45496,#9078);
#7234=LINE('',#45521,#9079);
#7235=LINE('',#45546,#9080);
#7236=LINE('',#45570,#9081);
#7237=LINE('',#45595,#9082);
#7238=LINE('',#45619,#9083);
#7239=LINE('',#45644,#9084);
#7240=LINE('',#45668,#9085);
#7241=LINE('',#45693,#9086);
#7242=LINE('',#45718,#9087);
#7243=LINE('',#45742,#9088);
#7244=LINE('',#45767,#9089);
#7245=LINE('',#45792,#9090);
#7246=LINE('',#45816,#9091);
#7247=LINE('',#45840,#9092);
#7248=LINE('',#45865,#9093);
#7249=LINE('',#45890,#9094);
#7250=LINE('',#45914,#9095);
#7251=LINE('',#45939,#9096);
#7252=LINE('',#45964,#9097);
#7253=LINE('',#49237,#9098);
#7254=LINE('',#49238,#9099);
#7255=LINE('',#49241,#9100);
#7256=LINE('',#49243,#9101);
#7257=LINE('',#49249,#9102);
#7258=LINE('',#49258,#9103);
#7259=LINE('',#49259,#9104);
#7260=LINE('',#49262,#9105);
#7261=LINE('',#49264,#9106);
#7262=LINE('',#49270,#9107);
#7263=LINE('',#49279,#9108);
#7264=LINE('',#49280,#9109);
#7265=LINE('',#49283,#9110);
#7266=LINE('',#49285,#9111);
#7267=LINE('',#49291,#9112);
#7268=LINE('',#49300,#9113);
#7269=LINE('',#49301,#9114);
#7270=LINE('',#49304,#9115);
#7271=LINE('',#49306,#9116);
#7272=LINE('',#49312,#9117);
#7273=LINE('',#49321,#9118);
#7274=LINE('',#49322,#9119);
#7275=LINE('',#49325,#9120);
#7276=LINE('',#49327,#9121);
#7277=LINE('',#49333,#9122);
#7278=LINE('',#49342,#9123);
#7279=LINE('',#49343,#9124);
#7280=LINE('',#49346,#9125);
#7281=LINE('',#49348,#9126);
#7282=LINE('',#49354,#9127);
#7283=LINE('',#49363,#9128);
#7284=LINE('',#49364,#9129);
#7285=LINE('',#49367,#9130);
#7286=LINE('',#49369,#9131);
#7287=LINE('',#49375,#9132);
#7288=LINE('',#49384,#9133);
#7289=LINE('',#49385,#9134);
#7290=LINE('',#49388,#9135);
#7291=LINE('',#49390,#9136);
#7292=LINE('',#49396,#9137);
#7293=LINE('',#49405,#9138);
#7294=LINE('',#49406,#9139);
#7295=LINE('',#49409,#9140);
#7296=LINE('',#49411,#9141);
#7297=LINE('',#49417,#9142);
#7298=LINE('',#49426,#9143);
#7299=LINE('',#49427,#9144);
#7300=LINE('',#49430,#9145);
#7301=LINE('',#49432,#9146);
#7302=LINE('',#49438,#9147);
#7303=LINE('',#49447,#9148);
#7304=LINE('',#49448,#9149);
#7305=LINE('',#49451,#9150);
#7306=LINE('',#49453,#9151);
#7307=LINE('',#49459,#9152);
#7308=LINE('',#49468,#9153);
#7309=LINE('',#49469,#9154);
#7310=LINE('',#49472,#9155);
#7311=LINE('',#49474,#9156);
#7312=LINE('',#49480,#9157);
#7313=LINE('',#49489,#9158);
#7314=LINE('',#49490,#9159);
#7315=LINE('',#49493,#9160);
#7316=LINE('',#49495,#9161);
#7317=LINE('',#49501,#9162);
#7318=LINE('',#49510,#9163);
#7319=LINE('',#49511,#9164);
#7320=LINE('',#49514,#9165);
#7321=LINE('',#49516,#9166);
#7322=LINE('',#49522,#9167);
#7323=LINE('',#49531,#9168);
#7324=LINE('',#49532,#9169);
#7325=LINE('',#49535,#9170);
#7326=LINE('',#49537,#9171);
#7327=LINE('',#49543,#9172);
#7328=LINE('',#49552,#9173);
#7329=LINE('',#49553,#9174);
#7330=LINE('',#49556,#9175);
#7331=LINE('',#49558,#9176);
#7332=LINE('',#49564,#9177);
#7333=LINE('',#49573,#9178);
#7334=LINE('',#49574,#9179);
#7335=LINE('',#49577,#9180);
#7336=LINE('',#49579,#9181);
#7337=LINE('',#49585,#9182);
#7338=LINE('',#49594,#9183);
#7339=LINE('',#49596,#9184);
#7340=LINE('',#49600,#9185);
#7341=LINE('',#49602,#9186);
#7342=LINE('',#49608,#9187);
#7343=LINE('',#49617,#9188);
#7344=LINE('',#49618,#9189);
#7345=LINE('',#49621,#9190);
#7346=LINE('',#49623,#9191);
#7347=LINE('',#49629,#9192);
#7348=LINE('',#49638,#9193);
#7349=LINE('',#49639,#9194);
#7350=LINE('',#49642,#9195);
#7351=LINE('',#49644,#9196);
#7352=LINE('',#49650,#9197);
#7353=LINE('',#49659,#9198);
#7354=LINE('',#49660,#9199);
#7355=LINE('',#49663,#9200);
#7356=LINE('',#49665,#9201);
#7357=LINE('',#49671,#9202);
#7358=LINE('',#49680,#9203);
#7359=LINE('',#49681,#9204);
#7360=LINE('',#49684,#9205);
#7361=LINE('',#49686,#9206);
#7362=LINE('',#49692,#9207);
#7363=LINE('',#49701,#9208);
#7364=LINE('',#49702,#9209);
#7365=LINE('',#49705,#9210);
#7366=LINE('',#49707,#9211);
#7367=LINE('',#49713,#9212);
#7368=LINE('',#49722,#9213);
#7369=LINE('',#49723,#9214);
#7370=LINE('',#49726,#9215);
#7371=LINE('',#49728,#9216);
#7372=LINE('',#49734,#9217);
#7373=LINE('',#49743,#9218);
#7374=LINE('',#49744,#9219);
#7375=LINE('',#49747,#9220);
#7376=LINE('',#49749,#9221);
#7377=LINE('',#49755,#9222);
#7378=LINE('',#49764,#9223);
#7379=LINE('',#49765,#9224);
#7380=LINE('',#49768,#9225);
#7381=LINE('',#49770,#9226);
#7382=LINE('',#49776,#9227);
#7383=LINE('',#49785,#9228);
#7384=LINE('',#49786,#9229);
#7385=LINE('',#49789,#9230);
#7386=LINE('',#49791,#9231);
#7387=LINE('',#49797,#9232);
#7388=LINE('',#49806,#9233);
#7389=LINE('',#49807,#9234);
#7390=LINE('',#49810,#9235);
#7391=LINE('',#49812,#9236);
#7392=LINE('',#49818,#9237);
#7393=LINE('',#49827,#9238);
#7394=LINE('',#49828,#9239);
#7395=LINE('',#49831,#9240);
#7396=LINE('',#49833,#9241);
#7397=LINE('',#49839,#9242);
#7398=LINE('',#49848,#9243);
#7399=LINE('',#49849,#9244);
#7400=LINE('',#49852,#9245);
#7401=LINE('',#49854,#9246);
#7402=LINE('',#49860,#9247);
#7403=LINE('',#49869,#9248);
#7404=LINE('',#49870,#9249);
#7405=LINE('',#49873,#9250);
#7406=LINE('',#49875,#9251);
#7407=LINE('',#49881,#9252);
#7408=LINE('',#49890,#9253);
#7409=LINE('',#49891,#9254);
#7410=LINE('',#49894,#9255);
#7411=LINE('',#49896,#9256);
#7412=LINE('',#49902,#9257);
#7413=LINE('',#49911,#9258);
#7414=LINE('',#49912,#9259);
#7415=LINE('',#49915,#9260);
#7416=LINE('',#49917,#9261);
#7417=LINE('',#49923,#9262);
#7418=LINE('',#49932,#9263);
#7419=LINE('',#49933,#9264);
#7420=LINE('',#49936,#9265);
#7421=LINE('',#49938,#9266);
#7422=LINE('',#49944,#9267);
#7423=LINE('',#49953,#9268);
#7424=LINE('',#49954,#9269);
#7425=LINE('',#49957,#9270);
#7426=LINE('',#49959,#9271);
#7427=LINE('',#49965,#9272);
#7428=LINE('',#49988,#9273);
#7429=LINE('',#50010,#9274);
#7430=LINE('',#50014,#9275);
#7431=LINE('',#50018,#9276);
#7432=LINE('',#50020,#9277);
#7433=LINE('',#50028,#9278);
#7434=LINE('',#50033,#9279);
#7435=LINE('',#50037,#9280);
#7436=LINE('',#50042,#9281);
#7437=LINE('',#50044,#9282);
#7438=LINE('',#50046,#9283);
#7439=LINE('',#50047,#9284);
#7440=LINE('',#50050,#9285);
#7441=LINE('',#50052,#9286);
#7442=LINE('',#50053,#9287);
#7443=LINE('',#50056,#9288);
#7444=LINE('',#50058,#9289);
#7445=LINE('',#50059,#9290);
#7446=LINE('',#50062,#9291);
#7447=LINE('',#50064,#9292);
#7448=LINE('',#50065,#9293);
#7449=LINE('',#50068,#9294);
#7450=LINE('',#50070,#9295);
#7451=LINE('',#50071,#9296);
#7452=LINE('',#50073,#9297);
#7453=LINE('',#50074,#9298);
#7454=LINE('',#50080,#9299);
#7455=LINE('',#50086,#9300);
#8980=VECTOR('',#30025,0.15);
#8981=VECTOR('',#30028,0.15);
#8982=VECTOR('',#30035,0.15);
#8983=VECTOR('',#30038,0.15);
#8984=VECTOR('',#30041,0.15);
#8985=VECTOR('',#30044,0.15);
#8986=VECTOR('',#30047,0.15);
#8987=VECTOR('',#30050,0.15);
#8988=VECTOR('',#30053,0.15);
#8989=VECTOR('',#30056,0.15);
#8990=VECTOR('',#30059,0.15);
#8991=VECTOR('',#30062,0.15);
#8992=VECTOR('',#30065,0.15);
#8993=VECTOR('',#30068,0.15);
#8994=VECTOR('',#30071,0.15);
#8995=VECTOR('',#30074,0.15);
#8996=VECTOR('',#30077,0.15);
#8997=VECTOR('',#30080,0.15);
#8998=VECTOR('',#30083,0.15);
#8999=VECTOR('',#30086,0.15);
#9000=VECTOR('',#30089,0.15);
#9001=VECTOR('',#30092,0.15);
#9002=VECTOR('',#30095,0.15);
#9003=VECTOR('',#30098,0.15);
#9004=VECTOR('',#30101,0.15);
#9005=VECTOR('',#30104,0.15);
#9006=VECTOR('',#30107,0.15);
#9007=VECTOR('',#30110,0.15);
#9008=VECTOR('',#30113,0.15);
#9009=VECTOR('',#30116,0.15);
#9010=VECTOR('',#30119,0.15);
#9011=VECTOR('',#30122,0.15);
#9012=VECTOR('',#30125,0.15);
#9013=VECTOR('',#30128,0.15);
#9014=VECTOR('',#30131,0.15);
#9015=VECTOR('',#30134,0.15);
#9016=VECTOR('',#30137,0.15);
#9017=VECTOR('',#30140,0.15);
#9018=VECTOR('',#30143,0.15);
#9019=VECTOR('',#30146,0.15);
#9020=VECTOR('',#30149,0.15);
#9021=VECTOR('',#30152,0.15);
#9022=VECTOR('',#30155,0.15);
#9023=VECTOR('',#30158,0.15);
#9024=VECTOR('',#30161,0.15);
#9025=VECTOR('',#30164,0.15);
#9026=VECTOR('',#30167,0.15);
#9027=VECTOR('',#30170,0.15);
#9028=VECTOR('',#30173,0.15);
#9029=VECTOR('',#30176,0.15);
#9030=VECTOR('',#30179,0.15);
#9031=VECTOR('',#30182,0.15);
#9032=VECTOR('',#30185,0.15);
#9033=VECTOR('',#30188,0.15);
#9034=VECTOR('',#30191,0.15);
#9035=VECTOR('',#30194,0.15);
#9036=VECTOR('',#30197,0.15);
#9037=VECTOR('',#30200,0.15);
#9038=VECTOR('',#30203,0.15);
#9039=VECTOR('',#30206,0.117775);
#9040=VECTOR('',#30211,0.117775);
#9041=VECTOR('',#30214,0.117775);
#9042=VECTOR('',#30217,0.117775);
#9043=VECTOR('',#30220,0.117775);
#9044=VECTOR('',#30223,0.117775);
#9045=VECTOR('',#30226,0.117775);
#9046=VECTOR('',#30229,0.117775);
#9047=VECTOR('',#30232,0.117775);
#9048=VECTOR('',#30235,0.117775);
#9049=VECTOR('',#30238,0.117775);
#9050=VECTOR('',#30241,0.117775);
#9051=VECTOR('',#30244,0.117775);
#9052=VECTOR('',#30247,0.117775);
#9053=VECTOR('',#30250,0.117775);
#9054=VECTOR('',#30253,0.117775);
#9055=VECTOR('',#30256,0.117775);
#9056=VECTOR('',#30259,0.117775);
#9057=VECTOR('',#30262,0.117775);
#9058=VECTOR('',#30265,0.117775);
#9059=VECTOR('',#30268,0.117775);
#9060=VECTOR('',#30271,0.117775);
#9061=VECTOR('',#30274,0.117775);
#9062=VECTOR('',#30277,0.117775);
#9063=VECTOR('',#30280,0.117775);
#9064=VECTOR('',#30283,0.117775);
#9065=VECTOR('',#30286,0.117775);
#9066=VECTOR('',#30289,0.117775);
#9067=VECTOR('',#30292,0.117775);
#9068=VECTOR('',#30295,0.117775);
#9069=VECTOR('',#30298,0.117775);
#9070=VECTOR('',#30301,0.117775);
#9071=VECTOR('',#30304,0.117775);
#9072=VECTOR('',#30307,0.117775);
#9073=VECTOR('',#30310,0.117775);
#9074=VECTOR('',#30313,0.117775);
#9075=VECTOR('',#30316,0.117775);
#9076=VECTOR('',#30319,0.117775);
#9077=VECTOR('',#30322,0.117775);
#9078=VECTOR('',#30325,0.117775);
#9079=VECTOR('',#30328,0.117775);
#9080=VECTOR('',#30331,0.117775);
#9081=VECTOR('',#30334,0.117775);
#9082=VECTOR('',#30337,0.117775);
#9083=VECTOR('',#30340,0.117775);
#9084=VECTOR('',#30343,0.117775);
#9085=VECTOR('',#30346,0.117775);
#9086=VECTOR('',#30349,0.117775);
#9087=VECTOR('',#30352,0.117775);
#9088=VECTOR('',#30355,0.117775);
#9089=VECTOR('',#30358,0.117775);
#9090=VECTOR('',#30361,0.117775);
#9091=VECTOR('',#30364,0.117775);
#9092=VECTOR('',#30367,0.117775);
#9093=VECTOR('',#30370,0.117775);
#9094=VECTOR('',#30373,0.117775);
#9095=VECTOR('',#30376,0.117775);
#9096=VECTOR('',#30379,0.117775);
#9097=VECTOR('',#30382,0.117775);
#9098=VECTOR('',#30399,1.);
#9099=VECTOR('',#30400,1.);
#9100=VECTOR('',#30403,1.);
#9101=VECTOR('',#30404,1.);
#9102=VECTOR('',#30407,1.);
#9103=VECTOR('',#30412,1.);
#9104=VECTOR('',#30413,1.);
#9105=VECTOR('',#30416,1.);
#9106=VECTOR('',#30417,1.);
#9107=VECTOR('',#30420,1.);
#9108=VECTOR('',#30425,1.);
#9109=VECTOR('',#30426,1.);
#9110=VECTOR('',#30429,1.);
#9111=VECTOR('',#30430,1.);
#9112=VECTOR('',#30433,1.);
#9113=VECTOR('',#30438,1.);
#9114=VECTOR('',#30439,1.);
#9115=VECTOR('',#30442,1.);
#9116=VECTOR('',#30443,1.);
#9117=VECTOR('',#30446,1.);
#9118=VECTOR('',#30451,1.);
#9119=VECTOR('',#30452,1.);
#9120=VECTOR('',#30455,1.);
#9121=VECTOR('',#30456,1.);
#9122=VECTOR('',#30459,1.);
#9123=VECTOR('',#30464,1.);
#9124=VECTOR('',#30465,1.);
#9125=VECTOR('',#30468,1.);
#9126=VECTOR('',#30469,1.);
#9127=VECTOR('',#30472,1.);
#9128=VECTOR('',#30477,1.);
#9129=VECTOR('',#30478,1.);
#9130=VECTOR('',#30481,1.);
#9131=VECTOR('',#30482,1.);
#9132=VECTOR('',#30485,1.);
#9133=VECTOR('',#30490,1.);
#9134=VECTOR('',#30491,1.);
#9135=VECTOR('',#30494,1.);
#9136=VECTOR('',#30495,1.);
#9137=VECTOR('',#30498,1.);
#9138=VECTOR('',#30503,1.);
#9139=VECTOR('',#30504,1.);
#9140=VECTOR('',#30507,1.);
#9141=VECTOR('',#30508,1.);
#9142=VECTOR('',#30511,1.);
#9143=VECTOR('',#30516,1.);
#9144=VECTOR('',#30517,1.);
#9145=VECTOR('',#30520,1.);
#9146=VECTOR('',#30521,1.);
#9147=VECTOR('',#30524,1.);
#9148=VECTOR('',#30529,1.);
#9149=VECTOR('',#30530,1.);
#9150=VECTOR('',#30533,1.);
#9151=VECTOR('',#30534,1.);
#9152=VECTOR('',#30537,1.);
#9153=VECTOR('',#30542,1.);
#9154=VECTOR('',#30543,1.);
#9155=VECTOR('',#30546,1.);
#9156=VECTOR('',#30547,1.);
#9157=VECTOR('',#30550,1.);
#9158=VECTOR('',#30555,1.);
#9159=VECTOR('',#30556,1.);
#9160=VECTOR('',#30559,1.);
#9161=VECTOR('',#30560,1.);
#9162=VECTOR('',#30563,1.);
#9163=VECTOR('',#30568,1.);
#9164=VECTOR('',#30569,1.);
#9165=VECTOR('',#30572,1.);
#9166=VECTOR('',#30573,1.);
#9167=VECTOR('',#30576,1.);
#9168=VECTOR('',#30581,1.);
#9169=VECTOR('',#30582,1.);
#9170=VECTOR('',#30585,1.);
#9171=VECTOR('',#30586,1.);
#9172=VECTOR('',#30589,1.);
#9173=VECTOR('',#30594,1.);
#9174=VECTOR('',#30595,1.);
#9175=VECTOR('',#30598,1.);
#9176=VECTOR('',#30599,1.);
#9177=VECTOR('',#30602,1.);
#9178=VECTOR('',#30607,1.);
#9179=VECTOR('',#30608,1.);
#9180=VECTOR('',#30611,1.);
#9181=VECTOR('',#30612,1.);
#9182=VECTOR('',#30615,1.);
#9183=VECTOR('',#30620,1.);
#9184=VECTOR('',#30621,1.);
#9185=VECTOR('',#30626,1.);
#9186=VECTOR('',#30627,1.);
#9187=VECTOR('',#30630,1.);
#9188=VECTOR('',#30635,1.);
#9189=VECTOR('',#30636,1.);
#9190=VECTOR('',#30639,1.);
#9191=VECTOR('',#30640,1.);
#9192=VECTOR('',#30643,1.);
#9193=VECTOR('',#30648,1.);
#9194=VECTOR('',#30649,1.);
#9195=VECTOR('',#30652,1.);
#9196=VECTOR('',#30653,1.);
#9197=VECTOR('',#30656,1.);
#9198=VECTOR('',#30661,1.);
#9199=VECTOR('',#30662,1.);
#9200=VECTOR('',#30665,1.);
#9201=VECTOR('',#30666,1.);
#9202=VECTOR('',#30669,1.);
#9203=VECTOR('',#30674,1.);
#9204=VECTOR('',#30675,1.);
#9205=VECTOR('',#30678,1.);
#9206=VECTOR('',#30679,1.);
#9207=VECTOR('',#30682,1.);
#9208=VECTOR('',#30687,1.);
#9209=VECTOR('',#30688,1.);
#9210=VECTOR('',#30691,1.);
#9211=VECTOR('',#30692,1.);
#9212=VECTOR('',#30695,1.);
#9213=VECTOR('',#30700,1.);
#9214=VECTOR('',#30701,1.);
#9215=VECTOR('',#30704,1.);
#9216=VECTOR('',#30705,1.);
#9217=VECTOR('',#30708,1.);
#9218=VECTOR('',#30713,1.);
#9219=VECTOR('',#30714,1.);
#9220=VECTOR('',#30717,1.);
#9221=VECTOR('',#30718,1.);
#9222=VECTOR('',#30721,1.);
#9223=VECTOR('',#30726,1.);
#9224=VECTOR('',#30727,1.);
#9225=VECTOR('',#30730,1.);
#9226=VECTOR('',#30731,1.);
#9227=VECTOR('',#30734,1.);
#9228=VECTOR('',#30739,1.);
#9229=VECTOR('',#30740,1.);
#9230=VECTOR('',#30743,1.);
#9231=VECTOR('',#30744,1.);
#9232=VECTOR('',#30747,1.);
#9233=VECTOR('',#30752,1.);
#9234=VECTOR('',#30753,1.);
#9235=VECTOR('',#30756,1.);
#9236=VECTOR('',#30757,1.);
#9237=VECTOR('',#30760,1.);
#9238=VECTOR('',#30765,1.);
#9239=VECTOR('',#30766,1.);
#9240=VECTOR('',#30769,1.);
#9241=VECTOR('',#30770,1.);
#9242=VECTOR('',#30773,1.);
#9243=VECTOR('',#30778,1.);
#9244=VECTOR('',#30779,1.);
#9245=VECTOR('',#30782,1.);
#9246=VECTOR('',#30783,1.);
#9247=VECTOR('',#30786,1.);
#9248=VECTOR('',#30791,1.);
#9249=VECTOR('',#30792,1.);
#9250=VECTOR('',#30795,1.);
#9251=VECTOR('',#30796,1.);
#9252=VECTOR('',#30799,1.);
#9253=VECTOR('',#30804,1.);
#9254=VECTOR('',#30805,1.);
#9255=VECTOR('',#30808,1.);
#9256=VECTOR('',#30809,1.);
#9257=VECTOR('',#30812,1.);
#9258=VECTOR('',#30817,1.);
#9259=VECTOR('',#30818,1.);
#9260=VECTOR('',#30821,1.);
#9261=VECTOR('',#30822,1.);
#9262=VECTOR('',#30825,1.);
#9263=VECTOR('',#30830,1.);
#9264=VECTOR('',#30831,1.);
#9265=VECTOR('',#30834,1.);
#9266=VECTOR('',#30835,1.);
#9267=VECTOR('',#30838,1.);
#9268=VECTOR('',#30843,1.);
#9269=VECTOR('',#30844,1.);
#9270=VECTOR('',#30847,1.);
#9271=VECTOR('',#30848,1.);
#9272=VECTOR('',#30851,1.);
#9273=VECTOR('',#30888,0.275);
#9274=VECTOR('',#30927,1.);
#9275=VECTOR('',#30930,1.);
#9276=VECTOR('',#30935,1.);
#9277=VECTOR('',#30936,1.);
#9278=VECTOR('',#30939,1.);
#9279=VECTOR('',#30946,0.2675);
#9280=VECTOR('',#30949,0.0577350269189626);
#9281=VECTOR('',#30954,1.);
#9282=VECTOR('',#30955,1.);
#9283=VECTOR('',#30956,1.);
#9284=VECTOR('',#30957,1.);
#9285=VECTOR('',#30960,1.);
#9286=VECTOR('',#30961,1.);
#9287=VECTOR('',#30962,1.);
#9288=VECTOR('',#30965,1.);
#9289=VECTOR('',#30966,1.);
#9290=VECTOR('',#30967,1.);
#9291=VECTOR('',#30970,1.);
#9292=VECTOR('',#30971,1.);
#9293=VECTOR('',#30972,1.);
#9294=VECTOR('',#30975,1.);
#9295=VECTOR('',#30976,1.);
#9296=VECTOR('',#30977,1.);
#9297=VECTOR('',#30980,1.);
#9298=VECTOR('',#30981,1.);
#9299=VECTOR('',#30990,0.132);
#9300=VECTOR('',#30999,0.155);
#10911=VERTEX_POINT('',#41663);
#10912=VERTEX_POINT('',#41664);
#10913=VERTEX_POINT('',#41666);
#10914=VERTEX_POINT('',#41683);
#10915=VERTEX_POINT('',#41685);
#10916=VERTEX_POINT('',#41688);
#10917=VERTEX_POINT('',#41704);
#10918=VERTEX_POINT('',#41705);
#10919=VERTEX_POINT('',#41752);
#10920=VERTEX_POINT('',#41753);
#10921=VERTEX_POINT('',#41806);
#10922=VERTEX_POINT('',#41807);
#10923=VERTEX_POINT('',#41854);
#10924=VERTEX_POINT('',#41855);
#10925=VERTEX_POINT('',#41902);
#10926=VERTEX_POINT('',#41903);
#10927=VERTEX_POINT('',#41956);
#10928=VERTEX_POINT('',#41957);
#10929=VERTEX_POINT('',#42004);
#10930=VERTEX_POINT('',#42005);
#10931=VERTEX_POINT('',#42052);
#10932=VERTEX_POINT('',#42053);
#10933=VERTEX_POINT('',#42100);
#10934=VERTEX_POINT('',#42101);
#10935=VERTEX_POINT('',#42154);
#10936=VERTEX_POINT('',#42155);
#10937=VERTEX_POINT('',#42202);
#10938=VERTEX_POINT('',#42203);
#10939=VERTEX_POINT('',#42250);
#10940=VERTEX_POINT('',#42251);
#10941=VERTEX_POINT('',#42304);
#10942=VERTEX_POINT('',#42305);
#10943=VERTEX_POINT('',#42352);
#10944=VERTEX_POINT('',#42353);
#10945=VERTEX_POINT('',#42400);
#10946=VERTEX_POINT('',#42401);
#10947=VERTEX_POINT('',#42451);
#10948=VERTEX_POINT('',#42452);
#10949=VERTEX_POINT('',#42502);
#10950=VERTEX_POINT('',#42503);
#10951=VERTEX_POINT('',#42550);
#10952=VERTEX_POINT('',#42551);
#10953=VERTEX_POINT('',#42598);
#10954=VERTEX_POINT('',#42599);
#10955=VERTEX_POINT('',#42652);
#10956=VERTEX_POINT('',#42653);
#10957=VERTEX_POINT('',#42700);
#10958=VERTEX_POINT('',#42701);
#10959=VERTEX_POINT('',#42748);
#10960=VERTEX_POINT('',#42749);
#10961=VERTEX_POINT('',#42802);
#10962=VERTEX_POINT('',#42803);
#10963=VERTEX_POINT('',#42850);
#10964=VERTEX_POINT('',#42851);
#10965=VERTEX_POINT('',#42898);
#10966=VERTEX_POINT('',#42899);
#10967=VERTEX_POINT('',#42946);
#10968=VERTEX_POINT('',#42947);
#10969=VERTEX_POINT('',#43000);
#10970=VERTEX_POINT('',#43001);
#10971=VERTEX_POINT('',#43048);
#10972=VERTEX_POINT('',#43049);
#10973=VERTEX_POINT('',#43096);
#10974=VERTEX_POINT('',#43097);
#10975=VERTEX_POINT('',#43150);
#10976=VERTEX_POINT('',#43151);
#10977=VERTEX_POINT('',#43198);
#10978=VERTEX_POINT('',#43199);
#10979=VERTEX_POINT('',#43246);
#10980=VERTEX_POINT('',#43247);
#10981=VERTEX_POINT('',#43294);
#10982=VERTEX_POINT('',#43295);
#10983=VERTEX_POINT('',#43348);
#10984=VERTEX_POINT('',#43349);
#10985=VERTEX_POINT('',#43396);
#10986=VERTEX_POINT('',#43397);
#10987=VERTEX_POINT('',#43444);
#10988=VERTEX_POINT('',#43445);
#10989=VERTEX_POINT('',#43498);
#10990=VERTEX_POINT('',#43499);
#10991=VERTEX_POINT('',#43546);
#10992=VERTEX_POINT('',#43547);
#10993=VERTEX_POINT('',#43594);
#10994=VERTEX_POINT('',#43595);
#10995=VERTEX_POINT('',#43645);
#10996=VERTEX_POINT('',#43646);
#10997=VERTEX_POINT('',#43696);
#10998=VERTEX_POINT('',#43697);
#10999=VERTEX_POINT('',#43744);
#11000=VERTEX_POINT('',#43745);
#11001=VERTEX_POINT('',#43792);
#11002=VERTEX_POINT('',#43793);
#11003=VERTEX_POINT('',#43846);
#11004=VERTEX_POINT('',#43847);
#11005=VERTEX_POINT('',#43894);
#11006=VERTEX_POINT('',#43895);
#11007=VERTEX_POINT('',#43942);
#11008=VERTEX_POINT('',#43943);
#11009=VERTEX_POINT('',#43996);
#11010=VERTEX_POINT('',#43997);
#11011=VERTEX_POINT('',#44044);
#11012=VERTEX_POINT('',#44045);
#11013=VERTEX_POINT('',#44092);
#11014=VERTEX_POINT('',#44093);
#11015=VERTEX_POINT('',#44140);
#11016=VERTEX_POINT('',#44141);
#11017=VERTEX_POINT('',#44194);
#11018=VERTEX_POINT('',#44195);
#11019=VERTEX_POINT('',#44242);
#11020=VERTEX_POINT('',#44243);
#11021=VERTEX_POINT('',#44290);
#11022=VERTEX_POINT('',#44291);
#11023=VERTEX_POINT('',#44344);
#11024=VERTEX_POINT('',#44345);
#11025=VERTEX_POINT('',#44392);
#11026=VERTEX_POINT('',#44393);
#11027=VERTEX_POINT('',#44440);
#11028=VERTEX_POINT('',#44441);
#11029=VERTEX_POINT('',#44488);
#11030=VERTEX_POINT('',#44489);
#11031=VERTEX_POINT('',#44542);
#11032=VERTEX_POINT('',#44543);
#11033=VERTEX_POINT('',#44545);
#11034=VERTEX_POINT('',#44552);
#11035=VERTEX_POINT('',#44560);
#11036=VERTEX_POINT('',#44561);
#11037=VERTEX_POINT('',#44585);
#11038=VERTEX_POINT('',#44586);
#11039=VERTEX_POINT('',#44610);
#11040=VERTEX_POINT('',#44611);
#11041=VERTEX_POINT('',#44634);
#11042=VERTEX_POINT('',#44635);
#11043=VERTEX_POINT('',#44658);
#11044=VERTEX_POINT('',#44659);
#11045=VERTEX_POINT('',#44683);
#11046=VERTEX_POINT('',#44684);
#11047=VERTEX_POINT('',#44708);
#11048=VERTEX_POINT('',#44709);
#11049=VERTEX_POINT('',#44732);
#11050=VERTEX_POINT('',#44733);
#11051=VERTEX_POINT('',#44757);
#11052=VERTEX_POINT('',#44758);
#11053=VERTEX_POINT('',#44782);
#11054=VERTEX_POINT('',#44783);
#11055=VERTEX_POINT('',#44806);
#11056=VERTEX_POINT('',#44807);
#11057=VERTEX_POINT('',#44830);
#11058=VERTEX_POINT('',#44831);
#11059=VERTEX_POINT('',#44855);
#11060=VERTEX_POINT('',#44856);
#11061=VERTEX_POINT('',#44880);
#11062=VERTEX_POINT('',#44881);
#11063=VERTEX_POINT('',#44904);
#11064=VERTEX_POINT('',#44905);
#11065=VERTEX_POINT('',#44929);
#11066=VERTEX_POINT('',#44930);
#11067=VERTEX_POINT('',#44954);
#11068=VERTEX_POINT('',#44955);
#11069=VERTEX_POINT('',#44978);
#11070=VERTEX_POINT('',#44979);
#11071=VERTEX_POINT('',#45003);
#11072=VERTEX_POINT('',#45004);
#11073=VERTEX_POINT('',#45027);
#11074=VERTEX_POINT('',#45028);
#11075=VERTEX_POINT('',#45052);
#11076=VERTEX_POINT('',#45053);
#11077=VERTEX_POINT('',#45076);
#11078=VERTEX_POINT('',#45077);
#11079=VERTEX_POINT('',#45101);
#11080=VERTEX_POINT('',#45102);
#11081=VERTEX_POINT('',#45126);
#11082=VERTEX_POINT('',#45127);
#11083=VERTEX_POINT('',#45150);
#11084=VERTEX_POINT('',#45151);
#11085=VERTEX_POINT('',#45175);
#11086=VERTEX_POINT('',#45176);
#11087=VERTEX_POINT('',#45200);
#11088=VERTEX_POINT('',#45201);
#11089=VERTEX_POINT('',#45224);
#11090=VERTEX_POINT('',#45225);
#11091=VERTEX_POINT('',#45248);
#11092=VERTEX_POINT('',#45249);
#11093=VERTEX_POINT('',#45273);
#11094=VERTEX_POINT('',#45274);
#11095=VERTEX_POINT('',#45298);
#11096=VERTEX_POINT('',#45299);
#11097=VERTEX_POINT('',#45322);
#11098=VERTEX_POINT('',#45323);
#11099=VERTEX_POINT('',#45347);
#11100=VERTEX_POINT('',#45348);
#11101=VERTEX_POINT('',#45372);
#11102=VERTEX_POINT('',#45373);
#11103=VERTEX_POINT('',#45396);
#11104=VERTEX_POINT('',#45397);
#11105=VERTEX_POINT('',#45420);
#11106=VERTEX_POINT('',#45421);
#11107=VERTEX_POINT('',#45445);
#11108=VERTEX_POINT('',#45446);
#11109=VERTEX_POINT('',#45470);
#11110=VERTEX_POINT('',#45471);
#11111=VERTEX_POINT('',#45494);
#11112=VERTEX_POINT('',#45495);
#11113=VERTEX_POINT('',#45519);
#11114=VERTEX_POINT('',#45520);
#11115=VERTEX_POINT('',#45544);
#11116=VERTEX_POINT('',#45545);
#11117=VERTEX_POINT('',#45568);
#11118=VERTEX_POINT('',#45569);
#11119=VERTEX_POINT('',#45593);
#11120=VERTEX_POINT('',#45594);
#11121=VERTEX_POINT('',#45617);
#11122=VERTEX_POINT('',#45618);
#11123=VERTEX_POINT('',#45642);
#11124=VERTEX_POINT('',#45643);
#11125=VERTEX_POINT('',#45666);
#11126=VERTEX_POINT('',#45667);
#11127=VERTEX_POINT('',#45691);
#11128=VERTEX_POINT('',#45692);
#11129=VERTEX_POINT('',#45716);
#11130=VERTEX_POINT('',#45717);
#11131=VERTEX_POINT('',#45740);
#11132=VERTEX_POINT('',#45741);
#11133=VERTEX_POINT('',#45765);
#11134=VERTEX_POINT('',#45766);
#11135=VERTEX_POINT('',#45790);
#11136=VERTEX_POINT('',#45791);
#11137=VERTEX_POINT('',#45814);
#11138=VERTEX_POINT('',#45815);
#11139=VERTEX_POINT('',#45838);
#11140=VERTEX_POINT('',#45839);
#11141=VERTEX_POINT('',#45863);
#11142=VERTEX_POINT('',#45864);
#11143=VERTEX_POINT('',#45888);
#11144=VERTEX_POINT('',#45889);
#11145=VERTEX_POINT('',#45912);
#11146=VERTEX_POINT('',#45913);
#11147=VERTEX_POINT('',#45937);
#11148=VERTEX_POINT('',#45938);
#11149=VERTEX_POINT('',#45962);
#11150=VERTEX_POINT('',#45963);
#11151=VERTEX_POINT('',#45986);
#11152=VERTEX_POINT('',#46039);
#11153=VERTEX_POINT('',#46041);
#11154=VERTEX_POINT('',#47606);
#11155=VERTEX_POINT('',#47665);
#11156=VERTEX_POINT('',#49233);
#11157=VERTEX_POINT('',#49234);
#11158=VERTEX_POINT('',#49236);
#11159=VERTEX_POINT('',#49240);
#11160=VERTEX_POINT('',#49242);
#11161=VERTEX_POINT('',#49248);
#11162=VERTEX_POINT('',#49254);
#11163=VERTEX_POINT('',#49255);
#11164=VERTEX_POINT('',#49257);
#11165=VERTEX_POINT('',#49261);
#11166=VERTEX_POINT('',#49263);
#11167=VERTEX_POINT('',#49269);
#11168=VERTEX_POINT('',#49275);
#11169=VERTEX_POINT('',#49276);
#11170=VERTEX_POINT('',#49278);
#11171=VERTEX_POINT('',#49282);
#11172=VERTEX_POINT('',#49284);
#11173=VERTEX_POINT('',#49290);
#11174=VERTEX_POINT('',#49296);
#11175=VERTEX_POINT('',#49297);
#11176=VERTEX_POINT('',#49299);
#11177=VERTEX_POINT('',#49303);
#11178=VERTEX_POINT('',#49305);
#11179=VERTEX_POINT('',#49311);
#11180=VERTEX_POINT('',#49317);
#11181=VERTEX_POINT('',#49318);
#11182=VERTEX_POINT('',#49320);
#11183=VERTEX_POINT('',#49324);
#11184=VERTEX_POINT('',#49326);
#11185=VERTEX_POINT('',#49332);
#11186=VERTEX_POINT('',#49338);
#11187=VERTEX_POINT('',#49339);
#11188=VERTEX_POINT('',#49341);
#11189=VERTEX_POINT('',#49345);
#11190=VERTEX_POINT('',#49347);
#11191=VERTEX_POINT('',#49353);
#11192=VERTEX_POINT('',#49359);
#11193=VERTEX_POINT('',#49360);
#11194=VERTEX_POINT('',#49362);
#11195=VERTEX_POINT('',#49366);
#11196=VERTEX_POINT('',#49368);
#11197=VERTEX_POINT('',#49374);
#11198=VERTEX_POINT('',#49380);
#11199=VERTEX_POINT('',#49381);
#11200=VERTEX_POINT('',#49383);
#11201=VERTEX_POINT('',#49387);
#11202=VERTEX_POINT('',#49389);
#11203=VERTEX_POINT('',#49395);
#11204=VERTEX_POINT('',#49401);
#11205=VERTEX_POINT('',#49402);
#11206=VERTEX_POINT('',#49404);
#11207=VERTEX_POINT('',#49408);
#11208=VERTEX_POINT('',#49410);
#11209=VERTEX_POINT('',#49416);
#11210=VERTEX_POINT('',#49422);
#11211=VERTEX_POINT('',#49423);
#11212=VERTEX_POINT('',#49425);
#11213=VERTEX_POINT('',#49429);
#11214=VERTEX_POINT('',#49431);
#11215=VERTEX_POINT('',#49437);
#11216=VERTEX_POINT('',#49443);
#11217=VERTEX_POINT('',#49444);
#11218=VERTEX_POINT('',#49446);
#11219=VERTEX_POINT('',#49450);
#11220=VERTEX_POINT('',#49452);
#11221=VERTEX_POINT('',#49458);
#11222=VERTEX_POINT('',#49464);
#11223=VERTEX_POINT('',#49465);
#11224=VERTEX_POINT('',#49467);
#11225=VERTEX_POINT('',#49471);
#11226=VERTEX_POINT('',#49473);
#11227=VERTEX_POINT('',#49479);
#11228=VERTEX_POINT('',#49485);
#11229=VERTEX_POINT('',#49486);
#11230=VERTEX_POINT('',#49488);
#11231=VERTEX_POINT('',#49492);
#11232=VERTEX_POINT('',#49494);
#11233=VERTEX_POINT('',#49500);
#11234=VERTEX_POINT('',#49506);
#11235=VERTEX_POINT('',#49507);
#11236=VERTEX_POINT('',#49509);
#11237=VERTEX_POINT('',#49513);
#11238=VERTEX_POINT('',#49515);
#11239=VERTEX_POINT('',#49521);
#11240=VERTEX_POINT('',#49527);
#11241=VERTEX_POINT('',#49528);
#11242=VERTEX_POINT('',#49530);
#11243=VERTEX_POINT('',#49534);
#11244=VERTEX_POINT('',#49536);
#11245=VERTEX_POINT('',#49542);
#11246=VERTEX_POINT('',#49548);
#11247=VERTEX_POINT('',#49549);
#11248=VERTEX_POINT('',#49551);
#11249=VERTEX_POINT('',#49555);
#11250=VERTEX_POINT('',#49557);
#11251=VERTEX_POINT('',#49563);
#11252=VERTEX_POINT('',#49569);
#11253=VERTEX_POINT('',#49570);
#11254=VERTEX_POINT('',#49572);
#11255=VERTEX_POINT('',#49576);
#11256=VERTEX_POINT('',#49578);
#11257=VERTEX_POINT('',#49584);
#11258=VERTEX_POINT('',#49590);
#11259=VERTEX_POINT('',#49591);
#11260=VERTEX_POINT('',#49593);
#11261=VERTEX_POINT('',#49595);
#11262=VERTEX_POINT('',#49599);
#11263=VERTEX_POINT('',#49601);
#11264=VERTEX_POINT('',#49607);
#11265=VERTEX_POINT('',#49613);
#11266=VERTEX_POINT('',#49614);
#11267=VERTEX_POINT('',#49616);
#11268=VERTEX_POINT('',#49620);
#11269=VERTEX_POINT('',#49622);
#11270=VERTEX_POINT('',#49628);
#11271=VERTEX_POINT('',#49634);
#11272=VERTEX_POINT('',#49635);
#11273=VERTEX_POINT('',#49637);
#11274=VERTEX_POINT('',#49641);
#11275=VERTEX_POINT('',#49643);
#11276=VERTEX_POINT('',#49649);
#11277=VERTEX_POINT('',#49655);
#11278=VERTEX_POINT('',#49656);
#11279=VERTEX_POINT('',#49658);
#11280=VERTEX_POINT('',#49662);
#11281=VERTEX_POINT('',#49664);
#11282=VERTEX_POINT('',#49670);
#11283=VERTEX_POINT('',#49676);
#11284=VERTEX_POINT('',#49677);
#11285=VERTEX_POINT('',#49679);
#11286=VERTEX_POINT('',#49683);
#11287=VERTEX_POINT('',#49685);
#11288=VERTEX_POINT('',#49691);
#11289=VERTEX_POINT('',#49697);
#11290=VERTEX_POINT('',#49698);
#11291=VERTEX_POINT('',#49700);
#11292=VERTEX_POINT('',#49704);
#11293=VERTEX_POINT('',#49706);
#11294=VERTEX_POINT('',#49712);
#11295=VERTEX_POINT('',#49718);
#11296=VERTEX_POINT('',#49719);
#11297=VERTEX_POINT('',#49721);
#11298=VERTEX_POINT('',#49725);
#11299=VERTEX_POINT('',#49727);
#11300=VERTEX_POINT('',#49733);
#11301=VERTEX_POINT('',#49739);
#11302=VERTEX_POINT('',#49740);
#11303=VERTEX_POINT('',#49742);
#11304=VERTEX_POINT('',#49746);
#11305=VERTEX_POINT('',#49748);
#11306=VERTEX_POINT('',#49754);
#11307=VERTEX_POINT('',#49760);
#11308=VERTEX_POINT('',#49761);
#11309=VERTEX_POINT('',#49763);
#11310=VERTEX_POINT('',#49767);
#11311=VERTEX_POINT('',#49769);
#11312=VERTEX_POINT('',#49775);
#11313=VERTEX_POINT('',#49781);
#11314=VERTEX_POINT('',#49782);
#11315=VERTEX_POINT('',#49784);
#11316=VERTEX_POINT('',#49788);
#11317=VERTEX_POINT('',#49790);
#11318=VERTEX_POINT('',#49796);
#11319=VERTEX_POINT('',#49802);
#11320=VERTEX_POINT('',#49803);
#11321=VERTEX_POINT('',#49805);
#11322=VERTEX_POINT('',#49809);
#11323=VERTEX_POINT('',#49811);
#11324=VERTEX_POINT('',#49817);
#11325=VERTEX_POINT('',#49823);
#11326=VERTEX_POINT('',#49824);
#11327=VERTEX_POINT('',#49826);
#11328=VERTEX_POINT('',#49830);
#11329=VERTEX_POINT('',#49832);
#11330=VERTEX_POINT('',#49838);
#11331=VERTEX_POINT('',#49844);
#11332=VERTEX_POINT('',#49845);
#11333=VERTEX_POINT('',#49847);
#11334=VERTEX_POINT('',#49851);
#11335=VERTEX_POINT('',#49853);
#11336=VERTEX_POINT('',#49859);
#11337=VERTEX_POINT('',#49865);
#11338=VERTEX_POINT('',#49866);
#11339=VERTEX_POINT('',#49868);
#11340=VERTEX_POINT('',#49872);
#11341=VERTEX_POINT('',#49874);
#11342=VERTEX_POINT('',#49880);
#11343=VERTEX_POINT('',#49886);
#11344=VERTEX_POINT('',#49887);
#11345=VERTEX_POINT('',#49889);
#11346=VERTEX_POINT('',#49893);
#11347=VERTEX_POINT('',#49895);
#11348=VERTEX_POINT('',#49901);
#11349=VERTEX_POINT('',#49907);
#11350=VERTEX_POINT('',#49908);
#11351=VERTEX_POINT('',#49910);
#11352=VERTEX_POINT('',#49914);
#11353=VERTEX_POINT('',#49916);
#11354=VERTEX_POINT('',#49922);
#11355=VERTEX_POINT('',#49928);
#11356=VERTEX_POINT('',#49929);
#11357=VERTEX_POINT('',#49931);
#11358=VERTEX_POINT('',#49935);
#11359=VERTEX_POINT('',#49937);
#11360=VERTEX_POINT('',#49943);
#11361=VERTEX_POINT('',#49949);
#11362=VERTEX_POINT('',#49950);
#11363=VERTEX_POINT('',#49952);
#11364=VERTEX_POINT('',#49956);
#11365=VERTEX_POINT('',#49958);
#11366=VERTEX_POINT('',#49964);
#11367=VERTEX_POINT('',#49987);
#11368=VERTEX_POINT('',#50007);
#11369=VERTEX_POINT('',#50009);
#11370=VERTEX_POINT('',#50011);
#11371=VERTEX_POINT('',#50013);
#11372=VERTEX_POINT('',#50017);
#11373=VERTEX_POINT('',#50019);
#11374=VERTEX_POINT('',#50031);
#11375=VERTEX_POINT('',#50035);
#11376=VERTEX_POINT('',#50036);
#11377=VERTEX_POINT('',#50040);
#11378=VERTEX_POINT('',#50041);
#11379=VERTEX_POINT('',#50043);
#11380=VERTEX_POINT('',#50045);
#11381=VERTEX_POINT('',#50049);
#11382=VERTEX_POINT('',#50051);
#11383=VERTEX_POINT('',#50055);
#11384=VERTEX_POINT('',#50057);
#11385=VERTEX_POINT('',#50061);
#11386=VERTEX_POINT('',#50063);
#11387=VERTEX_POINT('',#50067);
#11388=VERTEX_POINT('',#50069);
#11389=VERTEX_POINT('',#50077);
#11390=VERTEX_POINT('',#50084);
#13865=EDGE_CURVE('',#10911,#10912,#7135,.T.);
#13866=EDGE_CURVE('',#10911,#10913,#555,.T.);
#13867=EDGE_CURVE('',#10913,#10914,#5680,.T.);
#13868=EDGE_CURVE('',#10914,#10915,#7136,.T.);
#13869=EDGE_CURVE('',#10915,#10915,#5681,.T.);
#13870=EDGE_CURVE('',#10914,#10916,#5682,.T.);
#13871=EDGE_CURVE('',#10916,#10912,#556,.T.);
#13872=EDGE_CURVE('',#10917,#10918,#7137,.T.);
#13873=EDGE_CURVE('',#10917,#10911,#557,.T.);
#13874=EDGE_CURVE('',#10912,#10918,#558,.T.);
#13875=EDGE_CURVE('',#10919,#10920,#7138,.T.);
#13876=EDGE_CURVE('',#10919,#10917,#559,.T.);
#13877=EDGE_CURVE('',#10918,#10920,#560,.T.);
#13878=EDGE_CURVE('',#10921,#10922,#7139,.T.);
#13879=EDGE_CURVE('',#10921,#10919,#561,.T.);
#13880=EDGE_CURVE('',#10920,#10922,#562,.T.);
#13881=EDGE_CURVE('',#10923,#10924,#7140,.T.);
#13882=EDGE_CURVE('',#10923,#10921,#563,.T.);
#13883=EDGE_CURVE('',#10922,#10924,#564,.T.);
#13884=EDGE_CURVE('',#10925,#10926,#7141,.T.);
#13885=EDGE_CURVE('',#10925,#10923,#565,.T.);
#13886=EDGE_CURVE('',#10924,#10926,#566,.T.);
#13887=EDGE_CURVE('',#10927,#10928,#7142,.T.);
#13888=EDGE_CURVE('',#10927,#10925,#567,.T.);
#13889=EDGE_CURVE('',#10926,#10928,#568,.T.);
#13890=EDGE_CURVE('',#10929,#10930,#7143,.T.);
#13891=EDGE_CURVE('',#10929,#10927,#569,.T.);
#13892=EDGE_CURVE('',#10928,#10930,#570,.T.);
#13893=EDGE_CURVE('',#10931,#10932,#7144,.T.);
#13894=EDGE_CURVE('',#10931,#10929,#571,.T.);
#13895=EDGE_CURVE('',#10930,#10932,#572,.T.);
#13896=EDGE_CURVE('',#10933,#10934,#7145,.T.);
#13897=EDGE_CURVE('',#10933,#10931,#573,.T.);
#13898=EDGE_CURVE('',#10932,#10934,#574,.T.);
#13899=EDGE_CURVE('',#10935,#10936,#7146,.T.);
#13900=EDGE_CURVE('',#10935,#10933,#575,.T.);
#13901=EDGE_CURVE('',#10934,#10936,#576,.T.);
#13902=EDGE_CURVE('',#10937,#10938,#7147,.T.);
#13903=EDGE_CURVE('',#10937,#10935,#577,.T.);
#13904=EDGE_CURVE('',#10936,#10938,#578,.T.);
#13905=EDGE_CURVE('',#10939,#10940,#7148,.T.);
#13906=EDGE_CURVE('',#10939,#10937,#579,.T.);
#13907=EDGE_CURVE('',#10938,#10940,#580,.T.);
#13908=EDGE_CURVE('',#10941,#10942,#7149,.T.);
#13909=EDGE_CURVE('',#10941,#10939,#581,.T.);
#13910=EDGE_CURVE('',#10940,#10942,#582,.T.);
#13911=EDGE_CURVE('',#10943,#10944,#7150,.T.);
#13912=EDGE_CURVE('',#10943,#10941,#583,.T.);
#13913=EDGE_CURVE('',#10942,#10944,#584,.T.);
#13914=EDGE_CURVE('',#10945,#10946,#7151,.T.);
#13915=EDGE_CURVE('',#10945,#10943,#585,.T.);
#13916=EDGE_CURVE('',#10944,#10946,#586,.T.);
#13917=EDGE_CURVE('',#10947,#10948,#7152,.T.);
#13918=EDGE_CURVE('',#10947,#10945,#587,.T.);
#13919=EDGE_CURVE('',#10946,#10948,#588,.T.);
#13920=EDGE_CURVE('',#10949,#10950,#7153,.T.);
#13921=EDGE_CURVE('',#10949,#10947,#589,.T.);
#13922=EDGE_CURVE('',#10948,#10950,#590,.T.);
#13923=EDGE_CURVE('',#10951,#10952,#7154,.T.);
#13924=EDGE_CURVE('',#10951,#10949,#591,.T.);
#13925=EDGE_CURVE('',#10950,#10952,#592,.T.);
#13926=EDGE_CURVE('',#10953,#10954,#7155,.T.);
#13927=EDGE_CURVE('',#10953,#10951,#593,.T.);
#13928=EDGE_CURVE('',#10952,#10954,#594,.T.);
#13929=EDGE_CURVE('',#10955,#10956,#7156,.T.);
#13930=EDGE_CURVE('',#10955,#10953,#595,.T.);
#13931=EDGE_CURVE('',#10954,#10956,#596,.T.);
#13932=EDGE_CURVE('',#10957,#10958,#7157,.T.);
#13933=EDGE_CURVE('',#10957,#10955,#597,.T.);
#13934=EDGE_CURVE('',#10956,#10958,#598,.T.);
#13935=EDGE_CURVE('',#10959,#10960,#7158,.T.);
#13936=EDGE_CURVE('',#10959,#10957,#599,.T.);
#13937=EDGE_CURVE('',#10958,#10960,#600,.T.);
#13938=EDGE_CURVE('',#10961,#10962,#7159,.T.);
#13939=EDGE_CURVE('',#10961,#10959,#601,.T.);
#13940=EDGE_CURVE('',#10960,#10962,#602,.T.);
#13941=EDGE_CURVE('',#10963,#10964,#7160,.T.);
#13942=EDGE_CURVE('',#10963,#10961,#603,.T.);
#13943=EDGE_CURVE('',#10962,#10964,#604,.T.);
#13944=EDGE_CURVE('',#10965,#10966,#7161,.T.);
#13945=EDGE_CURVE('',#10965,#10963,#605,.T.);
#13946=EDGE_CURVE('',#10964,#10966,#606,.T.);
#13947=EDGE_CURVE('',#10967,#10968,#7162,.T.);
#13948=EDGE_CURVE('',#10967,#10965,#607,.T.);
#13949=EDGE_CURVE('',#10966,#10968,#608,.T.);
#13950=EDGE_CURVE('',#10969,#10970,#7163,.T.);
#13951=EDGE_CURVE('',#10969,#10967,#609,.T.);
#13952=EDGE_CURVE('',#10968,#10970,#610,.T.);
#13953=EDGE_CURVE('',#10971,#10972,#7164,.T.);
#13954=EDGE_CURVE('',#10971,#10969,#611,.T.);
#13955=EDGE_CURVE('',#10970,#10972,#612,.T.);
#13956=EDGE_CURVE('',#10973,#10974,#7165,.T.);
#13957=EDGE_CURVE('',#10973,#10971,#613,.T.);
#13958=EDGE_CURVE('',#10972,#10974,#614,.T.);
#13959=EDGE_CURVE('',#10975,#10976,#7166,.T.);
#13960=EDGE_CURVE('',#10975,#10973,#615,.T.);
#13961=EDGE_CURVE('',#10974,#10976,#616,.T.);
#13962=EDGE_CURVE('',#10977,#10978,#7167,.T.);
#13963=EDGE_CURVE('',#10977,#10975,#617,.T.);
#13964=EDGE_CURVE('',#10976,#10978,#618,.T.);
#13965=EDGE_CURVE('',#10979,#10980,#7168,.T.);
#13966=EDGE_CURVE('',#10979,#10977,#619,.T.);
#13967=EDGE_CURVE('',#10978,#10980,#620,.T.);
#13968=EDGE_CURVE('',#10981,#10982,#7169,.T.);
#13969=EDGE_CURVE('',#10981,#10979,#621,.T.);
#13970=EDGE_CURVE('',#10980,#10982,#622,.T.);
#13971=EDGE_CURVE('',#10983,#10984,#7170,.T.);
#13972=EDGE_CURVE('',#10983,#10981,#623,.T.);
#13973=EDGE_CURVE('',#10982,#10984,#624,.T.);
#13974=EDGE_CURVE('',#10985,#10986,#7171,.T.);
#13975=EDGE_CURVE('',#10985,#10983,#625,.T.);
#13976=EDGE_CURVE('',#10984,#10986,#626,.T.);
#13977=EDGE_CURVE('',#10987,#10988,#7172,.T.);
#13978=EDGE_CURVE('',#10987,#10985,#627,.T.);
#13979=EDGE_CURVE('',#10986,#10988,#628,.T.);
#13980=EDGE_CURVE('',#10989,#10990,#7173,.T.);
#13981=EDGE_CURVE('',#10989,#10987,#629,.T.);
#13982=EDGE_CURVE('',#10988,#10990,#630,.T.);
#13983=EDGE_CURVE('',#10991,#10992,#7174,.T.);
#13984=EDGE_CURVE('',#10991,#10989,#631,.T.);
#13985=EDGE_CURVE('',#10990,#10992,#632,.T.);
#13986=EDGE_CURVE('',#10993,#10994,#7175,.T.);
#13987=EDGE_CURVE('',#10993,#10991,#633,.T.);
#13988=EDGE_CURVE('',#10992,#10994,#634,.T.);
#13989=EDGE_CURVE('',#10995,#10996,#7176,.T.);
#13990=EDGE_CURVE('',#10995,#10993,#635,.T.);
#13991=EDGE_CURVE('',#10994,#10996,#636,.T.);
#13992=EDGE_CURVE('',#10997,#10998,#7177,.T.);
#13993=EDGE_CURVE('',#10997,#10995,#637,.T.);
#13994=EDGE_CURVE('',#10996,#10998,#638,.T.);
#13995=EDGE_CURVE('',#10999,#11000,#7178,.T.);
#13996=EDGE_CURVE('',#10999,#10997,#639,.T.);
#13997=EDGE_CURVE('',#10998,#11000,#640,.T.);
#13998=EDGE_CURVE('',#11001,#11002,#7179,.T.);
#13999=EDGE_CURVE('',#11001,#10999,#641,.T.);
#14000=EDGE_CURVE('',#11000,#11002,#642,.T.);
#14001=EDGE_CURVE('',#11003,#11004,#7180,.T.);
#14002=EDGE_CURVE('',#11003,#11001,#643,.T.);
#14003=EDGE_CURVE('',#11002,#11004,#644,.T.);
#14004=EDGE_CURVE('',#11005,#11006,#7181,.T.);
#14005=EDGE_CURVE('',#11005,#11003,#645,.T.);
#14006=EDGE_CURVE('',#11004,#11006,#646,.T.);
#14007=EDGE_CURVE('',#11007,#11008,#7182,.T.);
#14008=EDGE_CURVE('',#11007,#11005,#647,.T.);
#14009=EDGE_CURVE('',#11006,#11008,#648,.T.);
#14010=EDGE_CURVE('',#11009,#11010,#7183,.T.);
#14011=EDGE_CURVE('',#11009,#11007,#649,.T.);
#14012=EDGE_CURVE('',#11008,#11010,#650,.T.);
#14013=EDGE_CURVE('',#11011,#11012,#7184,.T.);
#14014=EDGE_CURVE('',#11011,#11009,#651,.T.);
#14015=EDGE_CURVE('',#11010,#11012,#652,.T.);
#14016=EDGE_CURVE('',#11013,#11014,#7185,.T.);
#14017=EDGE_CURVE('',#11013,#11011,#653,.T.);
#14018=EDGE_CURVE('',#11012,#11014,#654,.T.);
#14019=EDGE_CURVE('',#11015,#11016,#7186,.T.);
#14020=EDGE_CURVE('',#11015,#11013,#655,.T.);
#14021=EDGE_CURVE('',#11014,#11016,#656,.T.);
#14022=EDGE_CURVE('',#11017,#11018,#7187,.T.);
#14023=EDGE_CURVE('',#11017,#11015,#657,.T.);
#14024=EDGE_CURVE('',#11016,#11018,#658,.T.);
#14025=EDGE_CURVE('',#11019,#11020,#7188,.T.);
#14026=EDGE_CURVE('',#11019,#11017,#659,.T.);
#14027=EDGE_CURVE('',#11018,#11020,#660,.T.);
#14028=EDGE_CURVE('',#11021,#11022,#7189,.T.);
#14029=EDGE_CURVE('',#11021,#11019,#661,.T.);
#14030=EDGE_CURVE('',#11020,#11022,#662,.T.);
#14031=EDGE_CURVE('',#11023,#11024,#7190,.T.);
#14032=EDGE_CURVE('',#11023,#11021,#663,.T.);
#14033=EDGE_CURVE('',#11022,#11024,#664,.T.);
#14034=EDGE_CURVE('',#11025,#11026,#7191,.T.);
#14035=EDGE_CURVE('',#11025,#11023,#665,.T.);
#14036=EDGE_CURVE('',#11024,#11026,#666,.T.);
#14037=EDGE_CURVE('',#11027,#11028,#7192,.T.);
#14038=EDGE_CURVE('',#11027,#11025,#667,.T.);
#14039=EDGE_CURVE('',#11026,#11028,#668,.T.);
#14040=EDGE_CURVE('',#11029,#11030,#7193,.T.);
#14041=EDGE_CURVE('',#11029,#11027,#669,.T.);
#14042=EDGE_CURVE('',#11028,#11030,#670,.T.);
#14043=EDGE_CURVE('',#11031,#11032,#7194,.T.);
#14044=EDGE_CURVE('',#11031,#11033,#671,.T.);
#14045=EDGE_CURVE('',#11034,#11033,#5683,.T.);
#14046=EDGE_CURVE('',#11032,#11034,#672,.T.);
#14047=EDGE_CURVE('',#11035,#11036,#7195,.T.);
#14048=EDGE_CURVE('',#11035,#11031,#673,.T.);
#14049=EDGE_CURVE('',#11036,#11032,#674,.T.);
#14050=EDGE_CURVE('',#11037,#11038,#7196,.T.);
#14051=EDGE_CURVE('',#11037,#11035,#675,.T.);
#14052=EDGE_CURVE('',#11038,#11036,#676,.T.);
#14053=EDGE_CURVE('',#11039,#11040,#7197,.T.);
#14054=EDGE_CURVE('',#11039,#11037,#677,.T.);
#14055=EDGE_CURVE('',#11040,#11038,#678,.T.);
#14056=EDGE_CURVE('',#11041,#11042,#7198,.T.);
#14057=EDGE_CURVE('',#11041,#11039,#679,.T.);
#14058=EDGE_CURVE('',#11042,#11040,#680,.T.);
#14059=EDGE_CURVE('',#11043,#11044,#7199,.T.);
#14060=EDGE_CURVE('',#11043,#11041,#681,.T.);
#14061=EDGE_CURVE('',#11044,#11042,#682,.T.);
#14062=EDGE_CURVE('',#11045,#11046,#7200,.T.);
#14063=EDGE_CURVE('',#11045,#11043,#683,.T.);
#14064=EDGE_CURVE('',#11046,#11044,#684,.T.);
#14065=EDGE_CURVE('',#11047,#11048,#7201,.T.);
#14066=EDGE_CURVE('',#11047,#11045,#685,.T.);
#14067=EDGE_CURVE('',#11048,#11046,#686,.T.);
#14068=EDGE_CURVE('',#11049,#11050,#7202,.T.);
#14069=EDGE_CURVE('',#11049,#11047,#687,.T.);
#14070=EDGE_CURVE('',#11050,#11048,#688,.T.);
#14071=EDGE_CURVE('',#11051,#11052,#7203,.T.);
#14072=EDGE_CURVE('',#11051,#11049,#689,.T.);
#14073=EDGE_CURVE('',#11052,#11050,#690,.T.);
#14074=EDGE_CURVE('',#11053,#11054,#7204,.T.);
#14075=EDGE_CURVE('',#11053,#11051,#691,.T.);
#14076=EDGE_CURVE('',#11054,#11052,#692,.T.);
#14077=EDGE_CURVE('',#11055,#11056,#7205,.T.);
#14078=EDGE_CURVE('',#11055,#11053,#693,.T.);
#14079=EDGE_CURVE('',#11056,#11054,#694,.T.);
#14080=EDGE_CURVE('',#11057,#11058,#7206,.T.);
#14081=EDGE_CURVE('',#11057,#11055,#695,.T.);
#14082=EDGE_CURVE('',#11058,#11056,#696,.T.);
#14083=EDGE_CURVE('',#11059,#11060,#7207,.T.);
#14084=EDGE_CURVE('',#11059,#11057,#697,.T.);
#14085=EDGE_CURVE('',#11060,#11058,#698,.T.);
#14086=EDGE_CURVE('',#11061,#11062,#7208,.T.);
#14087=EDGE_CURVE('',#11061,#11059,#699,.T.);
#14088=EDGE_CURVE('',#11062,#11060,#700,.T.);
#14089=EDGE_CURVE('',#11063,#11064,#7209,.T.);
#14090=EDGE_CURVE('',#11063,#11061,#701,.T.);
#14091=EDGE_CURVE('',#11064,#11062,#702,.T.);
#14092=EDGE_CURVE('',#11065,#11066,#7210,.T.);
#14093=EDGE_CURVE('',#11065,#11063,#703,.T.);
#14094=EDGE_CURVE('',#11066,#11064,#704,.T.);
#14095=EDGE_CURVE('',#11067,#11068,#7211,.T.);
#14096=EDGE_CURVE('',#11067,#11065,#705,.T.);
#14097=EDGE_CURVE('',#11068,#11066,#706,.T.);
#14098=EDGE_CURVE('',#11069,#11070,#7212,.T.);
#14099=EDGE_CURVE('',#11069,#11067,#707,.T.);
#14100=EDGE_CURVE('',#11070,#11068,#708,.T.);
#14101=EDGE_CURVE('',#11071,#11072,#7213,.T.);
#14102=EDGE_CURVE('',#11071,#11069,#709,.T.);
#14103=EDGE_CURVE('',#11072,#11070,#710,.T.);
#14104=EDGE_CURVE('',#11073,#11074,#7214,.T.);
#14105=EDGE_CURVE('',#11073,#11071,#711,.T.);
#14106=EDGE_CURVE('',#11074,#11072,#712,.T.);
#14107=EDGE_CURVE('',#11075,#11076,#7215,.T.);
#14108=EDGE_CURVE('',#11075,#11073,#713,.T.);
#14109=EDGE_CURVE('',#11076,#11074,#714,.T.);
#14110=EDGE_CURVE('',#11077,#11078,#7216,.T.);
#14111=EDGE_CURVE('',#11077,#11075,#715,.T.);
#14112=EDGE_CURVE('',#11078,#11076,#716,.T.);
#14113=EDGE_CURVE('',#11079,#11080,#7217,.T.);
#14114=EDGE_CURVE('',#11079,#11077,#717,.T.);
#14115=EDGE_CURVE('',#11080,#11078,#718,.T.);
#14116=EDGE_CURVE('',#11081,#11082,#7218,.T.);
#14117=EDGE_CURVE('',#11081,#11079,#719,.T.);
#14118=EDGE_CURVE('',#11082,#11080,#720,.T.);
#14119=EDGE_CURVE('',#11083,#11084,#7219,.T.);
#14120=EDGE_CURVE('',#11083,#11081,#721,.T.);
#14121=EDGE_CURVE('',#11084,#11082,#722,.T.);
#14122=EDGE_CURVE('',#11085,#11086,#7220,.T.);
#14123=EDGE_CURVE('',#11085,#11083,#723,.T.);
#14124=EDGE_CURVE('',#11086,#11084,#724,.T.);
#14125=EDGE_CURVE('',#11087,#11088,#7221,.T.);
#14126=EDGE_CURVE('',#11087,#11085,#725,.T.);
#14127=EDGE_CURVE('',#11088,#11086,#726,.T.);
#14128=EDGE_CURVE('',#11089,#11090,#7222,.T.);
#14129=EDGE_CURVE('',#11089,#11087,#727,.T.);
#14130=EDGE_CURVE('',#11090,#11088,#728,.T.);
#14131=EDGE_CURVE('',#11091,#11092,#7223,.T.);
#14132=EDGE_CURVE('',#11091,#11089,#729,.T.);
#14133=EDGE_CURVE('',#11092,#11090,#730,.T.);
#14134=EDGE_CURVE('',#11093,#11094,#7224,.T.);
#14135=EDGE_CURVE('',#11093,#11091,#731,.T.);
#14136=EDGE_CURVE('',#11094,#11092,#732,.T.);
#14137=EDGE_CURVE('',#11095,#11096,#7225,.T.);
#14138=EDGE_CURVE('',#11095,#11093,#733,.T.);
#14139=EDGE_CURVE('',#11096,#11094,#734,.T.);
#14140=EDGE_CURVE('',#11097,#11098,#7226,.T.);
#14141=EDGE_CURVE('',#11097,#11095,#735,.T.);
#14142=EDGE_CURVE('',#11098,#11096,#736,.T.);
#14143=EDGE_CURVE('',#11099,#11100,#7227,.T.);
#14144=EDGE_CURVE('',#11099,#11097,#737,.T.);
#14145=EDGE_CURVE('',#11100,#11098,#738,.T.);
#14146=EDGE_CURVE('',#11101,#11102,#7228,.T.);
#14147=EDGE_CURVE('',#11101,#11099,#739,.T.);
#14148=EDGE_CURVE('',#11102,#11100,#740,.T.);
#14149=EDGE_CURVE('',#11103,#11104,#7229,.T.);
#14150=EDGE_CURVE('',#11103,#11101,#741,.T.);
#14151=EDGE_CURVE('',#11104,#11102,#742,.T.);
#14152=EDGE_CURVE('',#11105,#11106,#7230,.T.);
#14153=EDGE_CURVE('',#11105,#11103,#743,.T.);
#14154=EDGE_CURVE('',#11106,#11104,#744,.T.);
#14155=EDGE_CURVE('',#11107,#11108,#7231,.T.);
#14156=EDGE_CURVE('',#11107,#11105,#745,.T.);
#14157=EDGE_CURVE('',#11108,#11106,#746,.T.);
#14158=EDGE_CURVE('',#11109,#11110,#7232,.T.);
#14159=EDGE_CURVE('',#11109,#11107,#747,.T.);
#14160=EDGE_CURVE('',#11110,#11108,#748,.T.);
#14161=EDGE_CURVE('',#11111,#11112,#7233,.T.);
#14162=EDGE_CURVE('',#11111,#11109,#749,.T.);
#14163=EDGE_CURVE('',#11112,#11110,#750,.T.);
#14164=EDGE_CURVE('',#11113,#11114,#7234,.T.);
#14165=EDGE_CURVE('',#11113,#11111,#751,.T.);
#14166=EDGE_CURVE('',#11114,#11112,#752,.T.);
#14167=EDGE_CURVE('',#11115,#11116,#7235,.T.);
#14168=EDGE_CURVE('',#11115,#11113,#753,.T.);
#14169=EDGE_CURVE('',#11116,#11114,#754,.T.);
#14170=EDGE_CURVE('',#11117,#11118,#7236,.T.);
#14171=EDGE_CURVE('',#11117,#11115,#755,.T.);
#14172=EDGE_CURVE('',#11118,#11116,#756,.T.);
#14173=EDGE_CURVE('',#11119,#11120,#7237,.T.);
#14174=EDGE_CURVE('',#11119,#11117,#757,.T.);
#14175=EDGE_CURVE('',#11120,#11118,#758,.T.);
#14176=EDGE_CURVE('',#11121,#11122,#7238,.T.);
#14177=EDGE_CURVE('',#11121,#11119,#759,.T.);
#14178=EDGE_CURVE('',#11122,#11120,#760,.T.);
#14179=EDGE_CURVE('',#11123,#11124,#7239,.T.);
#14180=EDGE_CURVE('',#11123,#11121,#761,.T.);
#14181=EDGE_CURVE('',#11124,#11122,#762,.T.);
#14182=EDGE_CURVE('',#11125,#11126,#7240,.T.);
#14183=EDGE_CURVE('',#11125,#11123,#763,.T.);
#14184=EDGE_CURVE('',#11126,#11124,#764,.T.);
#14185=EDGE_CURVE('',#11127,#11128,#7241,.T.);
#14186=EDGE_CURVE('',#11127,#11125,#765,.T.);
#14187=EDGE_CURVE('',#11128,#11126,#766,.T.);
#14188=EDGE_CURVE('',#11129,#11130,#7242,.T.);
#14189=EDGE_CURVE('',#11129,#11127,#767,.T.);
#14190=EDGE_CURVE('',#11130,#11128,#768,.T.);
#14191=EDGE_CURVE('',#11131,#11132,#7243,.T.);
#14192=EDGE_CURVE('',#11131,#11129,#769,.T.);
#14193=EDGE_CURVE('',#11132,#11130,#770,.T.);
#14194=EDGE_CURVE('',#11133,#11134,#7244,.T.);
#14195=EDGE_CURVE('',#11133,#11131,#771,.T.);
#14196=EDGE_CURVE('',#11134,#11132,#772,.T.);
#14197=EDGE_CURVE('',#11135,#11136,#7245,.T.);
#14198=EDGE_CURVE('',#11135,#11133,#773,.T.);
#14199=EDGE_CURVE('',#11136,#11134,#774,.T.);
#14200=EDGE_CURVE('',#11137,#11138,#7246,.T.);
#14201=EDGE_CURVE('',#11137,#11135,#775,.T.);
#14202=EDGE_CURVE('',#11138,#11136,#776,.T.);
#14203=EDGE_CURVE('',#11139,#11140,#7247,.T.);
#14204=EDGE_CURVE('',#11139,#11137,#777,.T.);
#14205=EDGE_CURVE('',#11140,#11138,#778,.T.);
#14206=EDGE_CURVE('',#11141,#11142,#7248,.T.);
#14207=EDGE_CURVE('',#11141,#11139,#779,.T.);
#14208=EDGE_CURVE('',#11142,#11140,#780,.T.);
#14209=EDGE_CURVE('',#11143,#11144,#7249,.T.);
#14210=EDGE_CURVE('',#11143,#11141,#781,.T.);
#14211=EDGE_CURVE('',#11144,#11142,#782,.T.);
#14212=EDGE_CURVE('',#11145,#11146,#7250,.T.);
#14213=EDGE_CURVE('',#11145,#11143,#783,.T.);
#14214=EDGE_CURVE('',#11146,#11144,#784,.T.);
#14215=EDGE_CURVE('',#11147,#11148,#7251,.T.);
#14216=EDGE_CURVE('',#11147,#11145,#785,.T.);
#14217=EDGE_CURVE('',#11148,#11146,#786,.T.);
#14218=EDGE_CURVE('',#11149,#11150,#7252,.T.);
#14219=EDGE_CURVE('',#11149,#11147,#787,.T.);
#14220=EDGE_CURVE('',#11150,#11148,#788,.T.);
#14221=EDGE_CURVE('',#11033,#11151,#789,.T.);
#14222=EDGE_CURVE('',#11152,#11151,#5684,.T.);
#14223=EDGE_CURVE('',#11153,#11152,#5685,.T.);
#14224=EDGE_CURVE('',#11153,#11034,#790,.T.);
#14225=EDGE_CURVE('',#11030,#11153,#791,.T.);
#14226=EDGE_CURVE('',#11154,#10916,#792,.T.);
#14227=EDGE_CURVE('',#11154,#11150,#793,.T.);
#14228=EDGE_CURVE('',#10913,#11155,#794,.T.);
#14229=EDGE_CURVE('',#11155,#11154,#5686,.T.);
#14230=EDGE_CURVE('',#11155,#11149,#795,.T.);
#14231=EDGE_CURVE('',#11151,#11029,#796,.T.);
#14232=EDGE_CURVE('',#11156,#11157,#5687,.T.);
#14233=EDGE_CURVE('',#11156,#11158,#7253,.T.);
#14234=EDGE_CURVE('',#11158,#11157,#7254,.T.);
#14235=EDGE_CURVE('',#11157,#11159,#7255,.T.);
#14236=EDGE_CURVE('',#11158,#11160,#7256,.T.);
#14237=EDGE_CURVE('',#11159,#11160,#219,.T.);
#14238=EDGE_CURVE('',#11161,#11156,#7257,.T.);
#14239=EDGE_CURVE('',#11160,#11161,#220,.T.);
#14240=EDGE_CURVE('',#11162,#11163,#5688,.T.);
#14241=EDGE_CURVE('',#11162,#11164,#7258,.T.);
#14242=EDGE_CURVE('',#11164,#11163,#7259,.T.);
#14243=EDGE_CURVE('',#11163,#11165,#7260,.T.);
#14244=EDGE_CURVE('',#11164,#11166,#7261,.T.);
#14245=EDGE_CURVE('',#11165,#11166,#221,.T.);
#14246=EDGE_CURVE('',#11167,#11162,#7262,.T.);
#14247=EDGE_CURVE('',#11166,#11167,#222,.T.);
#14248=EDGE_CURVE('',#11168,#11169,#5689,.T.);
#14249=EDGE_CURVE('',#11168,#11170,#7263,.T.);
#14250=EDGE_CURVE('',#11170,#11169,#7264,.T.);
#14251=EDGE_CURVE('',#11169,#11171,#7265,.T.);
#14252=EDGE_CURVE('',#11170,#11172,#7266,.T.);
#14253=EDGE_CURVE('',#11171,#11172,#223,.T.);
#14254=EDGE_CURVE('',#11173,#11168,#7267,.T.);
#14255=EDGE_CURVE('',#11172,#11173,#224,.T.);
#14256=EDGE_CURVE('',#11174,#11175,#5690,.T.);
#14257=EDGE_CURVE('',#11174,#11176,#7268,.T.);
#14258=EDGE_CURVE('',#11176,#11175,#7269,.T.);
#14259=EDGE_CURVE('',#11175,#11177,#7270,.T.);
#14260=EDGE_CURVE('',#11176,#11178,#7271,.T.);
#14261=EDGE_CURVE('',#11177,#11178,#225,.T.);
#14262=EDGE_CURVE('',#11179,#11174,#7272,.T.);
#14263=EDGE_CURVE('',#11178,#11179,#226,.T.);
#14264=EDGE_CURVE('',#11180,#11181,#5691,.T.);
#14265=EDGE_CURVE('',#11180,#11182,#7273,.T.);
#14266=EDGE_CURVE('',#11182,#11181,#7274,.T.);
#14267=EDGE_CURVE('',#11181,#11183,#7275,.T.);
#14268=EDGE_CURVE('',#11182,#11184,#7276,.T.);
#14269=EDGE_CURVE('',#11183,#11184,#227,.T.);
#14270=EDGE_CURVE('',#11185,#11180,#7277,.T.);
#14271=EDGE_CURVE('',#11184,#11185,#228,.T.);
#14272=EDGE_CURVE('',#11186,#11187,#5692,.T.);
#14273=EDGE_CURVE('',#11186,#11188,#7278,.T.);
#14274=EDGE_CURVE('',#11188,#11187,#7279,.T.);
#14275=EDGE_CURVE('',#11187,#11189,#7280,.T.);
#14276=EDGE_CURVE('',#11188,#11190,#7281,.T.);
#14277=EDGE_CURVE('',#11189,#11190,#229,.T.);
#14278=EDGE_CURVE('',#11191,#11186,#7282,.T.);
#14279=EDGE_CURVE('',#11190,#11191,#230,.T.);
#14280=EDGE_CURVE('',#11192,#11193,#5693,.T.);
#14281=EDGE_CURVE('',#11192,#11194,#7283,.T.);
#14282=EDGE_CURVE('',#11194,#11193,#7284,.T.);
#14283=EDGE_CURVE('',#11193,#11195,#7285,.T.);
#14284=EDGE_CURVE('',#11194,#11196,#7286,.T.);
#14285=EDGE_CURVE('',#11195,#11196,#231,.T.);
#14286=EDGE_CURVE('',#11197,#11192,#7287,.T.);
#14287=EDGE_CURVE('',#11196,#11197,#232,.T.);
#14288=EDGE_CURVE('',#11198,#11199,#5694,.T.);
#14289=EDGE_CURVE('',#11198,#11200,#7288,.T.);
#14290=EDGE_CURVE('',#11200,#11199,#7289,.T.);
#14291=EDGE_CURVE('',#11199,#11201,#7290,.T.);
#14292=EDGE_CURVE('',#11200,#11202,#7291,.T.);
#14293=EDGE_CURVE('',#11201,#11202,#233,.T.);
#14294=EDGE_CURVE('',#11203,#11198,#7292,.T.);
#14295=EDGE_CURVE('',#11202,#11203,#234,.T.);
#14296=EDGE_CURVE('',#11204,#11205,#5695,.T.);
#14297=EDGE_CURVE('',#11204,#11206,#7293,.T.);
#14298=EDGE_CURVE('',#11206,#11205,#7294,.T.);
#14299=EDGE_CURVE('',#11205,#11207,#7295,.T.);
#14300=EDGE_CURVE('',#11206,#11208,#7296,.T.);
#14301=EDGE_CURVE('',#11207,#11208,#235,.T.);
#14302=EDGE_CURVE('',#11209,#11204,#7297,.T.);
#14303=EDGE_CURVE('',#11208,#11209,#236,.T.);
#14304=EDGE_CURVE('',#11210,#11211,#5696,.T.);
#14305=EDGE_CURVE('',#11210,#11212,#7298,.T.);
#14306=EDGE_CURVE('',#11212,#11211,#7299,.T.);
#14307=EDGE_CURVE('',#11211,#11213,#7300,.T.);
#14308=EDGE_CURVE('',#11212,#11214,#7301,.T.);
#14309=EDGE_CURVE('',#11213,#11214,#237,.T.);
#14310=EDGE_CURVE('',#11215,#11210,#7302,.T.);
#14311=EDGE_CURVE('',#11214,#11215,#238,.T.);
#14312=EDGE_CURVE('',#11216,#11217,#5697,.T.);
#14313=EDGE_CURVE('',#11216,#11218,#7303,.T.);
#14314=EDGE_CURVE('',#11218,#11217,#7304,.T.);
#14315=EDGE_CURVE('',#11217,#11219,#7305,.T.);
#14316=EDGE_CURVE('',#11218,#11220,#7306,.T.);
#14317=EDGE_CURVE('',#11219,#11220,#239,.T.);
#14318=EDGE_CURVE('',#11221,#11216,#7307,.T.);
#14319=EDGE_CURVE('',#11220,#11221,#240,.T.);
#14320=EDGE_CURVE('',#11222,#11223,#5698,.T.);
#14321=EDGE_CURVE('',#11222,#11224,#7308,.T.);
#14322=EDGE_CURVE('',#11224,#11223,#7309,.T.);
#14323=EDGE_CURVE('',#11223,#11225,#7310,.T.);
#14324=EDGE_CURVE('',#11224,#11226,#7311,.T.);
#14325=EDGE_CURVE('',#11225,#11226,#241,.T.);
#14326=EDGE_CURVE('',#11227,#11222,#7312,.T.);
#14327=EDGE_CURVE('',#11226,#11227,#242,.T.);
#14328=EDGE_CURVE('',#11228,#11229,#5699,.T.);
#14329=EDGE_CURVE('',#11228,#11230,#7313,.T.);
#14330=EDGE_CURVE('',#11230,#11229,#7314,.T.);
#14331=EDGE_CURVE('',#11229,#11231,#7315,.T.);
#14332=EDGE_CURVE('',#11230,#11232,#7316,.T.);
#14333=EDGE_CURVE('',#11231,#11232,#243,.T.);
#14334=EDGE_CURVE('',#11233,#11228,#7317,.T.);
#14335=EDGE_CURVE('',#11232,#11233,#244,.T.);
#14336=EDGE_CURVE('',#11234,#11235,#5700,.T.);
#14337=EDGE_CURVE('',#11234,#11236,#7318,.T.);
#14338=EDGE_CURVE('',#11236,#11235,#7319,.T.);
#14339=EDGE_CURVE('',#11235,#11237,#7320,.T.);
#14340=EDGE_CURVE('',#11236,#11238,#7321,.T.);
#14341=EDGE_CURVE('',#11237,#11238,#245,.T.);
#14342=EDGE_CURVE('',#11239,#11234,#7322,.T.);
#14343=EDGE_CURVE('',#11238,#11239,#246,.T.);
#14344=EDGE_CURVE('',#11240,#11241,#5701,.T.);
#14345=EDGE_CURVE('',#11240,#11242,#7323,.T.);
#14346=EDGE_CURVE('',#11242,#11241,#7324,.T.);
#14347=EDGE_CURVE('',#11241,#11243,#7325,.T.);
#14348=EDGE_CURVE('',#11242,#11244,#7326,.T.);
#14349=EDGE_CURVE('',#11243,#11244,#247,.T.);
#14350=EDGE_CURVE('',#11245,#11240,#7327,.T.);
#14351=EDGE_CURVE('',#11244,#11245,#248,.T.);
#14352=EDGE_CURVE('',#11246,#11247,#5702,.T.);
#14353=EDGE_CURVE('',#11246,#11248,#7328,.T.);
#14354=EDGE_CURVE('',#11248,#11247,#7329,.T.);
#14355=EDGE_CURVE('',#11247,#11249,#7330,.T.);
#14356=EDGE_CURVE('',#11248,#11250,#7331,.T.);
#14357=EDGE_CURVE('',#11249,#11250,#249,.T.);
#14358=EDGE_CURVE('',#11251,#11246,#7332,.T.);
#14359=EDGE_CURVE('',#11250,#11251,#250,.T.);
#14360=EDGE_CURVE('',#11252,#11253,#5703,.T.);
#14361=EDGE_CURVE('',#11252,#11254,#7333,.T.);
#14362=EDGE_CURVE('',#11254,#11253,#7334,.T.);
#14363=EDGE_CURVE('',#11253,#11255,#7335,.T.);
#14364=EDGE_CURVE('',#11254,#11256,#7336,.T.);
#14365=EDGE_CURVE('',#11255,#11256,#251,.T.);
#14366=EDGE_CURVE('',#11257,#11252,#7337,.T.);
#14367=EDGE_CURVE('',#11256,#11257,#252,.T.);
#14368=EDGE_CURVE('',#11258,#11259,#5704,.T.);
#14369=EDGE_CURVE('',#11258,#11260,#7338,.T.);
#14370=EDGE_CURVE('',#11260,#11261,#7339,.T.);
#14371=EDGE_CURVE('',#11259,#11261,#5705,.T.);
#14372=EDGE_CURVE('',#11261,#11262,#7340,.T.);
#14373=EDGE_CURVE('',#11260,#11263,#7341,.T.);
#14374=EDGE_CURVE('',#11262,#11263,#253,.T.);
#14375=EDGE_CURVE('',#11264,#11258,#7342,.T.);
#14376=EDGE_CURVE('',#11263,#11264,#254,.T.);
#14377=EDGE_CURVE('',#11265,#11266,#5706,.T.);
#14378=EDGE_CURVE('',#11265,#11267,#7343,.T.);
#14379=EDGE_CURVE('',#11267,#11266,#7344,.T.);
#14380=EDGE_CURVE('',#11266,#11268,#7345,.T.);
#14381=EDGE_CURVE('',#11267,#11269,#7346,.T.);
#14382=EDGE_CURVE('',#11268,#11269,#255,.T.);
#14383=EDGE_CURVE('',#11270,#11265,#7347,.T.);
#14384=EDGE_CURVE('',#11269,#11270,#256,.T.);
#14385=EDGE_CURVE('',#11271,#11272,#5707,.T.);
#14386=EDGE_CURVE('',#11271,#11273,#7348,.T.);
#14387=EDGE_CURVE('',#11273,#11272,#7349,.T.);
#14388=EDGE_CURVE('',#11272,#11274,#7350,.T.);
#14389=EDGE_CURVE('',#11273,#11275,#7351,.T.);
#14390=EDGE_CURVE('',#11274,#11275,#257,.T.);
#14391=EDGE_CURVE('',#11276,#11271,#7352,.T.);
#14392=EDGE_CURVE('',#11275,#11276,#258,.T.);
#14393=EDGE_CURVE('',#11277,#11278,#5708,.T.);
#14394=EDGE_CURVE('',#11277,#11279,#7353,.T.);
#14395=EDGE_CURVE('',#11279,#11278,#7354,.T.);
#14396=EDGE_CURVE('',#11278,#11280,#7355,.T.);
#14397=EDGE_CURVE('',#11279,#11281,#7356,.T.);
#14398=EDGE_CURVE('',#11280,#11281,#259,.T.);
#14399=EDGE_CURVE('',#11282,#11277,#7357,.T.);
#14400=EDGE_CURVE('',#11281,#11282,#260,.T.);
#14401=EDGE_CURVE('',#11283,#11284,#5709,.T.);
#14402=EDGE_CURVE('',#11283,#11285,#7358,.T.);
#14403=EDGE_CURVE('',#11285,#11284,#7359,.T.);
#14404=EDGE_CURVE('',#11284,#11286,#7360,.T.);
#14405=EDGE_CURVE('',#11285,#11287,#7361,.T.);
#14406=EDGE_CURVE('',#11286,#11287,#261,.T.);
#14407=EDGE_CURVE('',#11288,#11283,#7362,.T.);
#14408=EDGE_CURVE('',#11287,#11288,#262,.T.);
#14409=EDGE_CURVE('',#11289,#11290,#5710,.T.);
#14410=EDGE_CURVE('',#11289,#11291,#7363,.T.);
#14411=EDGE_CURVE('',#11291,#11290,#7364,.T.);
#14412=EDGE_CURVE('',#11290,#11292,#7365,.T.);
#14413=EDGE_CURVE('',#11291,#11293,#7366,.T.);
#14414=EDGE_CURVE('',#11292,#11293,#263,.T.);
#14415=EDGE_CURVE('',#11294,#11289,#7367,.T.);
#14416=EDGE_CURVE('',#11293,#11294,#264,.T.);
#14417=EDGE_CURVE('',#11295,#11296,#5711,.T.);
#14418=EDGE_CURVE('',#11295,#11297,#7368,.T.);
#14419=EDGE_CURVE('',#11297,#11296,#7369,.T.);
#14420=EDGE_CURVE('',#11296,#11298,#7370,.T.);
#14421=EDGE_CURVE('',#11297,#11299,#7371,.T.);
#14422=EDGE_CURVE('',#11298,#11299,#265,.T.);
#14423=EDGE_CURVE('',#11300,#11295,#7372,.T.);
#14424=EDGE_CURVE('',#11299,#11300,#266,.T.);
#14425=EDGE_CURVE('',#11301,#11302,#5712,.T.);
#14426=EDGE_CURVE('',#11301,#11303,#7373,.T.);
#14427=EDGE_CURVE('',#11303,#11302,#7374,.T.);
#14428=EDGE_CURVE('',#11302,#11304,#7375,.T.);
#14429=EDGE_CURVE('',#11303,#11305,#7376,.T.);
#14430=EDGE_CURVE('',#11304,#11305,#267,.T.);
#14431=EDGE_CURVE('',#11306,#11301,#7377,.T.);
#14432=EDGE_CURVE('',#11305,#11306,#268,.T.);
#14433=EDGE_CURVE('',#11307,#11308,#5713,.T.);
#14434=EDGE_CURVE('',#11307,#11309,#7378,.T.);
#14435=EDGE_CURVE('',#11309,#11308,#7379,.T.);
#14436=EDGE_CURVE('',#11308,#11310,#7380,.T.);
#14437=EDGE_CURVE('',#11309,#11311,#7381,.T.);
#14438=EDGE_CURVE('',#11310,#11311,#269,.T.);
#14439=EDGE_CURVE('',#11312,#11307,#7382,.T.);
#14440=EDGE_CURVE('',#11311,#11312,#270,.T.);
#14441=EDGE_CURVE('',#11313,#11314,#5714,.T.);
#14442=EDGE_CURVE('',#11313,#11315,#7383,.T.);
#14443=EDGE_CURVE('',#11315,#11314,#7384,.T.);
#14444=EDGE_CURVE('',#11314,#11316,#7385,.T.);
#14445=EDGE_CURVE('',#11315,#11317,#7386,.T.);
#14446=EDGE_CURVE('',#11316,#11317,#271,.T.);
#14447=EDGE_CURVE('',#11318,#11313,#7387,.T.);
#14448=EDGE_CURVE('',#11317,#11318,#272,.T.);
#14449=EDGE_CURVE('',#11319,#11320,#5715,.T.);
#14450=EDGE_CURVE('',#11319,#11321,#7388,.T.);
#14451=EDGE_CURVE('',#11321,#11320,#7389,.T.);
#14452=EDGE_CURVE('',#11320,#11322,#7390,.T.);
#14453=EDGE_CURVE('',#11321,#11323,#7391,.T.);
#14454=EDGE_CURVE('',#11322,#11323,#273,.T.);
#14455=EDGE_CURVE('',#11324,#11319,#7392,.T.);
#14456=EDGE_CURVE('',#11323,#11324,#274,.T.);
#14457=EDGE_CURVE('',#11325,#11326,#5716,.T.);
#14458=EDGE_CURVE('',#11325,#11327,#7393,.T.);
#14459=EDGE_CURVE('',#11327,#11326,#7394,.T.);
#14460=EDGE_CURVE('',#11326,#11328,#7395,.T.);
#14461=EDGE_CURVE('',#11327,#11329,#7396,.T.);
#14462=EDGE_CURVE('',#11328,#11329,#275,.T.);
#14463=EDGE_CURVE('',#11330,#11325,#7397,.T.);
#14464=EDGE_CURVE('',#11329,#11330,#276,.T.);
#14465=EDGE_CURVE('',#11331,#11332,#5717,.T.);
#14466=EDGE_CURVE('',#11331,#11333,#7398,.T.);
#14467=EDGE_CURVE('',#11333,#11332,#7399,.T.);
#14468=EDGE_CURVE('',#11332,#11334,#7400,.T.);
#14469=EDGE_CURVE('',#11333,#11335,#7401,.T.);
#14470=EDGE_CURVE('',#11334,#11335,#277,.T.);
#14471=EDGE_CURVE('',#11336,#11331,#7402,.T.);
#14472=EDGE_CURVE('',#11335,#11336,#278,.T.);
#14473=EDGE_CURVE('',#11337,#11338,#5718,.T.);
#14474=EDGE_CURVE('',#11337,#11339,#7403,.T.);
#14475=EDGE_CURVE('',#11339,#11338,#7404,.T.);
#14476=EDGE_CURVE('',#11338,#11340,#7405,.T.);
#14477=EDGE_CURVE('',#11339,#11341,#7406,.T.);
#14478=EDGE_CURVE('',#11340,#11341,#279,.T.);
#14479=EDGE_CURVE('',#11342,#11337,#7407,.T.);
#14480=EDGE_CURVE('',#11341,#11342,#280,.T.);
#14481=EDGE_CURVE('',#11343,#11344,#5719,.T.);
#14482=EDGE_CURVE('',#11343,#11345,#7408,.T.);
#14483=EDGE_CURVE('',#11345,#11344,#7409,.T.);
#14484=EDGE_CURVE('',#11344,#11346,#7410,.T.);
#14485=EDGE_CURVE('',#11345,#11347,#7411,.T.);
#14486=EDGE_CURVE('',#11346,#11347,#281,.T.);
#14487=EDGE_CURVE('',#11348,#11343,#7412,.T.);
#14488=EDGE_CURVE('',#11347,#11348,#282,.T.);
#14489=EDGE_CURVE('',#11349,#11350,#5720,.T.);
#14490=EDGE_CURVE('',#11349,#11351,#7413,.T.);
#14491=EDGE_CURVE('',#11351,#11350,#7414,.T.);
#14492=EDGE_CURVE('',#11350,#11352,#7415,.T.);
#14493=EDGE_CURVE('',#11351,#11353,#7416,.T.);
#14494=EDGE_CURVE('',#11352,#11353,#283,.T.);
#14495=EDGE_CURVE('',#11354,#11349,#7417,.T.);
#14496=EDGE_CURVE('',#11353,#11354,#284,.T.);
#14497=EDGE_CURVE('',#11355,#11356,#5721,.T.);
#14498=EDGE_CURVE('',#11355,#11357,#7418,.T.);
#14499=EDGE_CURVE('',#11357,#11356,#7419,.T.);
#14500=EDGE_CURVE('',#11356,#11358,#7420,.T.);
#14501=EDGE_CURVE('',#11357,#11359,#7421,.T.);
#14502=EDGE_CURVE('',#11358,#11359,#285,.T.);
#14503=EDGE_CURVE('',#11360,#11355,#7422,.T.);
#14504=EDGE_CURVE('',#11359,#11360,#286,.T.);
#14505=EDGE_CURVE('',#11361,#11362,#5722,.T.);
#14506=EDGE_CURVE('',#11361,#11363,#7423,.T.);
#14507=EDGE_CURVE('',#11363,#11362,#7424,.T.);
#14508=EDGE_CURVE('',#11362,#11364,#7425,.T.);
#14509=EDGE_CURVE('',#11363,#11365,#7426,.T.);
#14510=EDGE_CURVE('',#11364,#11365,#287,.T.);
#14511=EDGE_CURVE('',#11366,#11361,#7427,.T.);
#14512=EDGE_CURVE('',#11365,#11366,#288,.T.);
#14513=EDGE_CURVE('',#11167,#11159,#5723,.T.);
#14514=EDGE_CURVE('',#11173,#11165,#5724,.T.);
#14515=EDGE_CURVE('',#11179,#11171,#5725,.T.);
#14516=EDGE_CURVE('',#11185,#11177,#5726,.T.);
#14517=EDGE_CURVE('',#11191,#11183,#5727,.T.);
#14518=EDGE_CURVE('',#11197,#11189,#5728,.T.);
#14519=EDGE_CURVE('',#11203,#11195,#5729,.T.);
#14520=EDGE_CURVE('',#11209,#11201,#5730,.T.);
#14521=EDGE_CURVE('',#11215,#11207,#5731,.T.);
#14522=EDGE_CURVE('',#11221,#11213,#5732,.T.);
#14523=EDGE_CURVE('',#11227,#11219,#5733,.T.);
#14524=EDGE_CURVE('',#11233,#11225,#5734,.T.);
#14525=EDGE_CURVE('',#11239,#11231,#5735,.T.);
#14526=EDGE_CURVE('',#11245,#11237,#5736,.T.);
#14527=EDGE_CURVE('',#11251,#11243,#5737,.T.);
#14528=EDGE_CURVE('',#11257,#11249,#5738,.T.);
#14529=EDGE_CURVE('',#11264,#11255,#5739,.T.);
#14530=EDGE_CURVE('',#11259,#11367,#7428,.T.);
#14531=EDGE_CURVE('',#11367,#11367,#5740,.T.);
#14532=EDGE_CURVE('',#11270,#11262,#5741,.T.);
#14533=EDGE_CURVE('',#11276,#11268,#5742,.T.);
#14534=EDGE_CURVE('',#11282,#11274,#5743,.T.);
#14535=EDGE_CURVE('',#11288,#11280,#5744,.T.);
#14536=EDGE_CURVE('',#11294,#11286,#5745,.T.);
#14537=EDGE_CURVE('',#11300,#11292,#5746,.T.);
#14538=EDGE_CURVE('',#11306,#11298,#5747,.T.);
#14539=EDGE_CURVE('',#11312,#11304,#5748,.T.);
#14540=EDGE_CURVE('',#11318,#11310,#5749,.T.);
#14541=EDGE_CURVE('',#11324,#11316,#5750,.T.);
#14542=EDGE_CURVE('',#11330,#11322,#5751,.T.);
#14543=EDGE_CURVE('',#11336,#11328,#5752,.T.);
#14544=EDGE_CURVE('',#11342,#11334,#5753,.T.);
#14545=EDGE_CURVE('',#11348,#11340,#5754,.T.);
#14546=EDGE_CURVE('',#11354,#11346,#5755,.T.);
#14547=EDGE_CURVE('',#11360,#11352,#5756,.T.);
#14548=EDGE_CURVE('',#11366,#11358,#5757,.T.);
#14549=EDGE_CURVE('',#11368,#11364,#5758,.T.);
#14550=EDGE_CURVE('',#11368,#11369,#7429,.T.);
#14551=EDGE_CURVE('',#11369,#11370,#5759,.T.);
#14552=EDGE_CURVE('',#11370,#11371,#7430,.T.);
#14553=EDGE_CURVE('',#11161,#11371,#5760,.T.);
#14554=EDGE_CURVE('',#11372,#11370,#7431,.T.);
#14555=EDGE_CURVE('',#11372,#11373,#7432,.T.);
#14556=EDGE_CURVE('',#11371,#11373,#289,.T.);
#14557=EDGE_CURVE('',#11373,#11368,#290,.T.);
#14558=EDGE_CURVE('',#11369,#11372,#7433,.T.);
#14559=EDGE_CURVE('',#11374,#11374,#5761,.T.);
#14560=EDGE_CURVE('',#11374,#11263,#7434,.T.);
#14561=EDGE_CURVE('',#11375,#11376,#7435,.T.);
#14562=EDGE_CURVE('',#11376,#11376,#5762,.T.);
#14563=EDGE_CURVE('',#11377,#11378,#7436,.T.);
#14564=EDGE_CURVE('',#11377,#11379,#7437,.T.);
#14565=EDGE_CURVE('',#11379,#11380,#7438,.T.);
#14566=EDGE_CURVE('',#11378,#11380,#7439,.T.);
#14567=EDGE_CURVE('',#11381,#11377,#7440,.T.);
#14568=EDGE_CURVE('',#11381,#11382,#7441,.T.);
#14569=EDGE_CURVE('',#11382,#11379,#7442,.T.);
#14570=EDGE_CURVE('',#11383,#11381,#7443,.T.);
#14571=EDGE_CURVE('',#11383,#11384,#7444,.T.);
#14572=EDGE_CURVE('',#11384,#11382,#7445,.T.);
#14573=EDGE_CURVE('',#11385,#11383,#7446,.T.);
#14574=EDGE_CURVE('',#11385,#11386,#7447,.T.);
#14575=EDGE_CURVE('',#11386,#11384,#7448,.T.);
#14576=EDGE_CURVE('',#11387,#11385,#7449,.T.);
#14577=EDGE_CURVE('',#11387,#11388,#7450,.T.);
#14578=EDGE_CURVE('',#11388,#11386,#7451,.T.);
#14579=EDGE_CURVE('',#11378,#11387,#7452,.T.);
#14580=EDGE_CURVE('',#11380,#11388,#7453,.T.);
#14581=EDGE_CURVE('',#11389,#11389,#5763,.T.);
#14582=EDGE_CURVE('',#10915,#11389,#7454,.T.);
#14583=EDGE_CURVE('',#11151,#11153,#5764,.T.);
#14584=EDGE_CURVE('',#11390,#11390,#5765,.T.);
#14585=EDGE_CURVE('',#11390,#11152,#7455,.T.);
#19375=ORIENTED_EDGE('',*,*,#13865,.F.);
#19376=ORIENTED_EDGE('',*,*,#13866,.T.);
#19377=ORIENTED_EDGE('',*,*,#13867,.T.);
#19378=ORIENTED_EDGE('',*,*,#13868,.T.);
#19379=ORIENTED_EDGE('',*,*,#13869,.T.);
#19380=ORIENTED_EDGE('',*,*,#13868,.F.);
#19381=ORIENTED_EDGE('',*,*,#13870,.T.);
#19382=ORIENTED_EDGE('',*,*,#13871,.T.);
#19383=ORIENTED_EDGE('',*,*,#13872,.F.);
#19384=ORIENTED_EDGE('',*,*,#13873,.T.);
#19385=ORIENTED_EDGE('',*,*,#13865,.T.);
#19386=ORIENTED_EDGE('',*,*,#13874,.T.);
#19387=ORIENTED_EDGE('',*,*,#13875,.F.);
#19388=ORIENTED_EDGE('',*,*,#13876,.T.);
#19389=ORIENTED_EDGE('',*,*,#13872,.T.);
#19390=ORIENTED_EDGE('',*,*,#13877,.T.);
#19391=ORIENTED_EDGE('',*,*,#13878,.F.);
#19392=ORIENTED_EDGE('',*,*,#13879,.T.);
#19393=ORIENTED_EDGE('',*,*,#13875,.T.);
#19394=ORIENTED_EDGE('',*,*,#13880,.T.);
#19395=ORIENTED_EDGE('',*,*,#13881,.F.);
#19396=ORIENTED_EDGE('',*,*,#13882,.T.);
#19397=ORIENTED_EDGE('',*,*,#13878,.T.);
#19398=ORIENTED_EDGE('',*,*,#13883,.T.);
#19399=ORIENTED_EDGE('',*,*,#13884,.F.);
#19400=ORIENTED_EDGE('',*,*,#13885,.T.);
#19401=ORIENTED_EDGE('',*,*,#13881,.T.);
#19402=ORIENTED_EDGE('',*,*,#13886,.T.);
#19403=ORIENTED_EDGE('',*,*,#13887,.F.);
#19404=ORIENTED_EDGE('',*,*,#13888,.T.);
#19405=ORIENTED_EDGE('',*,*,#13884,.T.);
#19406=ORIENTED_EDGE('',*,*,#13889,.T.);
#19407=ORIENTED_EDGE('',*,*,#13890,.F.);
#19408=ORIENTED_EDGE('',*,*,#13891,.T.);
#19409=ORIENTED_EDGE('',*,*,#13887,.T.);
#19410=ORIENTED_EDGE('',*,*,#13892,.T.);
#19411=ORIENTED_EDGE('',*,*,#13893,.F.);
#19412=ORIENTED_EDGE('',*,*,#13894,.T.);
#19413=ORIENTED_EDGE('',*,*,#13890,.T.);
#19414=ORIENTED_EDGE('',*,*,#13895,.T.);
#19415=ORIENTED_EDGE('',*,*,#13896,.F.);
#19416=ORIENTED_EDGE('',*,*,#13897,.T.);
#19417=ORIENTED_EDGE('',*,*,#13893,.T.);
#19418=ORIENTED_EDGE('',*,*,#13898,.T.);
#19419=ORIENTED_EDGE('',*,*,#13899,.F.);
#19420=ORIENTED_EDGE('',*,*,#13900,.T.);
#19421=ORIENTED_EDGE('',*,*,#13896,.T.);
#19422=ORIENTED_EDGE('',*,*,#13901,.T.);
#19423=ORIENTED_EDGE('',*,*,#13902,.F.);
#19424=ORIENTED_EDGE('',*,*,#13903,.T.);
#19425=ORIENTED_EDGE('',*,*,#13899,.T.);
#19426=ORIENTED_EDGE('',*,*,#13904,.T.);
#19427=ORIENTED_EDGE('',*,*,#13905,.F.);
#19428=ORIENTED_EDGE('',*,*,#13906,.T.);
#19429=ORIENTED_EDGE('',*,*,#13902,.T.);
#19430=ORIENTED_EDGE('',*,*,#13907,.T.);
#19431=ORIENTED_EDGE('',*,*,#13908,.F.);
#19432=ORIENTED_EDGE('',*,*,#13909,.T.);
#19433=ORIENTED_EDGE('',*,*,#13905,.T.);
#19434=ORIENTED_EDGE('',*,*,#13910,.T.);
#19435=ORIENTED_EDGE('',*,*,#13911,.F.);
#19436=ORIENTED_EDGE('',*,*,#13912,.T.);
#19437=ORIENTED_EDGE('',*,*,#13908,.T.);
#19438=ORIENTED_EDGE('',*,*,#13913,.T.);
#19439=ORIENTED_EDGE('',*,*,#13914,.F.);
#19440=ORIENTED_EDGE('',*,*,#13915,.T.);
#19441=ORIENTED_EDGE('',*,*,#13911,.T.);
#19442=ORIENTED_EDGE('',*,*,#13916,.T.);
#19443=ORIENTED_EDGE('',*,*,#13917,.F.);
#19444=ORIENTED_EDGE('',*,*,#13918,.T.);
#19445=ORIENTED_EDGE('',*,*,#13914,.T.);
#19446=ORIENTED_EDGE('',*,*,#13919,.T.);
#19447=ORIENTED_EDGE('',*,*,#13920,.F.);
#19448=ORIENTED_EDGE('',*,*,#13921,.T.);
#19449=ORIENTED_EDGE('',*,*,#13917,.T.);
#19450=ORIENTED_EDGE('',*,*,#13922,.T.);
#19451=ORIENTED_EDGE('',*,*,#13923,.F.);
#19452=ORIENTED_EDGE('',*,*,#13924,.T.);
#19453=ORIENTED_EDGE('',*,*,#13920,.T.);
#19454=ORIENTED_EDGE('',*,*,#13925,.T.);
#19455=ORIENTED_EDGE('',*,*,#13926,.F.);
#19456=ORIENTED_EDGE('',*,*,#13927,.T.);
#19457=ORIENTED_EDGE('',*,*,#13923,.T.);
#19458=ORIENTED_EDGE('',*,*,#13928,.T.);
#19459=ORIENTED_EDGE('',*,*,#13929,.F.);
#19460=ORIENTED_EDGE('',*,*,#13930,.T.);
#19461=ORIENTED_EDGE('',*,*,#13926,.T.);
#19462=ORIENTED_EDGE('',*,*,#13931,.T.);
#19463=ORIENTED_EDGE('',*,*,#13932,.F.);
#19464=ORIENTED_EDGE('',*,*,#13933,.T.);
#19465=ORIENTED_EDGE('',*,*,#13929,.T.);
#19466=ORIENTED_EDGE('',*,*,#13934,.T.);
#19467=ORIENTED_EDGE('',*,*,#13935,.F.);
#19468=ORIENTED_EDGE('',*,*,#13936,.T.);
#19469=ORIENTED_EDGE('',*,*,#13932,.T.);
#19470=ORIENTED_EDGE('',*,*,#13937,.T.);
#19471=ORIENTED_EDGE('',*,*,#13938,.F.);
#19472=ORIENTED_EDGE('',*,*,#13939,.T.);
#19473=ORIENTED_EDGE('',*,*,#13935,.T.);
#19474=ORIENTED_EDGE('',*,*,#13940,.T.);
#19475=ORIENTED_EDGE('',*,*,#13941,.F.);
#19476=ORIENTED_EDGE('',*,*,#13942,.T.);
#19477=ORIENTED_EDGE('',*,*,#13938,.T.);
#19478=ORIENTED_EDGE('',*,*,#13943,.T.);
#19479=ORIENTED_EDGE('',*,*,#13944,.F.);
#19480=ORIENTED_EDGE('',*,*,#13945,.T.);
#19481=ORIENTED_EDGE('',*,*,#13941,.T.);
#19482=ORIENTED_EDGE('',*,*,#13946,.T.);
#19483=ORIENTED_EDGE('',*,*,#13947,.F.);
#19484=ORIENTED_EDGE('',*,*,#13948,.T.);
#19485=ORIENTED_EDGE('',*,*,#13944,.T.);
#19486=ORIENTED_EDGE('',*,*,#13949,.T.);
#19487=ORIENTED_EDGE('',*,*,#13950,.F.);
#19488=ORIENTED_EDGE('',*,*,#13951,.T.);
#19489=ORIENTED_EDGE('',*,*,#13947,.T.);
#19490=ORIENTED_EDGE('',*,*,#13952,.T.);
#19491=ORIENTED_EDGE('',*,*,#13953,.F.);
#19492=ORIENTED_EDGE('',*,*,#13954,.T.);
#19493=ORIENTED_EDGE('',*,*,#13950,.T.);
#19494=ORIENTED_EDGE('',*,*,#13955,.T.);
#19495=ORIENTED_EDGE('',*,*,#13956,.F.);
#19496=ORIENTED_EDGE('',*,*,#13957,.T.);
#19497=ORIENTED_EDGE('',*,*,#13953,.T.);
#19498=ORIENTED_EDGE('',*,*,#13958,.T.);
#19499=ORIENTED_EDGE('',*,*,#13959,.F.);
#19500=ORIENTED_EDGE('',*,*,#13960,.T.);
#19501=ORIENTED_EDGE('',*,*,#13956,.T.);
#19502=ORIENTED_EDGE('',*,*,#13961,.T.);
#19503=ORIENTED_EDGE('',*,*,#13962,.F.);
#19504=ORIENTED_EDGE('',*,*,#13963,.T.);
#19505=ORIENTED_EDGE('',*,*,#13959,.T.);
#19506=ORIENTED_EDGE('',*,*,#13964,.T.);
#19507=ORIENTED_EDGE('',*,*,#13965,.F.);
#19508=ORIENTED_EDGE('',*,*,#13966,.T.);
#19509=ORIENTED_EDGE('',*,*,#13962,.T.);
#19510=ORIENTED_EDGE('',*,*,#13967,.T.);
#19511=ORIENTED_EDGE('',*,*,#13968,.F.);
#19512=ORIENTED_EDGE('',*,*,#13969,.T.);
#19513=ORIENTED_EDGE('',*,*,#13965,.T.);
#19514=ORIENTED_EDGE('',*,*,#13970,.T.);
#19515=ORIENTED_EDGE('',*,*,#13971,.F.);
#19516=ORIENTED_EDGE('',*,*,#13972,.T.);
#19517=ORIENTED_EDGE('',*,*,#13968,.T.);
#19518=ORIENTED_EDGE('',*,*,#13973,.T.);
#19519=ORIENTED_EDGE('',*,*,#13974,.F.);
#19520=ORIENTED_EDGE('',*,*,#13975,.T.);
#19521=ORIENTED_EDGE('',*,*,#13971,.T.);
#19522=ORIENTED_EDGE('',*,*,#13976,.T.);
#19523=ORIENTED_EDGE('',*,*,#13977,.F.);
#19524=ORIENTED_EDGE('',*,*,#13978,.T.);
#19525=ORIENTED_EDGE('',*,*,#13974,.T.);
#19526=ORIENTED_EDGE('',*,*,#13979,.T.);
#19527=ORIENTED_EDGE('',*,*,#13980,.F.);
#19528=ORIENTED_EDGE('',*,*,#13981,.T.);
#19529=ORIENTED_EDGE('',*,*,#13977,.T.);
#19530=ORIENTED_EDGE('',*,*,#13982,.T.);
#19531=ORIENTED_EDGE('',*,*,#13983,.F.);
#19532=ORIENTED_EDGE('',*,*,#13984,.T.);
#19533=ORIENTED_EDGE('',*,*,#13980,.T.);
#19534=ORIENTED_EDGE('',*,*,#13985,.T.);
#19535=ORIENTED_EDGE('',*,*,#13986,.F.);
#19536=ORIENTED_EDGE('',*,*,#13987,.T.);
#19537=ORIENTED_EDGE('',*,*,#13983,.T.);
#19538=ORIENTED_EDGE('',*,*,#13988,.T.);
#19539=ORIENTED_EDGE('',*,*,#13989,.F.);
#19540=ORIENTED_EDGE('',*,*,#13990,.T.);
#19541=ORIENTED_EDGE('',*,*,#13986,.T.);
#19542=ORIENTED_EDGE('',*,*,#13991,.T.);
#19543=ORIENTED_EDGE('',*,*,#13992,.F.);
#19544=ORIENTED_EDGE('',*,*,#13993,.T.);
#19545=ORIENTED_EDGE('',*,*,#13989,.T.);
#19546=ORIENTED_EDGE('',*,*,#13994,.T.);
#19547=ORIENTED_EDGE('',*,*,#13995,.F.);
#19548=ORIENTED_EDGE('',*,*,#13996,.T.);
#19549=ORIENTED_EDGE('',*,*,#13992,.T.);
#19550=ORIENTED_EDGE('',*,*,#13997,.T.);
#19551=ORIENTED_EDGE('',*,*,#13998,.F.);
#19552=ORIENTED_EDGE('',*,*,#13999,.T.);
#19553=ORIENTED_EDGE('',*,*,#13995,.T.);
#19554=ORIENTED_EDGE('',*,*,#14000,.T.);
#19555=ORIENTED_EDGE('',*,*,#14001,.F.);
#19556=ORIENTED_EDGE('',*,*,#14002,.T.);
#19557=ORIENTED_EDGE('',*,*,#13998,.T.);
#19558=ORIENTED_EDGE('',*,*,#14003,.T.);
#19559=ORIENTED_EDGE('',*,*,#14004,.F.);
#19560=ORIENTED_EDGE('',*,*,#14005,.T.);
#19561=ORIENTED_EDGE('',*,*,#14001,.T.);
#19562=ORIENTED_EDGE('',*,*,#14006,.T.);
#19563=ORIENTED_EDGE('',*,*,#14007,.F.);
#19564=ORIENTED_EDGE('',*,*,#14008,.T.);
#19565=ORIENTED_EDGE('',*,*,#14004,.T.);
#19566=ORIENTED_EDGE('',*,*,#14009,.T.);
#19567=ORIENTED_EDGE('',*,*,#14010,.F.);
#19568=ORIENTED_EDGE('',*,*,#14011,.T.);
#19569=ORIENTED_EDGE('',*,*,#14007,.T.);
#19570=ORIENTED_EDGE('',*,*,#14012,.T.);
#19571=ORIENTED_EDGE('',*,*,#14013,.F.);
#19572=ORIENTED_EDGE('',*,*,#14014,.T.);
#19573=ORIENTED_EDGE('',*,*,#14010,.T.);
#19574=ORIENTED_EDGE('',*,*,#14015,.T.);
#19575=ORIENTED_EDGE('',*,*,#14016,.F.);
#19576=ORIENTED_EDGE('',*,*,#14017,.T.);
#19577=ORIENTED_EDGE('',*,*,#14013,.T.);
#19578=ORIENTED_EDGE('',*,*,#14018,.T.);
#19579=ORIENTED_EDGE('',*,*,#14019,.F.);
#19580=ORIENTED_EDGE('',*,*,#14020,.T.);
#19581=ORIENTED_EDGE('',*,*,#14016,.T.);
#19582=ORIENTED_EDGE('',*,*,#14021,.T.);
#19583=ORIENTED_EDGE('',*,*,#14022,.F.);
#19584=ORIENTED_EDGE('',*,*,#14023,.T.);
#19585=ORIENTED_EDGE('',*,*,#14019,.T.);
#19586=ORIENTED_EDGE('',*,*,#14024,.T.);
#19587=ORIENTED_EDGE('',*,*,#14025,.F.);
#19588=ORIENTED_EDGE('',*,*,#14026,.T.);
#19589=ORIENTED_EDGE('',*,*,#14022,.T.);
#19590=ORIENTED_EDGE('',*,*,#14027,.T.);
#19591=ORIENTED_EDGE('',*,*,#14028,.F.);
#19592=ORIENTED_EDGE('',*,*,#14029,.T.);
#19593=ORIENTED_EDGE('',*,*,#14025,.T.);
#19594=ORIENTED_EDGE('',*,*,#14030,.T.);
#19595=ORIENTED_EDGE('',*,*,#14031,.F.);
#19596=ORIENTED_EDGE('',*,*,#14032,.T.);
#19597=ORIENTED_EDGE('',*,*,#14028,.T.);
#19598=ORIENTED_EDGE('',*,*,#14033,.T.);
#19599=ORIENTED_EDGE('',*,*,#14034,.F.);
#19600=ORIENTED_EDGE('',*,*,#14035,.T.);
#19601=ORIENTED_EDGE('',*,*,#14031,.T.);
#19602=ORIENTED_EDGE('',*,*,#14036,.T.);
#19603=ORIENTED_EDGE('',*,*,#14037,.F.);
#19604=ORIENTED_EDGE('',*,*,#14038,.T.);
#19605=ORIENTED_EDGE('',*,*,#14034,.T.);
#19606=ORIENTED_EDGE('',*,*,#14039,.T.);
#19607=ORIENTED_EDGE('',*,*,#14040,.F.);
#19608=ORIENTED_EDGE('',*,*,#14041,.T.);
#19609=ORIENTED_EDGE('',*,*,#14037,.T.);
#19610=ORIENTED_EDGE('',*,*,#14042,.T.);
#19611=ORIENTED_EDGE('',*,*,#14043,.F.);
#19612=ORIENTED_EDGE('',*,*,#14044,.T.);
#19613=ORIENTED_EDGE('',*,*,#14045,.F.);
#19614=ORIENTED_EDGE('',*,*,#14046,.F.);
#19615=ORIENTED_EDGE('',*,*,#14047,.F.);
#19616=ORIENTED_EDGE('',*,*,#14048,.T.);
#19617=ORIENTED_EDGE('',*,*,#14043,.T.);
#19618=ORIENTED_EDGE('',*,*,#14049,.F.);
#19619=ORIENTED_EDGE('',*,*,#14050,.F.);
#19620=ORIENTED_EDGE('',*,*,#14051,.T.);
#19621=ORIENTED_EDGE('',*,*,#14047,.T.);
#19622=ORIENTED_EDGE('',*,*,#14052,.F.);
#19623=ORIENTED_EDGE('',*,*,#14053,.F.);
#19624=ORIENTED_EDGE('',*,*,#14054,.T.);
#19625=ORIENTED_EDGE('',*,*,#14050,.T.);
#19626=ORIENTED_EDGE('',*,*,#14055,.F.);
#19627=ORIENTED_EDGE('',*,*,#14056,.F.);
#19628=ORIENTED_EDGE('',*,*,#14057,.T.);
#19629=ORIENTED_EDGE('',*,*,#14053,.T.);
#19630=ORIENTED_EDGE('',*,*,#14058,.F.);
#19631=ORIENTED_EDGE('',*,*,#14059,.F.);
#19632=ORIENTED_EDGE('',*,*,#14060,.T.);
#19633=ORIENTED_EDGE('',*,*,#14056,.T.);
#19634=ORIENTED_EDGE('',*,*,#14061,.F.);
#19635=ORIENTED_EDGE('',*,*,#14062,.F.);
#19636=ORIENTED_EDGE('',*,*,#14063,.T.);
#19637=ORIENTED_EDGE('',*,*,#14059,.T.);
#19638=ORIENTED_EDGE('',*,*,#14064,.F.);
#19639=ORIENTED_EDGE('',*,*,#14065,.F.);
#19640=ORIENTED_EDGE('',*,*,#14066,.T.);
#19641=ORIENTED_EDGE('',*,*,#14062,.T.);
#19642=ORIENTED_EDGE('',*,*,#14067,.F.);
#19643=ORIENTED_EDGE('',*,*,#14068,.F.);
#19644=ORIENTED_EDGE('',*,*,#14069,.T.);
#19645=ORIENTED_EDGE('',*,*,#14065,.T.);
#19646=ORIENTED_EDGE('',*,*,#14070,.F.);
#19647=ORIENTED_EDGE('',*,*,#14071,.F.);
#19648=ORIENTED_EDGE('',*,*,#14072,.T.);
#19649=ORIENTED_EDGE('',*,*,#14068,.T.);
#19650=ORIENTED_EDGE('',*,*,#14073,.F.);
#19651=ORIENTED_EDGE('',*,*,#14074,.F.);
#19652=ORIENTED_EDGE('',*,*,#14075,.T.);
#19653=ORIENTED_EDGE('',*,*,#14071,.T.);
#19654=ORIENTED_EDGE('',*,*,#14076,.F.);
#19655=ORIENTED_EDGE('',*,*,#14077,.F.);
#19656=ORIENTED_EDGE('',*,*,#14078,.T.);
#19657=ORIENTED_EDGE('',*,*,#14074,.T.);
#19658=ORIENTED_EDGE('',*,*,#14079,.F.);
#19659=ORIENTED_EDGE('',*,*,#14080,.F.);
#19660=ORIENTED_EDGE('',*,*,#14081,.T.);
#19661=ORIENTED_EDGE('',*,*,#14077,.T.);
#19662=ORIENTED_EDGE('',*,*,#14082,.F.);
#19663=ORIENTED_EDGE('',*,*,#14083,.F.);
#19664=ORIENTED_EDGE('',*,*,#14084,.T.);
#19665=ORIENTED_EDGE('',*,*,#14080,.T.);
#19666=ORIENTED_EDGE('',*,*,#14085,.F.);
#19667=ORIENTED_EDGE('',*,*,#14086,.F.);
#19668=ORIENTED_EDGE('',*,*,#14087,.T.);
#19669=ORIENTED_EDGE('',*,*,#14083,.T.);
#19670=ORIENTED_EDGE('',*,*,#14088,.F.);
#19671=ORIENTED_EDGE('',*,*,#14089,.F.);
#19672=ORIENTED_EDGE('',*,*,#14090,.T.);
#19673=ORIENTED_EDGE('',*,*,#14086,.T.);
#19674=ORIENTED_EDGE('',*,*,#14091,.F.);
#19675=ORIENTED_EDGE('',*,*,#14092,.F.);
#19676=ORIENTED_EDGE('',*,*,#14093,.T.);
#19677=ORIENTED_EDGE('',*,*,#14089,.T.);
#19678=ORIENTED_EDGE('',*,*,#14094,.F.);
#19679=ORIENTED_EDGE('',*,*,#14095,.F.);
#19680=ORIENTED_EDGE('',*,*,#14096,.T.);
#19681=ORIENTED_EDGE('',*,*,#14092,.T.);
#19682=ORIENTED_EDGE('',*,*,#14097,.F.);
#19683=ORIENTED_EDGE('',*,*,#14098,.F.);
#19684=ORIENTED_EDGE('',*,*,#14099,.T.);
#19685=ORIENTED_EDGE('',*,*,#14095,.T.);
#19686=ORIENTED_EDGE('',*,*,#14100,.F.);
#19687=ORIENTED_EDGE('',*,*,#14101,.F.);
#19688=ORIENTED_EDGE('',*,*,#14102,.T.);
#19689=ORIENTED_EDGE('',*,*,#14098,.T.);
#19690=ORIENTED_EDGE('',*,*,#14103,.F.);
#19691=ORIENTED_EDGE('',*,*,#14104,.F.);
#19692=ORIENTED_EDGE('',*,*,#14105,.T.);
#19693=ORIENTED_EDGE('',*,*,#14101,.T.);
#19694=ORIENTED_EDGE('',*,*,#14106,.F.);
#19695=ORIENTED_EDGE('',*,*,#14107,.F.);
#19696=ORIENTED_EDGE('',*,*,#14108,.T.);
#19697=ORIENTED_EDGE('',*,*,#14104,.T.);
#19698=ORIENTED_EDGE('',*,*,#14109,.F.);
#19699=ORIENTED_EDGE('',*,*,#14110,.F.);
#19700=ORIENTED_EDGE('',*,*,#14111,.T.);
#19701=ORIENTED_EDGE('',*,*,#14107,.T.);
#19702=ORIENTED_EDGE('',*,*,#14112,.F.);
#19703=ORIENTED_EDGE('',*,*,#14113,.F.);
#19704=ORIENTED_EDGE('',*,*,#14114,.T.);
#19705=ORIENTED_EDGE('',*,*,#14110,.T.);
#19706=ORIENTED_EDGE('',*,*,#14115,.F.);
#19707=ORIENTED_EDGE('',*,*,#14116,.F.);
#19708=ORIENTED_EDGE('',*,*,#14117,.T.);
#19709=ORIENTED_EDGE('',*,*,#14113,.T.);
#19710=ORIENTED_EDGE('',*,*,#14118,.F.);
#19711=ORIENTED_EDGE('',*,*,#14119,.F.);
#19712=ORIENTED_EDGE('',*,*,#14120,.T.);
#19713=ORIENTED_EDGE('',*,*,#14116,.T.);
#19714=ORIENTED_EDGE('',*,*,#14121,.F.);
#19715=ORIENTED_EDGE('',*,*,#14122,.F.);
#19716=ORIENTED_EDGE('',*,*,#14123,.T.);
#19717=ORIENTED_EDGE('',*,*,#14119,.T.);
#19718=ORIENTED_EDGE('',*,*,#14124,.F.);
#19719=ORIENTED_EDGE('',*,*,#14125,.F.);
#19720=ORIENTED_EDGE('',*,*,#14126,.T.);
#19721=ORIENTED_EDGE('',*,*,#14122,.T.);
#19722=ORIENTED_EDGE('',*,*,#14127,.F.);
#19723=ORIENTED_EDGE('',*,*,#14128,.F.);
#19724=ORIENTED_EDGE('',*,*,#14129,.T.);
#19725=ORIENTED_EDGE('',*,*,#14125,.T.);
#19726=ORIENTED_EDGE('',*,*,#14130,.F.);
#19727=ORIENTED_EDGE('',*,*,#14131,.F.);
#19728=ORIENTED_EDGE('',*,*,#14132,.T.);
#19729=ORIENTED_EDGE('',*,*,#14128,.T.);
#19730=ORIENTED_EDGE('',*,*,#14133,.F.);
#19731=ORIENTED_EDGE('',*,*,#14134,.F.);
#19732=ORIENTED_EDGE('',*,*,#14135,.T.);
#19733=ORIENTED_EDGE('',*,*,#14131,.T.);
#19734=ORIENTED_EDGE('',*,*,#14136,.F.);
#19735=ORIENTED_EDGE('',*,*,#14137,.F.);
#19736=ORIENTED_EDGE('',*,*,#14138,.T.);
#19737=ORIENTED_EDGE('',*,*,#14134,.T.);
#19738=ORIENTED_EDGE('',*,*,#14139,.F.);
#19739=ORIENTED_EDGE('',*,*,#14140,.F.);
#19740=ORIENTED_EDGE('',*,*,#14141,.T.);
#19741=ORIENTED_EDGE('',*,*,#14137,.T.);
#19742=ORIENTED_EDGE('',*,*,#14142,.F.);
#19743=ORIENTED_EDGE('',*,*,#14143,.F.);
#19744=ORIENTED_EDGE('',*,*,#14144,.T.);
#19745=ORIENTED_EDGE('',*,*,#14140,.T.);
#19746=ORIENTED_EDGE('',*,*,#14145,.F.);
#19747=ORIENTED_EDGE('',*,*,#14146,.F.);
#19748=ORIENTED_EDGE('',*,*,#14147,.T.);
#19749=ORIENTED_EDGE('',*,*,#14143,.T.);
#19750=ORIENTED_EDGE('',*,*,#14148,.F.);
#19751=ORIENTED_EDGE('',*,*,#14149,.F.);
#19752=ORIENTED_EDGE('',*,*,#14150,.T.);
#19753=ORIENTED_EDGE('',*,*,#14146,.T.);
#19754=ORIENTED_EDGE('',*,*,#14151,.F.);
#19755=ORIENTED_EDGE('',*,*,#14152,.F.);
#19756=ORIENTED_EDGE('',*,*,#14153,.T.);
#19757=ORIENTED_EDGE('',*,*,#14149,.T.);
#19758=ORIENTED_EDGE('',*,*,#14154,.F.);
#19759=ORIENTED_EDGE('',*,*,#14155,.F.);
#19760=ORIENTED_EDGE('',*,*,#14156,.T.);
#19761=ORIENTED_EDGE('',*,*,#14152,.T.);
#19762=ORIENTED_EDGE('',*,*,#14157,.F.);
#19763=ORIENTED_EDGE('',*,*,#14158,.F.);
#19764=ORIENTED_EDGE('',*,*,#14159,.T.);
#19765=ORIENTED_EDGE('',*,*,#14155,.T.);
#19766=ORIENTED_EDGE('',*,*,#14160,.F.);
#19767=ORIENTED_EDGE('',*,*,#14161,.F.);
#19768=ORIENTED_EDGE('',*,*,#14162,.T.);
#19769=ORIENTED_EDGE('',*,*,#14158,.T.);
#19770=ORIENTED_EDGE('',*,*,#14163,.F.);
#19771=ORIENTED_EDGE('',*,*,#14164,.F.);
#19772=ORIENTED_EDGE('',*,*,#14165,.T.);
#19773=ORIENTED_EDGE('',*,*,#14161,.T.);
#19774=ORIENTED_EDGE('',*,*,#14166,.F.);
#19775=ORIENTED_EDGE('',*,*,#14167,.F.);
#19776=ORIENTED_EDGE('',*,*,#14168,.T.);
#19777=ORIENTED_EDGE('',*,*,#14164,.T.);
#19778=ORIENTED_EDGE('',*,*,#14169,.F.);
#19779=ORIENTED_EDGE('',*,*,#14170,.F.);
#19780=ORIENTED_EDGE('',*,*,#14171,.T.);
#19781=ORIENTED_EDGE('',*,*,#14167,.T.);
#19782=ORIENTED_EDGE('',*,*,#14172,.F.);
#19783=ORIENTED_EDGE('',*,*,#14173,.F.);
#19784=ORIENTED_EDGE('',*,*,#14174,.T.);
#19785=ORIENTED_EDGE('',*,*,#14170,.T.);
#19786=ORIENTED_EDGE('',*,*,#14175,.F.);
#19787=ORIENTED_EDGE('',*,*,#14176,.F.);
#19788=ORIENTED_EDGE('',*,*,#14177,.T.);
#19789=ORIENTED_EDGE('',*,*,#14173,.T.);
#19790=ORIENTED_EDGE('',*,*,#14178,.F.);
#19791=ORIENTED_EDGE('',*,*,#14179,.F.);
#19792=ORIENTED_EDGE('',*,*,#14180,.T.);
#19793=ORIENTED_EDGE('',*,*,#14176,.T.);
#19794=ORIENTED_EDGE('',*,*,#14181,.F.);
#19795=ORIENTED_EDGE('',*,*,#14182,.F.);
#19796=ORIENTED_EDGE('',*,*,#14183,.T.);
#19797=ORIENTED_EDGE('',*,*,#14179,.T.);
#19798=ORIENTED_EDGE('',*,*,#14184,.F.);
#19799=ORIENTED_EDGE('',*,*,#14185,.F.);
#19800=ORIENTED_EDGE('',*,*,#14186,.T.);
#19801=ORIENTED_EDGE('',*,*,#14182,.T.);
#19802=ORIENTED_EDGE('',*,*,#14187,.F.);
#19803=ORIENTED_EDGE('',*,*,#14188,.F.);
#19804=ORIENTED_EDGE('',*,*,#14189,.T.);
#19805=ORIENTED_EDGE('',*,*,#14185,.T.);
#19806=ORIENTED_EDGE('',*,*,#14190,.F.);
#19807=ORIENTED_EDGE('',*,*,#14191,.F.);
#19808=ORIENTED_EDGE('',*,*,#14192,.T.);
#19809=ORIENTED_EDGE('',*,*,#14188,.T.);
#19810=ORIENTED_EDGE('',*,*,#14193,.F.);
#19811=ORIENTED_EDGE('',*,*,#14194,.F.);
#19812=ORIENTED_EDGE('',*,*,#14195,.T.);
#19813=ORIENTED_EDGE('',*,*,#14191,.T.);
#19814=ORIENTED_EDGE('',*,*,#14196,.F.);
#19815=ORIENTED_EDGE('',*,*,#14197,.F.);
#19816=ORIENTED_EDGE('',*,*,#14198,.T.);
#19817=ORIENTED_EDGE('',*,*,#14194,.T.);
#19818=ORIENTED_EDGE('',*,*,#14199,.F.);
#19819=ORIENTED_EDGE('',*,*,#14200,.F.);
#19820=ORIENTED_EDGE('',*,*,#14201,.T.);
#19821=ORIENTED_EDGE('',*,*,#14197,.T.);
#19822=ORIENTED_EDGE('',*,*,#14202,.F.);
#19823=ORIENTED_EDGE('',*,*,#14203,.F.);
#19824=ORIENTED_EDGE('',*,*,#14204,.T.);
#19825=ORIENTED_EDGE('',*,*,#14200,.T.);
#19826=ORIENTED_EDGE('',*,*,#14205,.F.);
#19827=ORIENTED_EDGE('',*,*,#14206,.F.);
#19828=ORIENTED_EDGE('',*,*,#14207,.T.);
#19829=ORIENTED_EDGE('',*,*,#14203,.T.);
#19830=ORIENTED_EDGE('',*,*,#14208,.F.);
#19831=ORIENTED_EDGE('',*,*,#14209,.F.);
#19832=ORIENTED_EDGE('',*,*,#14210,.T.);
#19833=ORIENTED_EDGE('',*,*,#14206,.T.);
#19834=ORIENTED_EDGE('',*,*,#14211,.F.);
#19835=ORIENTED_EDGE('',*,*,#14212,.F.);
#19836=ORIENTED_EDGE('',*,*,#14213,.T.);
#19837=ORIENTED_EDGE('',*,*,#14209,.T.);
#19838=ORIENTED_EDGE('',*,*,#14214,.F.);
#19839=ORIENTED_EDGE('',*,*,#14215,.F.);
#19840=ORIENTED_EDGE('',*,*,#14216,.T.);
#19841=ORIENTED_EDGE('',*,*,#14212,.T.);
#19842=ORIENTED_EDGE('',*,*,#14217,.F.);
#19843=ORIENTED_EDGE('',*,*,#14218,.F.);
#19844=ORIENTED_EDGE('',*,*,#14219,.T.);
#19845=ORIENTED_EDGE('',*,*,#14215,.T.);
#19846=ORIENTED_EDGE('',*,*,#14220,.F.);
#19847=ORIENTED_EDGE('',*,*,#14045,.T.);
#19848=ORIENTED_EDGE('',*,*,#14221,.T.);
#19849=ORIENTED_EDGE('',*,*,#14222,.F.);
#19850=ORIENTED_EDGE('',*,*,#14223,.F.);
#19851=ORIENTED_EDGE('',*,*,#14224,.T.);
#19852=ORIENTED_EDGE('',*,*,#14224,.F.);
#19853=ORIENTED_EDGE('',*,*,#14225,.F.);
#19854=ORIENTED_EDGE('',*,*,#14042,.F.);
#19855=ORIENTED_EDGE('',*,*,#14039,.F.);
#19856=ORIENTED_EDGE('',*,*,#14036,.F.);
#19857=ORIENTED_EDGE('',*,*,#14033,.F.);
#19858=ORIENTED_EDGE('',*,*,#14030,.F.);
#19859=ORIENTED_EDGE('',*,*,#14027,.F.);
#19860=ORIENTED_EDGE('',*,*,#14024,.F.);
#19861=ORIENTED_EDGE('',*,*,#14021,.F.);
#19862=ORIENTED_EDGE('',*,*,#14018,.F.);
#19863=ORIENTED_EDGE('',*,*,#14015,.F.);
#19864=ORIENTED_EDGE('',*,*,#14012,.F.);
#19865=ORIENTED_EDGE('',*,*,#14009,.F.);
#19866=ORIENTED_EDGE('',*,*,#14006,.F.);
#19867=ORIENTED_EDGE('',*,*,#14003,.F.);
#19868=ORIENTED_EDGE('',*,*,#14000,.F.);
#19869=ORIENTED_EDGE('',*,*,#13997,.F.);
#19870=ORIENTED_EDGE('',*,*,#13994,.F.);
#19871=ORIENTED_EDGE('',*,*,#13991,.F.);
#19872=ORIENTED_EDGE('',*,*,#13988,.F.);
#19873=ORIENTED_EDGE('',*,*,#13985,.F.);
#19874=ORIENTED_EDGE('',*,*,#13982,.F.);
#19875=ORIENTED_EDGE('',*,*,#13979,.F.);
#19876=ORIENTED_EDGE('',*,*,#13976,.F.);
#19877=ORIENTED_EDGE('',*,*,#13973,.F.);
#19878=ORIENTED_EDGE('',*,*,#13970,.F.);
#19879=ORIENTED_EDGE('',*,*,#13967,.F.);
#19880=ORIENTED_EDGE('',*,*,#13964,.F.);
#19881=ORIENTED_EDGE('',*,*,#13961,.F.);
#19882=ORIENTED_EDGE('',*,*,#13958,.F.);
#19883=ORIENTED_EDGE('',*,*,#13955,.F.);
#19884=ORIENTED_EDGE('',*,*,#13952,.F.);
#19885=ORIENTED_EDGE('',*,*,#13949,.F.);
#19886=ORIENTED_EDGE('',*,*,#13946,.F.);
#19887=ORIENTED_EDGE('',*,*,#13943,.F.);
#19888=ORIENTED_EDGE('',*,*,#13940,.F.);
#19889=ORIENTED_EDGE('',*,*,#13937,.F.);
#19890=ORIENTED_EDGE('',*,*,#13934,.F.);
#19891=ORIENTED_EDGE('',*,*,#13931,.F.);
#19892=ORIENTED_EDGE('',*,*,#13928,.F.);
#19893=ORIENTED_EDGE('',*,*,#13925,.F.);
#19894=ORIENTED_EDGE('',*,*,#13922,.F.);
#19895=ORIENTED_EDGE('',*,*,#13919,.F.);
#19896=ORIENTED_EDGE('',*,*,#13916,.F.);
#19897=ORIENTED_EDGE('',*,*,#13913,.F.);
#19898=ORIENTED_EDGE('',*,*,#13910,.F.);
#19899=ORIENTED_EDGE('',*,*,#13907,.F.);
#19900=ORIENTED_EDGE('',*,*,#13904,.F.);
#19901=ORIENTED_EDGE('',*,*,#13901,.F.);
#19902=ORIENTED_EDGE('',*,*,#13898,.F.);
#19903=ORIENTED_EDGE('',*,*,#13895,.F.);
#19904=ORIENTED_EDGE('',*,*,#13892,.F.);
#19905=ORIENTED_EDGE('',*,*,#13889,.F.);
#19906=ORIENTED_EDGE('',*,*,#13886,.F.);
#19907=ORIENTED_EDGE('',*,*,#13883,.F.);
#19908=ORIENTED_EDGE('',*,*,#13880,.F.);
#19909=ORIENTED_EDGE('',*,*,#13877,.F.);
#19910=ORIENTED_EDGE('',*,*,#13874,.F.);
#19911=ORIENTED_EDGE('',*,*,#13871,.F.);
#19912=ORIENTED_EDGE('',*,*,#14226,.F.);
#19913=ORIENTED_EDGE('',*,*,#14227,.T.);
#19914=ORIENTED_EDGE('',*,*,#14220,.T.);
#19915=ORIENTED_EDGE('',*,*,#14217,.T.);
#19916=ORIENTED_EDGE('',*,*,#14214,.T.);
#19917=ORIENTED_EDGE('',*,*,#14211,.T.);
#19918=ORIENTED_EDGE('',*,*,#14208,.T.);
#19919=ORIENTED_EDGE('',*,*,#14205,.T.);
#19920=ORIENTED_EDGE('',*,*,#14202,.T.);
#19921=ORIENTED_EDGE('',*,*,#14199,.T.);
#19922=ORIENTED_EDGE('',*,*,#14196,.T.);
#19923=ORIENTED_EDGE('',*,*,#14193,.T.);
#19924=ORIENTED_EDGE('',*,*,#14190,.T.);
#19925=ORIENTED_EDGE('',*,*,#14187,.T.);
#19926=ORIENTED_EDGE('',*,*,#14184,.T.);
#19927=ORIENTED_EDGE('',*,*,#14181,.T.);
#19928=ORIENTED_EDGE('',*,*,#14178,.T.);
#19929=ORIENTED_EDGE('',*,*,#14175,.T.);
#19930=ORIENTED_EDGE('',*,*,#14172,.T.);
#19931=ORIENTED_EDGE('',*,*,#14169,.T.);
#19932=ORIENTED_EDGE('',*,*,#14166,.T.);
#19933=ORIENTED_EDGE('',*,*,#14163,.T.);
#19934=ORIENTED_EDGE('',*,*,#14160,.T.);
#19935=ORIENTED_EDGE('',*,*,#14157,.T.);
#19936=ORIENTED_EDGE('',*,*,#14154,.T.);
#19937=ORIENTED_EDGE('',*,*,#14151,.T.);
#19938=ORIENTED_EDGE('',*,*,#14148,.T.);
#19939=ORIENTED_EDGE('',*,*,#14145,.T.);
#19940=ORIENTED_EDGE('',*,*,#14142,.T.);
#19941=ORIENTED_EDGE('',*,*,#14139,.T.);
#19942=ORIENTED_EDGE('',*,*,#14136,.T.);
#19943=ORIENTED_EDGE('',*,*,#14133,.T.);
#19944=ORIENTED_EDGE('',*,*,#14130,.T.);
#19945=ORIENTED_EDGE('',*,*,#14127,.T.);
#19946=ORIENTED_EDGE('',*,*,#14124,.T.);
#19947=ORIENTED_EDGE('',*,*,#14121,.T.);
#19948=ORIENTED_EDGE('',*,*,#14118,.T.);
#19949=ORIENTED_EDGE('',*,*,#14115,.T.);
#19950=ORIENTED_EDGE('',*,*,#14112,.T.);
#19951=ORIENTED_EDGE('',*,*,#14109,.T.);
#19952=ORIENTED_EDGE('',*,*,#14106,.T.);
#19953=ORIENTED_EDGE('',*,*,#14103,.T.);
#19954=ORIENTED_EDGE('',*,*,#14100,.T.);
#19955=ORIENTED_EDGE('',*,*,#14097,.T.);
#19956=ORIENTED_EDGE('',*,*,#14094,.T.);
#19957=ORIENTED_EDGE('',*,*,#14091,.T.);
#19958=ORIENTED_EDGE('',*,*,#14088,.T.);
#19959=ORIENTED_EDGE('',*,*,#14085,.T.);
#19960=ORIENTED_EDGE('',*,*,#14082,.T.);
#19961=ORIENTED_EDGE('',*,*,#14079,.T.);
#19962=ORIENTED_EDGE('',*,*,#14076,.T.);
#19963=ORIENTED_EDGE('',*,*,#14073,.T.);
#19964=ORIENTED_EDGE('',*,*,#14070,.T.);
#19965=ORIENTED_EDGE('',*,*,#14067,.T.);
#19966=ORIENTED_EDGE('',*,*,#14064,.T.);
#19967=ORIENTED_EDGE('',*,*,#14061,.T.);
#19968=ORIENTED_EDGE('',*,*,#14058,.T.);
#19969=ORIENTED_EDGE('',*,*,#14055,.T.);
#19970=ORIENTED_EDGE('',*,*,#14052,.T.);
#19971=ORIENTED_EDGE('',*,*,#14049,.T.);
#19972=ORIENTED_EDGE('',*,*,#14046,.T.);
#19973=ORIENTED_EDGE('',*,*,#13867,.F.);
#19974=ORIENTED_EDGE('',*,*,#14228,.T.);
#19975=ORIENTED_EDGE('',*,*,#14229,.T.);
#19976=ORIENTED_EDGE('',*,*,#14226,.T.);
#19977=ORIENTED_EDGE('',*,*,#13870,.F.);
#19978=ORIENTED_EDGE('',*,*,#14218,.T.);
#19979=ORIENTED_EDGE('',*,*,#14227,.F.);
#19980=ORIENTED_EDGE('',*,*,#14229,.F.);
#19981=ORIENTED_EDGE('',*,*,#14230,.T.);
#19982=ORIENTED_EDGE('',*,*,#14221,.F.);
#19983=ORIENTED_EDGE('',*,*,#14044,.F.);
#19984=ORIENTED_EDGE('',*,*,#14048,.F.);
#19985=ORIENTED_EDGE('',*,*,#14051,.F.);
#19986=ORIENTED_EDGE('',*,*,#14054,.F.);
#19987=ORIENTED_EDGE('',*,*,#14057,.F.);
#19988=ORIENTED_EDGE('',*,*,#14060,.F.);
#19989=ORIENTED_EDGE('',*,*,#14063,.F.);
#19990=ORIENTED_EDGE('',*,*,#14066,.F.);
#19991=ORIENTED_EDGE('',*,*,#14069,.F.);
#19992=ORIENTED_EDGE('',*,*,#14072,.F.);
#19993=ORIENTED_EDGE('',*,*,#14075,.F.);
#19994=ORIENTED_EDGE('',*,*,#14078,.F.);
#19995=ORIENTED_EDGE('',*,*,#14081,.F.);
#19996=ORIENTED_EDGE('',*,*,#14084,.F.);
#19997=ORIENTED_EDGE('',*,*,#14087,.F.);
#19998=ORIENTED_EDGE('',*,*,#14090,.F.);
#19999=ORIENTED_EDGE('',*,*,#14093,.F.);
#20000=ORIENTED_EDGE('',*,*,#14096,.F.);
#20001=ORIENTED_EDGE('',*,*,#14099,.F.);
#20002=ORIENTED_EDGE('',*,*,#14102,.F.);
#20003=ORIENTED_EDGE('',*,*,#14105,.F.);
#20004=ORIENTED_EDGE('',*,*,#14108,.F.);
#20005=ORIENTED_EDGE('',*,*,#14111,.F.);
#20006=ORIENTED_EDGE('',*,*,#14114,.F.);
#20007=ORIENTED_EDGE('',*,*,#14117,.F.);
#20008=ORIENTED_EDGE('',*,*,#14120,.F.);
#20009=ORIENTED_EDGE('',*,*,#14123,.F.);
#20010=ORIENTED_EDGE('',*,*,#14126,.F.);
#20011=ORIENTED_EDGE('',*,*,#14129,.F.);
#20012=ORIENTED_EDGE('',*,*,#14132,.F.);
#20013=ORIENTED_EDGE('',*,*,#14135,.F.);
#20014=ORIENTED_EDGE('',*,*,#14138,.F.);
#20015=ORIENTED_EDGE('',*,*,#14141,.F.);
#20016=ORIENTED_EDGE('',*,*,#14144,.F.);
#20017=ORIENTED_EDGE('',*,*,#14147,.F.);
#20018=ORIENTED_EDGE('',*,*,#14150,.F.);
#20019=ORIENTED_EDGE('',*,*,#14153,.F.);
#20020=ORIENTED_EDGE('',*,*,#14156,.F.);
#20021=ORIENTED_EDGE('',*,*,#14159,.F.);
#20022=ORIENTED_EDGE('',*,*,#14162,.F.);
#20023=ORIENTED_EDGE('',*,*,#14165,.F.);
#20024=ORIENTED_EDGE('',*,*,#14168,.F.);
#20025=ORIENTED_EDGE('',*,*,#14171,.F.);
#20026=ORIENTED_EDGE('',*,*,#14174,.F.);
#20027=ORIENTED_EDGE('',*,*,#14177,.F.);
#20028=ORIENTED_EDGE('',*,*,#14180,.F.);
#20029=ORIENTED_EDGE('',*,*,#14183,.F.);
#20030=ORIENTED_EDGE('',*,*,#14186,.F.);
#20031=ORIENTED_EDGE('',*,*,#14189,.F.);
#20032=ORIENTED_EDGE('',*,*,#14192,.F.);
#20033=ORIENTED_EDGE('',*,*,#14195,.F.);
#20034=ORIENTED_EDGE('',*,*,#14198,.F.);
#20035=ORIENTED_EDGE('',*,*,#14201,.F.);
#20036=ORIENTED_EDGE('',*,*,#14204,.F.);
#20037=ORIENTED_EDGE('',*,*,#14207,.F.);
#20038=ORIENTED_EDGE('',*,*,#14210,.F.);
#20039=ORIENTED_EDGE('',*,*,#14213,.F.);
#20040=ORIENTED_EDGE('',*,*,#14216,.F.);
#20041=ORIENTED_EDGE('',*,*,#14219,.F.);
#20042=ORIENTED_EDGE('',*,*,#14230,.F.);
#20043=ORIENTED_EDGE('',*,*,#14228,.F.);
#20044=ORIENTED_EDGE('',*,*,#13866,.F.);
#20045=ORIENTED_EDGE('',*,*,#13873,.F.);
#20046=ORIENTED_EDGE('',*,*,#13876,.F.);
#20047=ORIENTED_EDGE('',*,*,#13879,.F.);
#20048=ORIENTED_EDGE('',*,*,#13882,.F.);
#20049=ORIENTED_EDGE('',*,*,#13885,.F.);
#20050=ORIENTED_EDGE('',*,*,#13888,.F.);
#20051=ORIENTED_EDGE('',*,*,#13891,.F.);
#20052=ORIENTED_EDGE('',*,*,#13894,.F.);
#20053=ORIENTED_EDGE('',*,*,#13897,.F.);
#20054=ORIENTED_EDGE('',*,*,#13900,.F.);
#20055=ORIENTED_EDGE('',*,*,#13903,.F.);
#20056=ORIENTED_EDGE('',*,*,#13906,.F.);
#20057=ORIENTED_EDGE('',*,*,#13909,.F.);
#20058=ORIENTED_EDGE('',*,*,#13912,.F.);
#20059=ORIENTED_EDGE('',*,*,#13915,.F.);
#20060=ORIENTED_EDGE('',*,*,#13918,.F.);
#20061=ORIENTED_EDGE('',*,*,#13921,.F.);
#20062=ORIENTED_EDGE('',*,*,#13924,.F.);
#20063=ORIENTED_EDGE('',*,*,#13927,.F.);
#20064=ORIENTED_EDGE('',*,*,#13930,.F.);
#20065=ORIENTED_EDGE('',*,*,#13933,.F.);
#20066=ORIENTED_EDGE('',*,*,#13936,.F.);
#20067=ORIENTED_EDGE('',*,*,#13939,.F.);
#20068=ORIENTED_EDGE('',*,*,#13942,.F.);
#20069=ORIENTED_EDGE('',*,*,#13945,.F.);
#20070=ORIENTED_EDGE('',*,*,#13948,.F.);
#20071=ORIENTED_EDGE('',*,*,#13951,.F.);
#20072=ORIENTED_EDGE('',*,*,#13954,.F.);
#20073=ORIENTED_EDGE('',*,*,#13957,.F.);
#20074=ORIENTED_EDGE('',*,*,#13960,.F.);
#20075=ORIENTED_EDGE('',*,*,#13963,.F.);
#20076=ORIENTED_EDGE('',*,*,#13966,.F.);
#20077=ORIENTED_EDGE('',*,*,#13969,.F.);
#20078=ORIENTED_EDGE('',*,*,#13972,.F.);
#20079=ORIENTED_EDGE('',*,*,#13975,.F.);
#20080=ORIENTED_EDGE('',*,*,#13978,.F.);
#20081=ORIENTED_EDGE('',*,*,#13981,.F.);
#20082=ORIENTED_EDGE('',*,*,#13984,.F.);
#20083=ORIENTED_EDGE('',*,*,#13987,.F.);
#20084=ORIENTED_EDGE('',*,*,#13990,.F.);
#20085=ORIENTED_EDGE('',*,*,#13993,.F.);
#20086=ORIENTED_EDGE('',*,*,#13996,.F.);
#20087=ORIENTED_EDGE('',*,*,#13999,.F.);
#20088=ORIENTED_EDGE('',*,*,#14002,.F.);
#20089=ORIENTED_EDGE('',*,*,#14005,.F.);
#20090=ORIENTED_EDGE('',*,*,#14008,.F.);
#20091=ORIENTED_EDGE('',*,*,#14011,.F.);
#20092=ORIENTED_EDGE('',*,*,#14014,.F.);
#20093=ORIENTED_EDGE('',*,*,#14017,.F.);
#20094=ORIENTED_EDGE('',*,*,#14020,.F.);
#20095=ORIENTED_EDGE('',*,*,#14023,.F.);
#20096=ORIENTED_EDGE('',*,*,#14026,.F.);
#20097=ORIENTED_EDGE('',*,*,#14029,.F.);
#20098=ORIENTED_EDGE('',*,*,#14032,.F.);
#20099=ORIENTED_EDGE('',*,*,#14035,.F.);
#20100=ORIENTED_EDGE('',*,*,#14038,.F.);
#20101=ORIENTED_EDGE('',*,*,#14041,.F.);
#20102=ORIENTED_EDGE('',*,*,#14231,.F.);
#20103=ORIENTED_EDGE('',*,*,#14232,.F.);
#20104=ORIENTED_EDGE('',*,*,#14233,.T.);
#20105=ORIENTED_EDGE('',*,*,#14234,.T.);
#20106=ORIENTED_EDGE('',*,*,#14235,.F.);
#20107=ORIENTED_EDGE('',*,*,#14234,.F.);
#20108=ORIENTED_EDGE('',*,*,#14236,.T.);
#20109=ORIENTED_EDGE('',*,*,#14237,.F.);
#20110=ORIENTED_EDGE('',*,*,#14238,.F.);
#20111=ORIENTED_EDGE('',*,*,#14239,.F.);
#20112=ORIENTED_EDGE('',*,*,#14236,.F.);
#20113=ORIENTED_EDGE('',*,*,#14233,.F.);
#20114=ORIENTED_EDGE('',*,*,#14240,.F.);
#20115=ORIENTED_EDGE('',*,*,#14241,.T.);
#20116=ORIENTED_EDGE('',*,*,#14242,.T.);
#20117=ORIENTED_EDGE('',*,*,#14243,.F.);
#20118=ORIENTED_EDGE('',*,*,#14242,.F.);
#20119=ORIENTED_EDGE('',*,*,#14244,.T.);
#20120=ORIENTED_EDGE('',*,*,#14245,.F.);
#20121=ORIENTED_EDGE('',*,*,#14246,.F.);
#20122=ORIENTED_EDGE('',*,*,#14247,.F.);
#20123=ORIENTED_EDGE('',*,*,#14244,.F.);
#20124=ORIENTED_EDGE('',*,*,#14241,.F.);
#20125=ORIENTED_EDGE('',*,*,#14248,.F.);
#20126=ORIENTED_EDGE('',*,*,#14249,.T.);
#20127=ORIENTED_EDGE('',*,*,#14250,.T.);
#20128=ORIENTED_EDGE('',*,*,#14251,.F.);
#20129=ORIENTED_EDGE('',*,*,#14250,.F.);
#20130=ORIENTED_EDGE('',*,*,#14252,.T.);
#20131=ORIENTED_EDGE('',*,*,#14253,.F.);
#20132=ORIENTED_EDGE('',*,*,#14254,.F.);
#20133=ORIENTED_EDGE('',*,*,#14255,.F.);
#20134=ORIENTED_EDGE('',*,*,#14252,.F.);
#20135=ORIENTED_EDGE('',*,*,#14249,.F.);
#20136=ORIENTED_EDGE('',*,*,#14256,.F.);
#20137=ORIENTED_EDGE('',*,*,#14257,.T.);
#20138=ORIENTED_EDGE('',*,*,#14258,.T.);
#20139=ORIENTED_EDGE('',*,*,#14259,.F.);
#20140=ORIENTED_EDGE('',*,*,#14258,.F.);
#20141=ORIENTED_EDGE('',*,*,#14260,.T.);
#20142=ORIENTED_EDGE('',*,*,#14261,.F.);
#20143=ORIENTED_EDGE('',*,*,#14262,.F.);
#20144=ORIENTED_EDGE('',*,*,#14263,.F.);
#20145=ORIENTED_EDGE('',*,*,#14260,.F.);
#20146=ORIENTED_EDGE('',*,*,#14257,.F.);
#20147=ORIENTED_EDGE('',*,*,#14264,.F.);
#20148=ORIENTED_EDGE('',*,*,#14265,.T.);
#20149=ORIENTED_EDGE('',*,*,#14266,.T.);
#20150=ORIENTED_EDGE('',*,*,#14267,.F.);
#20151=ORIENTED_EDGE('',*,*,#14266,.F.);
#20152=ORIENTED_EDGE('',*,*,#14268,.T.);
#20153=ORIENTED_EDGE('',*,*,#14269,.F.);
#20154=ORIENTED_EDGE('',*,*,#14270,.F.);
#20155=ORIENTED_EDGE('',*,*,#14271,.F.);
#20156=ORIENTED_EDGE('',*,*,#14268,.F.);
#20157=ORIENTED_EDGE('',*,*,#14265,.F.);
#20158=ORIENTED_EDGE('',*,*,#14272,.F.);
#20159=ORIENTED_EDGE('',*,*,#14273,.T.);
#20160=ORIENTED_EDGE('',*,*,#14274,.T.);
#20161=ORIENTED_EDGE('',*,*,#14275,.F.);
#20162=ORIENTED_EDGE('',*,*,#14274,.F.);
#20163=ORIENTED_EDGE('',*,*,#14276,.T.);
#20164=ORIENTED_EDGE('',*,*,#14277,.F.);
#20165=ORIENTED_EDGE('',*,*,#14278,.F.);
#20166=ORIENTED_EDGE('',*,*,#14279,.F.);
#20167=ORIENTED_EDGE('',*,*,#14276,.F.);
#20168=ORIENTED_EDGE('',*,*,#14273,.F.);
#20169=ORIENTED_EDGE('',*,*,#14280,.F.);
#20170=ORIENTED_EDGE('',*,*,#14281,.T.);
#20171=ORIENTED_EDGE('',*,*,#14282,.T.);
#20172=ORIENTED_EDGE('',*,*,#14283,.F.);
#20173=ORIENTED_EDGE('',*,*,#14282,.F.);
#20174=ORIENTED_EDGE('',*,*,#14284,.T.);
#20175=ORIENTED_EDGE('',*,*,#14285,.F.);
#20176=ORIENTED_EDGE('',*,*,#14286,.F.);
#20177=ORIENTED_EDGE('',*,*,#14287,.F.);
#20178=ORIENTED_EDGE('',*,*,#14284,.F.);
#20179=ORIENTED_EDGE('',*,*,#14281,.F.);
#20180=ORIENTED_EDGE('',*,*,#14288,.F.);
#20181=ORIENTED_EDGE('',*,*,#14289,.T.);
#20182=ORIENTED_EDGE('',*,*,#14290,.T.);
#20183=ORIENTED_EDGE('',*,*,#14291,.F.);
#20184=ORIENTED_EDGE('',*,*,#14290,.F.);
#20185=ORIENTED_EDGE('',*,*,#14292,.T.);
#20186=ORIENTED_EDGE('',*,*,#14293,.F.);
#20187=ORIENTED_EDGE('',*,*,#14294,.F.);
#20188=ORIENTED_EDGE('',*,*,#14295,.F.);
#20189=ORIENTED_EDGE('',*,*,#14292,.F.);
#20190=ORIENTED_EDGE('',*,*,#14289,.F.);
#20191=ORIENTED_EDGE('',*,*,#14296,.F.);
#20192=ORIENTED_EDGE('',*,*,#14297,.T.);
#20193=ORIENTED_EDGE('',*,*,#14298,.T.);
#20194=ORIENTED_EDGE('',*,*,#14299,.F.);
#20195=ORIENTED_EDGE('',*,*,#14298,.F.);
#20196=ORIENTED_EDGE('',*,*,#14300,.T.);
#20197=ORIENTED_EDGE('',*,*,#14301,.F.);
#20198=ORIENTED_EDGE('',*,*,#14302,.F.);
#20199=ORIENTED_EDGE('',*,*,#14303,.F.);
#20200=ORIENTED_EDGE('',*,*,#14300,.F.);
#20201=ORIENTED_EDGE('',*,*,#14297,.F.);
#20202=ORIENTED_EDGE('',*,*,#14304,.F.);
#20203=ORIENTED_EDGE('',*,*,#14305,.T.);
#20204=ORIENTED_EDGE('',*,*,#14306,.T.);
#20205=ORIENTED_EDGE('',*,*,#14307,.F.);
#20206=ORIENTED_EDGE('',*,*,#14306,.F.);
#20207=ORIENTED_EDGE('',*,*,#14308,.T.);
#20208=ORIENTED_EDGE('',*,*,#14309,.F.);
#20209=ORIENTED_EDGE('',*,*,#14310,.F.);
#20210=ORIENTED_EDGE('',*,*,#14311,.F.);
#20211=ORIENTED_EDGE('',*,*,#14308,.F.);
#20212=ORIENTED_EDGE('',*,*,#14305,.F.);
#20213=ORIENTED_EDGE('',*,*,#14312,.F.);
#20214=ORIENTED_EDGE('',*,*,#14313,.T.);
#20215=ORIENTED_EDGE('',*,*,#14314,.T.);
#20216=ORIENTED_EDGE('',*,*,#14315,.F.);
#20217=ORIENTED_EDGE('',*,*,#14314,.F.);
#20218=ORIENTED_EDGE('',*,*,#14316,.T.);
#20219=ORIENTED_EDGE('',*,*,#14317,.F.);
#20220=ORIENTED_EDGE('',*,*,#14318,.F.);
#20221=ORIENTED_EDGE('',*,*,#14319,.F.);
#20222=ORIENTED_EDGE('',*,*,#14316,.F.);
#20223=ORIENTED_EDGE('',*,*,#14313,.F.);
#20224=ORIENTED_EDGE('',*,*,#14320,.F.);
#20225=ORIENTED_EDGE('',*,*,#14321,.T.);
#20226=ORIENTED_EDGE('',*,*,#14322,.T.);
#20227=ORIENTED_EDGE('',*,*,#14323,.F.);
#20228=ORIENTED_EDGE('',*,*,#14322,.F.);
#20229=ORIENTED_EDGE('',*,*,#14324,.T.);
#20230=ORIENTED_EDGE('',*,*,#14325,.F.);
#20231=ORIENTED_EDGE('',*,*,#14326,.F.);
#20232=ORIENTED_EDGE('',*,*,#14327,.F.);
#20233=ORIENTED_EDGE('',*,*,#14324,.F.);
#20234=ORIENTED_EDGE('',*,*,#14321,.F.);
#20235=ORIENTED_EDGE('',*,*,#14328,.F.);
#20236=ORIENTED_EDGE('',*,*,#14329,.T.);
#20237=ORIENTED_EDGE('',*,*,#14330,.T.);
#20238=ORIENTED_EDGE('',*,*,#14331,.F.);
#20239=ORIENTED_EDGE('',*,*,#14330,.F.);
#20240=ORIENTED_EDGE('',*,*,#14332,.T.);
#20241=ORIENTED_EDGE('',*,*,#14333,.F.);
#20242=ORIENTED_EDGE('',*,*,#14334,.F.);
#20243=ORIENTED_EDGE('',*,*,#14335,.F.);
#20244=ORIENTED_EDGE('',*,*,#14332,.F.);
#20245=ORIENTED_EDGE('',*,*,#14329,.F.);
#20246=ORIENTED_EDGE('',*,*,#14336,.F.);
#20247=ORIENTED_EDGE('',*,*,#14337,.T.);
#20248=ORIENTED_EDGE('',*,*,#14338,.T.);
#20249=ORIENTED_EDGE('',*,*,#14339,.F.);
#20250=ORIENTED_EDGE('',*,*,#14338,.F.);
#20251=ORIENTED_EDGE('',*,*,#14340,.T.);
#20252=ORIENTED_EDGE('',*,*,#14341,.F.);
#20253=ORIENTED_EDGE('',*,*,#14342,.F.);
#20254=ORIENTED_EDGE('',*,*,#14343,.F.);
#20255=ORIENTED_EDGE('',*,*,#14340,.F.);
#20256=ORIENTED_EDGE('',*,*,#14337,.F.);
#20257=ORIENTED_EDGE('',*,*,#14344,.F.);
#20258=ORIENTED_EDGE('',*,*,#14345,.T.);
#20259=ORIENTED_EDGE('',*,*,#14346,.T.);
#20260=ORIENTED_EDGE('',*,*,#14347,.F.);
#20261=ORIENTED_EDGE('',*,*,#14346,.F.);
#20262=ORIENTED_EDGE('',*,*,#14348,.T.);
#20263=ORIENTED_EDGE('',*,*,#14349,.F.);
#20264=ORIENTED_EDGE('',*,*,#14350,.F.);
#20265=ORIENTED_EDGE('',*,*,#14351,.F.);
#20266=ORIENTED_EDGE('',*,*,#14348,.F.);
#20267=ORIENTED_EDGE('',*,*,#14345,.F.);
#20268=ORIENTED_EDGE('',*,*,#14352,.F.);
#20269=ORIENTED_EDGE('',*,*,#14353,.T.);
#20270=ORIENTED_EDGE('',*,*,#14354,.T.);
#20271=ORIENTED_EDGE('',*,*,#14355,.F.);
#20272=ORIENTED_EDGE('',*,*,#14354,.F.);
#20273=ORIENTED_EDGE('',*,*,#14356,.T.);
#20274=ORIENTED_EDGE('',*,*,#14357,.F.);
#20275=ORIENTED_EDGE('',*,*,#14358,.F.);
#20276=ORIENTED_EDGE('',*,*,#14359,.F.);
#20277=ORIENTED_EDGE('',*,*,#14356,.F.);
#20278=ORIENTED_EDGE('',*,*,#14353,.F.);
#20279=ORIENTED_EDGE('',*,*,#14360,.F.);
#20280=ORIENTED_EDGE('',*,*,#14361,.T.);
#20281=ORIENTED_EDGE('',*,*,#14362,.T.);
#20282=ORIENTED_EDGE('',*,*,#14363,.F.);
#20283=ORIENTED_EDGE('',*,*,#14362,.F.);
#20284=ORIENTED_EDGE('',*,*,#14364,.T.);
#20285=ORIENTED_EDGE('',*,*,#14365,.F.);
#20286=ORIENTED_EDGE('',*,*,#14366,.F.);
#20287=ORIENTED_EDGE('',*,*,#14367,.F.);
#20288=ORIENTED_EDGE('',*,*,#14364,.F.);
#20289=ORIENTED_EDGE('',*,*,#14361,.F.);
#20290=ORIENTED_EDGE('',*,*,#14368,.F.);
#20291=ORIENTED_EDGE('',*,*,#14369,.T.);
#20292=ORIENTED_EDGE('',*,*,#14370,.T.);
#20293=ORIENTED_EDGE('',*,*,#14371,.F.);
#20294=ORIENTED_EDGE('',*,*,#14372,.F.);
#20295=ORIENTED_EDGE('',*,*,#14370,.F.);
#20296=ORIENTED_EDGE('',*,*,#14373,.T.);
#20297=ORIENTED_EDGE('',*,*,#14374,.F.);
#20298=ORIENTED_EDGE('',*,*,#14375,.F.);
#20299=ORIENTED_EDGE('',*,*,#14376,.F.);
#20300=ORIENTED_EDGE('',*,*,#14373,.F.);
#20301=ORIENTED_EDGE('',*,*,#14369,.F.);
#20302=ORIENTED_EDGE('',*,*,#14377,.F.);
#20303=ORIENTED_EDGE('',*,*,#14378,.T.);
#20304=ORIENTED_EDGE('',*,*,#14379,.T.);
#20305=ORIENTED_EDGE('',*,*,#14380,.F.);
#20306=ORIENTED_EDGE('',*,*,#14379,.F.);
#20307=ORIENTED_EDGE('',*,*,#14381,.T.);
#20308=ORIENTED_EDGE('',*,*,#14382,.F.);
#20309=ORIENTED_EDGE('',*,*,#14383,.F.);
#20310=ORIENTED_EDGE('',*,*,#14384,.F.);
#20311=ORIENTED_EDGE('',*,*,#14381,.F.);
#20312=ORIENTED_EDGE('',*,*,#14378,.F.);
#20313=ORIENTED_EDGE('',*,*,#14385,.F.);
#20314=ORIENTED_EDGE('',*,*,#14386,.T.);
#20315=ORIENTED_EDGE('',*,*,#14387,.T.);
#20316=ORIENTED_EDGE('',*,*,#14388,.F.);
#20317=ORIENTED_EDGE('',*,*,#14387,.F.);
#20318=ORIENTED_EDGE('',*,*,#14389,.T.);
#20319=ORIENTED_EDGE('',*,*,#14390,.F.);
#20320=ORIENTED_EDGE('',*,*,#14391,.F.);
#20321=ORIENTED_EDGE('',*,*,#14392,.F.);
#20322=ORIENTED_EDGE('',*,*,#14389,.F.);
#20323=ORIENTED_EDGE('',*,*,#14386,.F.);
#20324=ORIENTED_EDGE('',*,*,#14393,.F.);
#20325=ORIENTED_EDGE('',*,*,#14394,.T.);
#20326=ORIENTED_EDGE('',*,*,#14395,.T.);
#20327=ORIENTED_EDGE('',*,*,#14396,.F.);
#20328=ORIENTED_EDGE('',*,*,#14395,.F.);
#20329=ORIENTED_EDGE('',*,*,#14397,.T.);
#20330=ORIENTED_EDGE('',*,*,#14398,.F.);
#20331=ORIENTED_EDGE('',*,*,#14399,.F.);
#20332=ORIENTED_EDGE('',*,*,#14400,.F.);
#20333=ORIENTED_EDGE('',*,*,#14397,.F.);
#20334=ORIENTED_EDGE('',*,*,#14394,.F.);
#20335=ORIENTED_EDGE('',*,*,#14401,.F.);
#20336=ORIENTED_EDGE('',*,*,#14402,.T.);
#20337=ORIENTED_EDGE('',*,*,#14403,.T.);
#20338=ORIENTED_EDGE('',*,*,#14404,.F.);
#20339=ORIENTED_EDGE('',*,*,#14403,.F.);
#20340=ORIENTED_EDGE('',*,*,#14405,.T.);
#20341=ORIENTED_EDGE('',*,*,#14406,.F.);
#20342=ORIENTED_EDGE('',*,*,#14407,.F.);
#20343=ORIENTED_EDGE('',*,*,#14408,.F.);
#20344=ORIENTED_EDGE('',*,*,#14405,.F.);
#20345=ORIENTED_EDGE('',*,*,#14402,.F.);
#20346=ORIENTED_EDGE('',*,*,#14409,.F.);
#20347=ORIENTED_EDGE('',*,*,#14410,.T.);
#20348=ORIENTED_EDGE('',*,*,#14411,.T.);
#20349=ORIENTED_EDGE('',*,*,#14412,.F.);
#20350=ORIENTED_EDGE('',*,*,#14411,.F.);
#20351=ORIENTED_EDGE('',*,*,#14413,.T.);
#20352=ORIENTED_EDGE('',*,*,#14414,.F.);
#20353=ORIENTED_EDGE('',*,*,#14415,.F.);
#20354=ORIENTED_EDGE('',*,*,#14416,.F.);
#20355=ORIENTED_EDGE('',*,*,#14413,.F.);
#20356=ORIENTED_EDGE('',*,*,#14410,.F.);
#20357=ORIENTED_EDGE('',*,*,#14417,.F.);
#20358=ORIENTED_EDGE('',*,*,#14418,.T.);
#20359=ORIENTED_EDGE('',*,*,#14419,.T.);
#20360=ORIENTED_EDGE('',*,*,#14420,.F.);
#20361=ORIENTED_EDGE('',*,*,#14419,.F.);
#20362=ORIENTED_EDGE('',*,*,#14421,.T.);
#20363=ORIENTED_EDGE('',*,*,#14422,.F.);
#20364=ORIENTED_EDGE('',*,*,#14423,.F.);
#20365=ORIENTED_EDGE('',*,*,#14424,.F.);
#20366=ORIENTED_EDGE('',*,*,#14421,.F.);
#20367=ORIENTED_EDGE('',*,*,#14418,.F.);
#20368=ORIENTED_EDGE('',*,*,#14425,.F.);
#20369=ORIENTED_EDGE('',*,*,#14426,.T.);
#20370=ORIENTED_EDGE('',*,*,#14427,.T.);
#20371=ORIENTED_EDGE('',*,*,#14428,.F.);
#20372=ORIENTED_EDGE('',*,*,#14427,.F.);
#20373=ORIENTED_EDGE('',*,*,#14429,.T.);
#20374=ORIENTED_EDGE('',*,*,#14430,.F.);
#20375=ORIENTED_EDGE('',*,*,#14431,.F.);
#20376=ORIENTED_EDGE('',*,*,#14432,.F.);
#20377=ORIENTED_EDGE('',*,*,#14429,.F.);
#20378=ORIENTED_EDGE('',*,*,#14426,.F.);
#20379=ORIENTED_EDGE('',*,*,#14433,.F.);
#20380=ORIENTED_EDGE('',*,*,#14434,.T.);
#20381=ORIENTED_EDGE('',*,*,#14435,.T.);
#20382=ORIENTED_EDGE('',*,*,#14436,.F.);
#20383=ORIENTED_EDGE('',*,*,#14435,.F.);
#20384=ORIENTED_EDGE('',*,*,#14437,.T.);
#20385=ORIENTED_EDGE('',*,*,#14438,.F.);
#20386=ORIENTED_EDGE('',*,*,#14439,.F.);
#20387=ORIENTED_EDGE('',*,*,#14440,.F.);
#20388=ORIENTED_EDGE('',*,*,#14437,.F.);
#20389=ORIENTED_EDGE('',*,*,#14434,.F.);
#20390=ORIENTED_EDGE('',*,*,#14441,.F.);
#20391=ORIENTED_EDGE('',*,*,#14442,.T.);
#20392=ORIENTED_EDGE('',*,*,#14443,.T.);
#20393=ORIENTED_EDGE('',*,*,#14444,.F.);
#20394=ORIENTED_EDGE('',*,*,#14443,.F.);
#20395=ORIENTED_EDGE('',*,*,#14445,.T.);
#20396=ORIENTED_EDGE('',*,*,#14446,.F.);
#20397=ORIENTED_EDGE('',*,*,#14447,.F.);
#20398=ORIENTED_EDGE('',*,*,#14448,.F.);
#20399=ORIENTED_EDGE('',*,*,#14445,.F.);
#20400=ORIENTED_EDGE('',*,*,#14442,.F.);
#20401=ORIENTED_EDGE('',*,*,#14449,.F.);
#20402=ORIENTED_EDGE('',*,*,#14450,.T.);
#20403=ORIENTED_EDGE('',*,*,#14451,.T.);
#20404=ORIENTED_EDGE('',*,*,#14452,.F.);
#20405=ORIENTED_EDGE('',*,*,#14451,.F.);
#20406=ORIENTED_EDGE('',*,*,#14453,.T.);
#20407=ORIENTED_EDGE('',*,*,#14454,.F.);
#20408=ORIENTED_EDGE('',*,*,#14455,.F.);
#20409=ORIENTED_EDGE('',*,*,#14456,.F.);
#20410=ORIENTED_EDGE('',*,*,#14453,.F.);
#20411=ORIENTED_EDGE('',*,*,#14450,.F.);
#20412=ORIENTED_EDGE('',*,*,#14457,.F.);
#20413=ORIENTED_EDGE('',*,*,#14458,.T.);
#20414=ORIENTED_EDGE('',*,*,#14459,.T.);
#20415=ORIENTED_EDGE('',*,*,#14460,.F.);
#20416=ORIENTED_EDGE('',*,*,#14459,.F.);
#20417=ORIENTED_EDGE('',*,*,#14461,.T.);
#20418=ORIENTED_EDGE('',*,*,#14462,.F.);
#20419=ORIENTED_EDGE('',*,*,#14463,.F.);
#20420=ORIENTED_EDGE('',*,*,#14464,.F.);
#20421=ORIENTED_EDGE('',*,*,#14461,.F.);
#20422=ORIENTED_EDGE('',*,*,#14458,.F.);
#20423=ORIENTED_EDGE('',*,*,#14465,.F.);
#20424=ORIENTED_EDGE('',*,*,#14466,.T.);
#20425=ORIENTED_EDGE('',*,*,#14467,.T.);
#20426=ORIENTED_EDGE('',*,*,#14468,.F.);
#20427=ORIENTED_EDGE('',*,*,#14467,.F.);
#20428=ORIENTED_EDGE('',*,*,#14469,.T.);
#20429=ORIENTED_EDGE('',*,*,#14470,.F.);
#20430=ORIENTED_EDGE('',*,*,#14471,.F.);
#20431=ORIENTED_EDGE('',*,*,#14472,.F.);
#20432=ORIENTED_EDGE('',*,*,#14469,.F.);
#20433=ORIENTED_EDGE('',*,*,#14466,.F.);
#20434=ORIENTED_EDGE('',*,*,#14473,.F.);
#20435=ORIENTED_EDGE('',*,*,#14474,.T.);
#20436=ORIENTED_EDGE('',*,*,#14475,.T.);
#20437=ORIENTED_EDGE('',*,*,#14476,.F.);
#20438=ORIENTED_EDGE('',*,*,#14475,.F.);
#20439=ORIENTED_EDGE('',*,*,#14477,.T.);
#20440=ORIENTED_EDGE('',*,*,#14478,.F.);
#20441=ORIENTED_EDGE('',*,*,#14479,.F.);
#20442=ORIENTED_EDGE('',*,*,#14480,.F.);
#20443=ORIENTED_EDGE('',*,*,#14477,.F.);
#20444=ORIENTED_EDGE('',*,*,#14474,.F.);
#20445=ORIENTED_EDGE('',*,*,#14481,.F.);
#20446=ORIENTED_EDGE('',*,*,#14482,.T.);
#20447=ORIENTED_EDGE('',*,*,#14483,.T.);
#20448=ORIENTED_EDGE('',*,*,#14484,.F.);
#20449=ORIENTED_EDGE('',*,*,#14483,.F.);
#20450=ORIENTED_EDGE('',*,*,#14485,.T.);
#20451=ORIENTED_EDGE('',*,*,#14486,.F.);
#20452=ORIENTED_EDGE('',*,*,#14487,.F.);
#20453=ORIENTED_EDGE('',*,*,#14488,.F.);
#20454=ORIENTED_EDGE('',*,*,#14485,.F.);
#20455=ORIENTED_EDGE('',*,*,#14482,.F.);
#20456=ORIENTED_EDGE('',*,*,#14489,.F.);
#20457=ORIENTED_EDGE('',*,*,#14490,.T.);
#20458=ORIENTED_EDGE('',*,*,#14491,.T.);
#20459=ORIENTED_EDGE('',*,*,#14492,.F.);
#20460=ORIENTED_EDGE('',*,*,#14491,.F.);
#20461=ORIENTED_EDGE('',*,*,#14493,.T.);
#20462=ORIENTED_EDGE('',*,*,#14494,.F.);
#20463=ORIENTED_EDGE('',*,*,#14495,.F.);
#20464=ORIENTED_EDGE('',*,*,#14496,.F.);
#20465=ORIENTED_EDGE('',*,*,#14493,.F.);
#20466=ORIENTED_EDGE('',*,*,#14490,.F.);
#20467=ORIENTED_EDGE('',*,*,#14497,.F.);
#20468=ORIENTED_EDGE('',*,*,#14498,.T.);
#20469=ORIENTED_EDGE('',*,*,#14499,.T.);
#20470=ORIENTED_EDGE('',*,*,#14500,.F.);
#20471=ORIENTED_EDGE('',*,*,#14499,.F.);
#20472=ORIENTED_EDGE('',*,*,#14501,.T.);
#20473=ORIENTED_EDGE('',*,*,#14502,.F.);
#20474=ORIENTED_EDGE('',*,*,#14503,.F.);
#20475=ORIENTED_EDGE('',*,*,#14504,.F.);
#20476=ORIENTED_EDGE('',*,*,#14501,.F.);
#20477=ORIENTED_EDGE('',*,*,#14498,.F.);
#20478=ORIENTED_EDGE('',*,*,#14505,.F.);
#20479=ORIENTED_EDGE('',*,*,#14506,.T.);
#20480=ORIENTED_EDGE('',*,*,#14507,.T.);
#20481=ORIENTED_EDGE('',*,*,#14508,.F.);
#20482=ORIENTED_EDGE('',*,*,#14507,.F.);
#20483=ORIENTED_EDGE('',*,*,#14509,.T.);
#20484=ORIENTED_EDGE('',*,*,#14510,.F.);
#20485=ORIENTED_EDGE('',*,*,#14511,.F.);
#20486=ORIENTED_EDGE('',*,*,#14512,.F.);
#20487=ORIENTED_EDGE('',*,*,#14509,.F.);
#20488=ORIENTED_EDGE('',*,*,#14506,.F.);
#20489=ORIENTED_EDGE('',*,*,#14238,.T.);
#20490=ORIENTED_EDGE('',*,*,#14232,.T.);
#20491=ORIENTED_EDGE('',*,*,#14235,.T.);
#20492=ORIENTED_EDGE('',*,*,#14513,.F.);
#20493=ORIENTED_EDGE('',*,*,#14246,.T.);
#20494=ORIENTED_EDGE('',*,*,#14240,.T.);
#20495=ORIENTED_EDGE('',*,*,#14243,.T.);
#20496=ORIENTED_EDGE('',*,*,#14514,.F.);
#20497=ORIENTED_EDGE('',*,*,#14254,.T.);
#20498=ORIENTED_EDGE('',*,*,#14248,.T.);
#20499=ORIENTED_EDGE('',*,*,#14251,.T.);
#20500=ORIENTED_EDGE('',*,*,#14515,.F.);
#20501=ORIENTED_EDGE('',*,*,#14262,.T.);
#20502=ORIENTED_EDGE('',*,*,#14256,.T.);
#20503=ORIENTED_EDGE('',*,*,#14259,.T.);
#20504=ORIENTED_EDGE('',*,*,#14516,.F.);
#20505=ORIENTED_EDGE('',*,*,#14270,.T.);
#20506=ORIENTED_EDGE('',*,*,#14264,.T.);
#20507=ORIENTED_EDGE('',*,*,#14267,.T.);
#20508=ORIENTED_EDGE('',*,*,#14517,.F.);
#20509=ORIENTED_EDGE('',*,*,#14278,.T.);
#20510=ORIENTED_EDGE('',*,*,#14272,.T.);
#20511=ORIENTED_EDGE('',*,*,#14275,.T.);
#20512=ORIENTED_EDGE('',*,*,#14518,.F.);
#20513=ORIENTED_EDGE('',*,*,#14286,.T.);
#20514=ORIENTED_EDGE('',*,*,#14280,.T.);
#20515=ORIENTED_EDGE('',*,*,#14283,.T.);
#20516=ORIENTED_EDGE('',*,*,#14519,.F.);
#20517=ORIENTED_EDGE('',*,*,#14294,.T.);
#20518=ORIENTED_EDGE('',*,*,#14288,.T.);
#20519=ORIENTED_EDGE('',*,*,#14291,.T.);
#20520=ORIENTED_EDGE('',*,*,#14520,.F.);
#20521=ORIENTED_EDGE('',*,*,#14302,.T.);
#20522=ORIENTED_EDGE('',*,*,#14296,.T.);
#20523=ORIENTED_EDGE('',*,*,#14299,.T.);
#20524=ORIENTED_EDGE('',*,*,#14521,.F.);
#20525=ORIENTED_EDGE('',*,*,#14310,.T.);
#20526=ORIENTED_EDGE('',*,*,#14304,.T.);
#20527=ORIENTED_EDGE('',*,*,#14307,.T.);
#20528=ORIENTED_EDGE('',*,*,#14522,.F.);
#20529=ORIENTED_EDGE('',*,*,#14318,.T.);
#20530=ORIENTED_EDGE('',*,*,#14312,.T.);
#20531=ORIENTED_EDGE('',*,*,#14315,.T.);
#20532=ORIENTED_EDGE('',*,*,#14523,.F.);
#20533=ORIENTED_EDGE('',*,*,#14326,.T.);
#20534=ORIENTED_EDGE('',*,*,#14320,.T.);
#20535=ORIENTED_EDGE('',*,*,#14323,.T.);
#20536=ORIENTED_EDGE('',*,*,#14524,.F.);
#20537=ORIENTED_EDGE('',*,*,#14334,.T.);
#20538=ORIENTED_EDGE('',*,*,#14328,.T.);
#20539=ORIENTED_EDGE('',*,*,#14331,.T.);
#20540=ORIENTED_EDGE('',*,*,#14525,.F.);
#20541=ORIENTED_EDGE('',*,*,#14342,.T.);
#20542=ORIENTED_EDGE('',*,*,#14336,.T.);
#20543=ORIENTED_EDGE('',*,*,#14339,.T.);
#20544=ORIENTED_EDGE('',*,*,#14526,.F.);
#20545=ORIENTED_EDGE('',*,*,#14350,.T.);
#20546=ORIENTED_EDGE('',*,*,#14344,.T.);
#20547=ORIENTED_EDGE('',*,*,#14347,.T.);
#20548=ORIENTED_EDGE('',*,*,#14527,.F.);
#20549=ORIENTED_EDGE('',*,*,#14358,.T.);
#20550=ORIENTED_EDGE('',*,*,#14352,.T.);
#20551=ORIENTED_EDGE('',*,*,#14355,.T.);
#20552=ORIENTED_EDGE('',*,*,#14528,.F.);
#20553=ORIENTED_EDGE('',*,*,#14366,.T.);
#20554=ORIENTED_EDGE('',*,*,#14360,.T.);
#20555=ORIENTED_EDGE('',*,*,#14363,.T.);
#20556=ORIENTED_EDGE('',*,*,#14529,.F.);
#20557=ORIENTED_EDGE('',*,*,#14375,.T.);
#20558=ORIENTED_EDGE('',*,*,#14368,.T.);
#20559=ORIENTED_EDGE('',*,*,#14530,.T.);
#20560=ORIENTED_EDGE('',*,*,#14531,.T.);
#20561=ORIENTED_EDGE('',*,*,#14530,.F.);
#20562=ORIENTED_EDGE('',*,*,#14371,.T.);
#20563=ORIENTED_EDGE('',*,*,#14372,.T.);
#20564=ORIENTED_EDGE('',*,*,#14532,.F.);
#20565=ORIENTED_EDGE('',*,*,#14383,.T.);
#20566=ORIENTED_EDGE('',*,*,#14377,.T.);
#20567=ORIENTED_EDGE('',*,*,#14380,.T.);
#20568=ORIENTED_EDGE('',*,*,#14533,.F.);
#20569=ORIENTED_EDGE('',*,*,#14391,.T.);
#20570=ORIENTED_EDGE('',*,*,#14385,.T.);
#20571=ORIENTED_EDGE('',*,*,#14388,.T.);
#20572=ORIENTED_EDGE('',*,*,#14534,.F.);
#20573=ORIENTED_EDGE('',*,*,#14399,.T.);
#20574=ORIENTED_EDGE('',*,*,#14393,.T.);
#20575=ORIENTED_EDGE('',*,*,#14396,.T.);
#20576=ORIENTED_EDGE('',*,*,#14535,.F.);
#20577=ORIENTED_EDGE('',*,*,#14407,.T.);
#20578=ORIENTED_EDGE('',*,*,#14401,.T.);
#20579=ORIENTED_EDGE('',*,*,#14404,.T.);
#20580=ORIENTED_EDGE('',*,*,#14536,.F.);
#20581=ORIENTED_EDGE('',*,*,#14415,.T.);
#20582=ORIENTED_EDGE('',*,*,#14409,.T.);
#20583=ORIENTED_EDGE('',*,*,#14412,.T.);
#20584=ORIENTED_EDGE('',*,*,#14537,.F.);
#20585=ORIENTED_EDGE('',*,*,#14423,.T.);
#20586=ORIENTED_EDGE('',*,*,#14417,.T.);
#20587=ORIENTED_EDGE('',*,*,#14420,.T.);
#20588=ORIENTED_EDGE('',*,*,#14538,.F.);
#20589=ORIENTED_EDGE('',*,*,#14431,.T.);
#20590=ORIENTED_EDGE('',*,*,#14425,.T.);
#20591=ORIENTED_EDGE('',*,*,#14428,.T.);
#20592=ORIENTED_EDGE('',*,*,#14539,.F.);
#20593=ORIENTED_EDGE('',*,*,#14439,.T.);
#20594=ORIENTED_EDGE('',*,*,#14433,.T.);
#20595=ORIENTED_EDGE('',*,*,#14436,.T.);
#20596=ORIENTED_EDGE('',*,*,#14540,.F.);
#20597=ORIENTED_EDGE('',*,*,#14447,.T.);
#20598=ORIENTED_EDGE('',*,*,#14441,.T.);
#20599=ORIENTED_EDGE('',*,*,#14444,.T.);
#20600=ORIENTED_EDGE('',*,*,#14541,.F.);
#20601=ORIENTED_EDGE('',*,*,#14455,.T.);
#20602=ORIENTED_EDGE('',*,*,#14449,.T.);
#20603=ORIENTED_EDGE('',*,*,#14452,.T.);
#20604=ORIENTED_EDGE('',*,*,#14542,.F.);
#20605=ORIENTED_EDGE('',*,*,#14463,.T.);
#20606=ORIENTED_EDGE('',*,*,#14457,.T.);
#20607=ORIENTED_EDGE('',*,*,#14460,.T.);
#20608=ORIENTED_EDGE('',*,*,#14543,.F.);
#20609=ORIENTED_EDGE('',*,*,#14471,.T.);
#20610=ORIENTED_EDGE('',*,*,#14465,.T.);
#20611=ORIENTED_EDGE('',*,*,#14468,.T.);
#20612=ORIENTED_EDGE('',*,*,#14544,.F.);
#20613=ORIENTED_EDGE('',*,*,#14479,.T.);
#20614=ORIENTED_EDGE('',*,*,#14473,.T.);
#20615=ORIENTED_EDGE('',*,*,#14476,.T.);
#20616=ORIENTED_EDGE('',*,*,#14545,.F.);
#20617=ORIENTED_EDGE('',*,*,#14487,.T.);
#20618=ORIENTED_EDGE('',*,*,#14481,.T.);
#20619=ORIENTED_EDGE('',*,*,#14484,.T.);
#20620=ORIENTED_EDGE('',*,*,#14546,.F.);
#20621=ORIENTED_EDGE('',*,*,#14495,.T.);
#20622=ORIENTED_EDGE('',*,*,#14489,.T.);
#20623=ORIENTED_EDGE('',*,*,#14492,.T.);
#20624=ORIENTED_EDGE('',*,*,#14547,.F.);
#20625=ORIENTED_EDGE('',*,*,#14503,.T.);
#20626=ORIENTED_EDGE('',*,*,#14497,.T.);
#20627=ORIENTED_EDGE('',*,*,#14500,.T.);
#20628=ORIENTED_EDGE('',*,*,#14548,.F.);
#20629=ORIENTED_EDGE('',*,*,#14511,.T.);
#20630=ORIENTED_EDGE('',*,*,#14505,.T.);
#20631=ORIENTED_EDGE('',*,*,#14508,.T.);
#20632=ORIENTED_EDGE('',*,*,#14549,.F.);
#20633=ORIENTED_EDGE('',*,*,#14550,.T.);
#20634=ORIENTED_EDGE('',*,*,#14551,.T.);
#20635=ORIENTED_EDGE('',*,*,#14552,.T.);
#20636=ORIENTED_EDGE('',*,*,#14553,.F.);
#20637=ORIENTED_EDGE('',*,*,#14552,.F.);
#20638=ORIENTED_EDGE('',*,*,#14554,.F.);
#20639=ORIENTED_EDGE('',*,*,#14555,.T.);
#20640=ORIENTED_EDGE('',*,*,#14556,.F.);
#20641=ORIENTED_EDGE('',*,*,#14557,.F.);
#20642=ORIENTED_EDGE('',*,*,#14555,.F.);
#20643=ORIENTED_EDGE('',*,*,#14558,.F.);
#20644=ORIENTED_EDGE('',*,*,#14550,.F.);
#20645=ORIENTED_EDGE('',*,*,#14551,.F.);
#20646=ORIENTED_EDGE('',*,*,#14558,.T.);
#20647=ORIENTED_EDGE('',*,*,#14554,.T.);
#20648=ORIENTED_EDGE('',*,*,#14559,.F.);
#20649=ORIENTED_EDGE('',*,*,#14560,.T.);
#20650=ORIENTED_EDGE('',*,*,#14376,.T.);
#20651=ORIENTED_EDGE('',*,*,#14529,.T.);
#20652=ORIENTED_EDGE('',*,*,#14365,.T.);
#20653=ORIENTED_EDGE('',*,*,#14367,.T.);
#20654=ORIENTED_EDGE('',*,*,#14528,.T.);
#20655=ORIENTED_EDGE('',*,*,#14357,.T.);
#20656=ORIENTED_EDGE('',*,*,#14359,.T.);
#20657=ORIENTED_EDGE('',*,*,#14527,.T.);
#20658=ORIENTED_EDGE('',*,*,#14349,.T.);
#20659=ORIENTED_EDGE('',*,*,#14351,.T.);
#20660=ORIENTED_EDGE('',*,*,#14526,.T.);
#20661=ORIENTED_EDGE('',*,*,#14341,.T.);
#20662=ORIENTED_EDGE('',*,*,#14343,.T.);
#20663=ORIENTED_EDGE('',*,*,#14525,.T.);
#20664=ORIENTED_EDGE('',*,*,#14333,.T.);
#20665=ORIENTED_EDGE('',*,*,#14335,.T.);
#20666=ORIENTED_EDGE('',*,*,#14524,.T.);
#20667=ORIENTED_EDGE('',*,*,#14325,.T.);
#20668=ORIENTED_EDGE('',*,*,#14327,.T.);
#20669=ORIENTED_EDGE('',*,*,#14523,.T.);
#20670=ORIENTED_EDGE('',*,*,#14317,.T.);
#20671=ORIENTED_EDGE('',*,*,#14319,.T.);
#20672=ORIENTED_EDGE('',*,*,#14522,.T.);
#20673=ORIENTED_EDGE('',*,*,#14309,.T.);
#20674=ORIENTED_EDGE('',*,*,#14311,.T.);
#20675=ORIENTED_EDGE('',*,*,#14521,.T.);
#20676=ORIENTED_EDGE('',*,*,#14301,.T.);
#20677=ORIENTED_EDGE('',*,*,#14303,.T.);
#20678=ORIENTED_EDGE('',*,*,#14520,.T.);
#20679=ORIENTED_EDGE('',*,*,#14293,.T.);
#20680=ORIENTED_EDGE('',*,*,#14295,.T.);
#20681=ORIENTED_EDGE('',*,*,#14519,.T.);
#20682=ORIENTED_EDGE('',*,*,#14285,.T.);
#20683=ORIENTED_EDGE('',*,*,#14287,.T.);
#20684=ORIENTED_EDGE('',*,*,#14518,.T.);
#20685=ORIENTED_EDGE('',*,*,#14277,.T.);
#20686=ORIENTED_EDGE('',*,*,#14279,.T.);
#20687=ORIENTED_EDGE('',*,*,#14517,.T.);
#20688=ORIENTED_EDGE('',*,*,#14269,.T.);
#20689=ORIENTED_EDGE('',*,*,#14271,.T.);
#20690=ORIENTED_EDGE('',*,*,#14516,.T.);
#20691=ORIENTED_EDGE('',*,*,#14261,.T.);
#20692=ORIENTED_EDGE('',*,*,#14263,.T.);
#20693=ORIENTED_EDGE('',*,*,#14515,.T.);
#20694=ORIENTED_EDGE('',*,*,#14253,.T.);
#20695=ORIENTED_EDGE('',*,*,#14255,.T.);
#20696=ORIENTED_EDGE('',*,*,#14514,.T.);
#20697=ORIENTED_EDGE('',*,*,#14245,.T.);
#20698=ORIENTED_EDGE('',*,*,#14247,.T.);
#20699=ORIENTED_EDGE('',*,*,#14513,.T.);
#20700=ORIENTED_EDGE('',*,*,#14237,.T.);
#20701=ORIENTED_EDGE('',*,*,#14239,.T.);
#20702=ORIENTED_EDGE('',*,*,#14553,.T.);
#20703=ORIENTED_EDGE('',*,*,#14556,.T.);
#20704=ORIENTED_EDGE('',*,*,#14557,.T.);
#20705=ORIENTED_EDGE('',*,*,#14549,.T.);
#20706=ORIENTED_EDGE('',*,*,#14510,.T.);
#20707=ORIENTED_EDGE('',*,*,#14512,.T.);
#20708=ORIENTED_EDGE('',*,*,#14548,.T.);
#20709=ORIENTED_EDGE('',*,*,#14502,.T.);
#20710=ORIENTED_EDGE('',*,*,#14504,.T.);
#20711=ORIENTED_EDGE('',*,*,#14547,.T.);
#20712=ORIENTED_EDGE('',*,*,#14494,.T.);
#20713=ORIENTED_EDGE('',*,*,#14496,.T.);
#20714=ORIENTED_EDGE('',*,*,#14546,.T.);
#20715=ORIENTED_EDGE('',*,*,#14486,.T.);
#20716=ORIENTED_EDGE('',*,*,#14488,.T.);
#20717=ORIENTED_EDGE('',*,*,#14545,.T.);
#20718=ORIENTED_EDGE('',*,*,#14478,.T.);
#20719=ORIENTED_EDGE('',*,*,#14480,.T.);
#20720=ORIENTED_EDGE('',*,*,#14544,.T.);
#20721=ORIENTED_EDGE('',*,*,#14470,.T.);
#20722=ORIENTED_EDGE('',*,*,#14472,.T.);
#20723=ORIENTED_EDGE('',*,*,#14543,.T.);
#20724=ORIENTED_EDGE('',*,*,#14462,.T.);
#20725=ORIENTED_EDGE('',*,*,#14464,.T.);
#20726=ORIENTED_EDGE('',*,*,#14542,.T.);
#20727=ORIENTED_EDGE('',*,*,#14454,.T.);
#20728=ORIENTED_EDGE('',*,*,#14456,.T.);
#20729=ORIENTED_EDGE('',*,*,#14541,.T.);
#20730=ORIENTED_EDGE('',*,*,#14446,.T.);
#20731=ORIENTED_EDGE('',*,*,#14448,.T.);
#20732=ORIENTED_EDGE('',*,*,#14540,.T.);
#20733=ORIENTED_EDGE('',*,*,#14438,.T.);
#20734=ORIENTED_EDGE('',*,*,#14440,.T.);
#20735=ORIENTED_EDGE('',*,*,#14539,.T.);
#20736=ORIENTED_EDGE('',*,*,#14430,.T.);
#20737=ORIENTED_EDGE('',*,*,#14432,.T.);
#20738=ORIENTED_EDGE('',*,*,#14538,.T.);
#20739=ORIENTED_EDGE('',*,*,#14422,.T.);
#20740=ORIENTED_EDGE('',*,*,#14424,.T.);
#20741=ORIENTED_EDGE('',*,*,#14537,.T.);
#20742=ORIENTED_EDGE('',*,*,#14414,.T.);
#20743=ORIENTED_EDGE('',*,*,#14416,.T.);
#20744=ORIENTED_EDGE('',*,*,#14536,.T.);
#20745=ORIENTED_EDGE('',*,*,#14406,.T.);
#20746=ORIENTED_EDGE('',*,*,#14408,.T.);
#20747=ORIENTED_EDGE('',*,*,#14535,.T.);
#20748=ORIENTED_EDGE('',*,*,#14398,.T.);
#20749=ORIENTED_EDGE('',*,*,#14400,.T.);
#20750=ORIENTED_EDGE('',*,*,#14534,.T.);
#20751=ORIENTED_EDGE('',*,*,#14390,.T.);
#20752=ORIENTED_EDGE('',*,*,#14392,.T.);
#20753=ORIENTED_EDGE('',*,*,#14533,.T.);
#20754=ORIENTED_EDGE('',*,*,#14382,.T.);
#20755=ORIENTED_EDGE('',*,*,#14384,.T.);
#20756=ORIENTED_EDGE('',*,*,#14532,.T.);
#20757=ORIENTED_EDGE('',*,*,#14374,.T.);
#20758=ORIENTED_EDGE('',*,*,#14560,.F.);
#20759=ORIENTED_EDGE('',*,*,#14561,.T.);
#20760=ORIENTED_EDGE('',*,*,#14562,.F.);
#20761=ORIENTED_EDGE('',*,*,#14561,.F.);
#20762=ORIENTED_EDGE('',*,*,#14563,.F.);
#20763=ORIENTED_EDGE('',*,*,#14564,.T.);
#20764=ORIENTED_EDGE('',*,*,#14565,.T.);
#20765=ORIENTED_EDGE('',*,*,#14566,.F.);
#20766=ORIENTED_EDGE('',*,*,#14567,.F.);
#20767=ORIENTED_EDGE('',*,*,#14568,.T.);
#20768=ORIENTED_EDGE('',*,*,#14569,.T.);
#20769=ORIENTED_EDGE('',*,*,#14564,.F.);
#20770=ORIENTED_EDGE('',*,*,#14570,.F.);
#20771=ORIENTED_EDGE('',*,*,#14571,.T.);
#20772=ORIENTED_EDGE('',*,*,#14572,.T.);
#20773=ORIENTED_EDGE('',*,*,#14568,.F.);
#20774=ORIENTED_EDGE('',*,*,#14573,.F.);
#20775=ORIENTED_EDGE('',*,*,#14574,.T.);
#20776=ORIENTED_EDGE('',*,*,#14575,.T.);
#20777=ORIENTED_EDGE('',*,*,#14571,.F.);
#20778=ORIENTED_EDGE('',*,*,#14576,.F.);
#20779=ORIENTED_EDGE('',*,*,#14577,.T.);
#20780=ORIENTED_EDGE('',*,*,#14578,.T.);
#20781=ORIENTED_EDGE('',*,*,#14574,.F.);
#20782=ORIENTED_EDGE('',*,*,#14579,.F.);
#20783=ORIENTED_EDGE('',*,*,#14566,.T.);
#20784=ORIENTED_EDGE('',*,*,#14580,.T.);
#20785=ORIENTED_EDGE('',*,*,#14577,.F.);
#20786=ORIENTED_EDGE('',*,*,#14580,.F.);
#20787=ORIENTED_EDGE('',*,*,#14565,.F.);
#20788=ORIENTED_EDGE('',*,*,#14569,.F.);
#20789=ORIENTED_EDGE('',*,*,#14572,.F.);
#20790=ORIENTED_EDGE('',*,*,#14575,.F.);
#20791=ORIENTED_EDGE('',*,*,#14578,.F.);
#20792=ORIENTED_EDGE('',*,*,#14562,.T.);
#20793=ORIENTED_EDGE('',*,*,#14581,.F.);
#20794=ORIENTED_EDGE('',*,*,#13869,.F.);
#20795=ORIENTED_EDGE('',*,*,#14582,.T.);
#20796=ORIENTED_EDGE('',*,*,#14581,.T.);
#20797=ORIENTED_EDGE('',*,*,#14582,.F.);
#20798=ORIENTED_EDGE('',*,*,#14040,.T.);
#20799=ORIENTED_EDGE('',*,*,#14225,.T.);
#20800=ORIENTED_EDGE('',*,*,#14583,.F.);
#20801=ORIENTED_EDGE('',*,*,#14231,.T.);
#20802=ORIENTED_EDGE('',*,*,#14584,.F.);
#20803=ORIENTED_EDGE('',*,*,#14585,.T.);
#20804=ORIENTED_EDGE('',*,*,#14222,.T.);
#20805=ORIENTED_EDGE('',*,*,#14583,.T.);
#20806=ORIENTED_EDGE('',*,*,#14223,.T.);
#20807=ORIENTED_EDGE('',*,*,#14585,.F.);
#20808=ORIENTED_EDGE('',*,*,#14531,.F.);
#20809=ORIENTED_EDGE('',*,*,#14584,.T.);
#20810=ORIENTED_EDGE('',*,*,#14559,.T.);
#20811=ORIENTED_EDGE('',*,*,#14563,.T.);
#20812=ORIENTED_EDGE('',*,*,#14579,.T.);
#20813=ORIENTED_EDGE('',*,*,#14576,.T.);
#20814=ORIENTED_EDGE('',*,*,#14573,.T.);
#20815=ORIENTED_EDGE('',*,*,#14570,.T.);
#20816=ORIENTED_EDGE('',*,*,#14567,.T.);
#21967=CONICAL_SURFACE('',#25349,0.2675,0.78539816339745);
#21968=CONICAL_SURFACE('',#25351,0.0577350269189626,1.00599363799961);
#21969=CONICAL_SURFACE('',#25362,0.132,0.785398163397448);
#21970=CONICAL_SURFACE('',#25365,0.155,0.785398163397449);
#22891=ADVANCED_FACE('',(#3152),#1117,.T.);
#22892=ADVANCED_FACE('',(#3153),#1118,.T.);
#22893=ADVANCED_FACE('',(#3154),#1119,.T.);
#22894=ADVANCED_FACE('',(#3155),#1120,.T.);
#22895=ADVANCED_FACE('',(#3156),#1121,.T.);
#22896=ADVANCED_FACE('',(#3157),#1122,.T.);
#22897=ADVANCED_FACE('',(#3158),#1123,.T.);
#22898=ADVANCED_FACE('',(#3159),#1124,.T.);
#22899=ADVANCED_FACE('',(#3160),#1125,.T.);
#22900=ADVANCED_FACE('',(#3161),#1126,.T.);
#22901=ADVANCED_FACE('',(#3162),#1127,.T.);
#22902=ADVANCED_FACE('',(#3163),#1128,.T.);
#22903=ADVANCED_FACE('',(#3164),#1129,.T.);
#22904=ADVANCED_FACE('',(#3165),#1130,.T.);
#22905=ADVANCED_FACE('',(#3166),#1131,.T.);
#22906=ADVANCED_FACE('',(#3167),#1132,.T.);
#22907=ADVANCED_FACE('',(#3168),#1133,.T.);
#22908=ADVANCED_FACE('',(#3169),#1134,.T.);
#22909=ADVANCED_FACE('',(#3170),#1135,.T.);
#22910=ADVANCED_FACE('',(#3171),#1136,.T.);
#22911=ADVANCED_FACE('',(#3172),#1137,.T.);
#22912=ADVANCED_FACE('',(#3173),#1138,.T.);
#22913=ADVANCED_FACE('',(#3174),#1139,.T.);
#22914=ADVANCED_FACE('',(#3175),#1140,.T.);
#22915=ADVANCED_FACE('',(#3176),#1141,.T.);
#22916=ADVANCED_FACE('',(#3177),#1142,.T.);
#22917=ADVANCED_FACE('',(#3178),#1143,.T.);
#22918=ADVANCED_FACE('',(#3179),#1144,.T.);
#22919=ADVANCED_FACE('',(#3180),#1145,.T.);
#22920=ADVANCED_FACE('',(#3181),#1146,.T.);
#22921=ADVANCED_FACE('',(#3182),#1147,.T.);
#22922=ADVANCED_FACE('',(#3183),#1148,.T.);
#22923=ADVANCED_FACE('',(#3184),#1149,.T.);
#22924=ADVANCED_FACE('',(#3185),#1150,.T.);
#22925=ADVANCED_FACE('',(#3186),#1151,.T.);
#22926=ADVANCED_FACE('',(#3187),#1152,.T.);
#22927=ADVANCED_FACE('',(#3188),#1153,.T.);
#22928=ADVANCED_FACE('',(#3189),#1154,.T.);
#22929=ADVANCED_FACE('',(#3190),#1155,.T.);
#22930=ADVANCED_FACE('',(#3191),#1156,.T.);
#22931=ADVANCED_FACE('',(#3192),#1157,.T.);
#22932=ADVANCED_FACE('',(#3193),#1158,.T.);
#22933=ADVANCED_FACE('',(#3194),#1159,.T.);
#22934=ADVANCED_FACE('',(#3195),#1160,.T.);
#22935=ADVANCED_FACE('',(#3196),#1161,.T.);
#22936=ADVANCED_FACE('',(#3197),#1162,.T.);
#22937=ADVANCED_FACE('',(#3198),#1163,.T.);
#22938=ADVANCED_FACE('',(#3199),#1164,.T.);
#22939=ADVANCED_FACE('',(#3200),#1165,.T.);
#22940=ADVANCED_FACE('',(#3201),#1166,.T.);
#22941=ADVANCED_FACE('',(#3202),#1167,.T.);
#22942=ADVANCED_FACE('',(#3203),#1168,.T.);
#22943=ADVANCED_FACE('',(#3204),#1169,.T.);
#22944=ADVANCED_FACE('',(#3205),#1170,.T.);
#22945=ADVANCED_FACE('',(#3206),#1171,.T.);
#22946=ADVANCED_FACE('',(#3207),#1172,.T.);
#22947=ADVANCED_FACE('',(#3208),#1173,.T.);
#22948=ADVANCED_FACE('',(#3209),#1174,.T.);
#22949=ADVANCED_FACE('',(#3210),#1175,.T.);
#22950=ADVANCED_FACE('',(#3211),#1176,.T.);
#22951=ADVANCED_FACE('',(#3212),#1177,.T.);
#22952=ADVANCED_FACE('',(#3213),#1178,.T.);
#22953=ADVANCED_FACE('',(#3214),#1179,.T.);
#22954=ADVANCED_FACE('',(#3215),#1180,.T.);
#22955=ADVANCED_FACE('',(#3216),#1181,.T.);
#22956=ADVANCED_FACE('',(#3217),#1182,.T.);
#22957=ADVANCED_FACE('',(#3218),#1183,.T.);
#22958=ADVANCED_FACE('',(#3219),#1184,.T.);
#22959=ADVANCED_FACE('',(#3220),#1185,.T.);
#22960=ADVANCED_FACE('',(#3221),#1186,.T.);
#22961=ADVANCED_FACE('',(#3222),#1187,.T.);
#22962=ADVANCED_FACE('',(#3223),#1188,.T.);
#22963=ADVANCED_FACE('',(#3224),#1189,.T.);
#22964=ADVANCED_FACE('',(#3225),#1190,.T.);
#22965=ADVANCED_FACE('',(#3226),#1191,.T.);
#22966=ADVANCED_FACE('',(#3227),#1192,.T.);
#22967=ADVANCED_FACE('',(#3228),#1193,.T.);
#22968=ADVANCED_FACE('',(#3229),#1194,.T.);
#22969=ADVANCED_FACE('',(#3230),#1195,.T.);
#22970=ADVANCED_FACE('',(#3231),#1196,.T.);
#22971=ADVANCED_FACE('',(#3232),#1197,.T.);
#22972=ADVANCED_FACE('',(#3233),#1198,.T.);
#22973=ADVANCED_FACE('',(#3234),#1199,.T.);
#22974=ADVANCED_FACE('',(#3235),#1200,.T.);
#22975=ADVANCED_FACE('',(#3236),#1201,.T.);
#22976=ADVANCED_FACE('',(#3237),#1202,.T.);
#22977=ADVANCED_FACE('',(#3238),#1203,.T.);
#22978=ADVANCED_FACE('',(#3239),#1204,.T.);
#22979=ADVANCED_FACE('',(#3240),#1205,.T.);
#22980=ADVANCED_FACE('',(#3241),#1206,.T.);
#22981=ADVANCED_FACE('',(#3242),#1207,.T.);
#22982=ADVANCED_FACE('',(#3243),#1208,.T.);
#22983=ADVANCED_FACE('',(#3244),#1209,.T.);
#22984=ADVANCED_FACE('',(#3245),#1210,.T.);
#22985=ADVANCED_FACE('',(#3246),#1211,.T.);
#22986=ADVANCED_FACE('',(#3247),#1212,.T.);
#22987=ADVANCED_FACE('',(#3248),#1213,.T.);
#22988=ADVANCED_FACE('',(#3249),#1214,.T.);
#22989=ADVANCED_FACE('',(#3250),#1215,.T.);
#22990=ADVANCED_FACE('',(#3251),#1216,.T.);
#22991=ADVANCED_FACE('',(#3252),#1217,.T.);
#22992=ADVANCED_FACE('',(#3253),#1218,.T.);
#22993=ADVANCED_FACE('',(#3254),#1219,.T.);
#22994=ADVANCED_FACE('',(#3255),#1220,.T.);
#22995=ADVANCED_FACE('',(#3256),#1221,.T.);
#22996=ADVANCED_FACE('',(#3257),#1222,.T.);
#22997=ADVANCED_FACE('',(#3258),#1223,.T.);
#22998=ADVANCED_FACE('',(#3259),#1224,.T.);
#22999=ADVANCED_FACE('',(#3260),#1225,.T.);
#23000=ADVANCED_FACE('',(#3261),#1226,.T.);
#23001=ADVANCED_FACE('',(#3262),#1227,.T.);
#23002=ADVANCED_FACE('',(#3263),#1228,.T.);
#23003=ADVANCED_FACE('',(#3264),#1229,.T.);
#23004=ADVANCED_FACE('',(#3265),#1230,.T.);
#23005=ADVANCED_FACE('',(#3266),#1231,.T.);
#23006=ADVANCED_FACE('',(#3267),#1232,.T.);
#23007=ADVANCED_FACE('',(#3268),#1233,.T.);
#23008=ADVANCED_FACE('',(#3269),#1996,.F.);
#23009=ADVANCED_FACE('',(#3270),#369,.F.);
#23010=ADVANCED_FACE('',(#3271),#1997,.T.);
#23011=ADVANCED_FACE('',(#3272),#1234,.T.);
#23012=ADVANCED_FACE('',(#3273),#370,.F.);
#23013=ADVANCED_FACE('',(#3274),#1998,.T.);
#23014=ADVANCED_FACE('',(#3275),#1999,.F.);
#23015=ADVANCED_FACE('',(#3276),#2000,.F.);
#23016=ADVANCED_FACE('',(#3277),#2001,.T.);
#23017=ADVANCED_FACE('',(#3278),#2002,.F.);
#23018=ADVANCED_FACE('',(#3279),#2003,.F.);
#23019=ADVANCED_FACE('',(#3280),#2004,.T.);
#23020=ADVANCED_FACE('',(#3281),#2005,.F.);
#23021=ADVANCED_FACE('',(#3282),#2006,.F.);
#23022=ADVANCED_FACE('',(#3283),#2007,.T.);
#23023=ADVANCED_FACE('',(#3284),#2008,.F.);
#23024=ADVANCED_FACE('',(#3285),#2009,.F.);
#23025=ADVANCED_FACE('',(#3286),#2010,.T.);
#23026=ADVANCED_FACE('',(#3287),#2011,.F.);
#23027=ADVANCED_FACE('',(#3288),#2012,.F.);
#23028=ADVANCED_FACE('',(#3289),#2013,.T.);
#23029=ADVANCED_FACE('',(#3290),#2014,.F.);
#23030=ADVANCED_FACE('',(#3291),#2015,.F.);
#23031=ADVANCED_FACE('',(#3292),#2016,.T.);
#23032=ADVANCED_FACE('',(#3293),#2017,.F.);
#23033=ADVANCED_FACE('',(#3294),#2018,.F.);
#23034=ADVANCED_FACE('',(#3295),#2019,.T.);
#23035=ADVANCED_FACE('',(#3296),#2020,.F.);
#23036=ADVANCED_FACE('',(#3297),#2021,.F.);
#23037=ADVANCED_FACE('',(#3298),#2022,.T.);
#23038=ADVANCED_FACE('',(#3299),#2023,.F.);
#23039=ADVANCED_FACE('',(#3300),#2024,.F.);
#23040=ADVANCED_FACE('',(#3301),#2025,.T.);
#23041=ADVANCED_FACE('',(#3302),#2026,.F.);
#23042=ADVANCED_FACE('',(#3303),#2027,.F.);
#23043=ADVANCED_FACE('',(#3304),#2028,.T.);
#23044=ADVANCED_FACE('',(#3305),#2029,.F.);
#23045=ADVANCED_FACE('',(#3306),#2030,.F.);
#23046=ADVANCED_FACE('',(#3307),#2031,.T.);
#23047=ADVANCED_FACE('',(#3308),#2032,.F.);
#23048=ADVANCED_FACE('',(#3309),#2033,.F.);
#23049=ADVANCED_FACE('',(#3310),#2034,.T.);
#23050=ADVANCED_FACE('',(#3311),#2035,.F.);
#23051=ADVANCED_FACE('',(#3312),#2036,.F.);
#23052=ADVANCED_FACE('',(#3313),#2037,.T.);
#23053=ADVANCED_FACE('',(#3314),#2038,.F.);
#23054=ADVANCED_FACE('',(#3315),#2039,.F.);
#23055=ADVANCED_FACE('',(#3316),#2040,.T.);
#23056=ADVANCED_FACE('',(#3317),#2041,.F.);
#23057=ADVANCED_FACE('',(#3318),#2042,.F.);
#23058=ADVANCED_FACE('',(#3319),#2043,.T.);
#23059=ADVANCED_FACE('',(#3320),#2044,.F.);
#23060=ADVANCED_FACE('',(#3321),#2045,.F.);
#23061=ADVANCED_FACE('',(#3322),#2046,.T.);
#23062=ADVANCED_FACE('',(#3323),#2047,.F.);
#23063=ADVANCED_FACE('',(#3324),#2048,.F.);
#23064=ADVANCED_FACE('',(#3325),#2049,.T.);
#23065=ADVANCED_FACE('',(#3326),#2050,.F.);
#23066=ADVANCED_FACE('',(#3327),#2051,.F.);
#23067=ADVANCED_FACE('',(#3328),#2052,.T.);
#23068=ADVANCED_FACE('',(#3329),#2053,.F.);
#23069=ADVANCED_FACE('',(#3330),#2054,.F.);
#23070=ADVANCED_FACE('',(#3331),#2055,.T.);
#23071=ADVANCED_FACE('',(#3332),#2056,.F.);
#23072=ADVANCED_FACE('',(#3333),#2057,.F.);
#23073=ADVANCED_FACE('',(#3334),#2058,.T.);
#23074=ADVANCED_FACE('',(#3335),#2059,.F.);
#23075=ADVANCED_FACE('',(#3336),#2060,.F.);
#23076=ADVANCED_FACE('',(#3337),#2061,.T.);
#23077=ADVANCED_FACE('',(#3338),#2062,.F.);
#23078=ADVANCED_FACE('',(#3339),#2063,.F.);
#23079=ADVANCED_FACE('',(#3340),#2064,.T.);
#23080=ADVANCED_FACE('',(#3341),#2065,.F.);
#23081=ADVANCED_FACE('',(#3342),#2066,.F.);
#23082=ADVANCED_FACE('',(#3343),#2067,.T.);
#23083=ADVANCED_FACE('',(#3344),#2068,.F.);
#23084=ADVANCED_FACE('',(#3345),#2069,.F.);
#23085=ADVANCED_FACE('',(#3346),#2070,.T.);
#23086=ADVANCED_FACE('',(#3347),#2071,.F.);
#23087=ADVANCED_FACE('',(#3348),#2072,.F.);
#23088=ADVANCED_FACE('',(#3349),#2073,.T.);
#23089=ADVANCED_FACE('',(#3350),#2074,.F.);
#23090=ADVANCED_FACE('',(#3351),#2075,.F.);
#23091=ADVANCED_FACE('',(#3352),#2076,.T.);
#23092=ADVANCED_FACE('',(#3353),#2077,.F.);
#23093=ADVANCED_FACE('',(#3354),#2078,.F.);
#23094=ADVANCED_FACE('',(#3355),#2079,.T.);
#23095=ADVANCED_FACE('',(#3356),#2080,.F.);
#23096=ADVANCED_FACE('',(#3357),#2081,.F.);
#23097=ADVANCED_FACE('',(#3358),#2082,.T.);
#23098=ADVANCED_FACE('',(#3359),#2083,.F.);
#23099=ADVANCED_FACE('',(#3360),#2084,.F.);
#23100=ADVANCED_FACE('',(#3361),#2085,.T.);
#23101=ADVANCED_FACE('',(#3362),#2086,.F.);
#23102=ADVANCED_FACE('',(#3363),#2087,.F.);
#23103=ADVANCED_FACE('',(#3364),#2088,.T.);
#23104=ADVANCED_FACE('',(#3365),#2089,.F.);
#23105=ADVANCED_FACE('',(#3366),#2090,.F.);
#23106=ADVANCED_FACE('',(#3367),#2091,.T.);
#23107=ADVANCED_FACE('',(#3368),#2092,.F.);
#23108=ADVANCED_FACE('',(#3369),#2093,.F.);
#23109=ADVANCED_FACE('',(#3370),#2094,.T.);
#23110=ADVANCED_FACE('',(#3371),#2095,.F.);
#23111=ADVANCED_FACE('',(#3372),#2096,.F.);
#23112=ADVANCED_FACE('',(#3373),#2097,.T.);
#23113=ADVANCED_FACE('',(#3374),#2098,.F.);
#23114=ADVANCED_FACE('',(#3375),#2099,.F.);
#23115=ADVANCED_FACE('',(#3376),#2100,.T.);
#23116=ADVANCED_FACE('',(#3377),#2101,.F.);
#23117=ADVANCED_FACE('',(#3378),#2102,.F.);
#23118=ADVANCED_FACE('',(#3379),#1235,.T.);
#23119=ADVANCED_FACE('',(#3380),#2103,.F.);
#23120=ADVANCED_FACE('',(#3381),#2104,.F.);
#23121=ADVANCED_FACE('',(#3382),#2105,.T.);
#23122=ADVANCED_FACE('',(#3383),#21967,.T.);
#23123=ADVANCED_FACE('',(#3384),#21968,.F.);
#23124=ADVANCED_FACE('',(#3385),#2106,.F.);
#23125=ADVANCED_FACE('',(#3386),#2107,.F.);
#23126=ADVANCED_FACE('',(#3387),#2108,.F.);
#23127=ADVANCED_FACE('',(#3388),#2109,.F.);
#23128=ADVANCED_FACE('',(#3389),#2110,.F.);
#23129=ADVANCED_FACE('',(#3390),#2111,.F.);
#23130=ADVANCED_FACE('',(#3391,#1442),#2112,.F.);
#23131=ADVANCED_FACE('',(#3392),#2113,.T.);
#23132=ADVANCED_FACE('',(#3393),#21969,.T.);
#23133=ADVANCED_FACE('',(#3394),#1236,.T.);
#23134=ADVANCED_FACE('',(#3395),#21970,.T.);
#23135=ADVANCED_FACE('',(#3396,#1443),#2114,.T.);
#23136=ADVANCED_FACE('',(#3397,#1444),#2115,.T.);
#23317=CLOSED_SHELL('',(#22891,#22892,#22893,#22894,#22895,#22896,#22897,
#22898,#22899,#22900,#22901,#22902,#22903,#22904,#22905,#22906,#22907,#22908,
#22909,#22910,#22911,#22912,#22913,#22914,#22915,#22916,#22917,#22918,#22919,
#22920,#22921,#22922,#22923,#22924,#22925,#22926,#22927,#22928,#22929,#22930,
#22931,#22932,#22933,#22934,#22935,#22936,#22937,#22938,#22939,#22940,#22941,
#22942,#22943,#22944,#22945,#22946,#22947,#22948,#22949,#22950,#22951,#22952,
#22953,#22954,#22955,#22956,#22957,#22958,#22959,#22960,#22961,#22962,#22963,
#22964,#22965,#22966,#22967,#22968,#22969,#22970,#22971,#22972,#22973,#22974,
#22975,#22976,#22977,#22978,#22979,#22980,#22981,#22982,#22983,#22984,#22985,
#22986,#22987,#22988,#22989,#22990,#22991,#22992,#22993,#22994,#22995,#22996,
#22997,#22998,#22999,#23000,#23001,#23002,#23003,#23004,#23005,#23006,#23007,
#23008,#23009,#23010,#23011,#23012,#23013,#23014,#23015,#23016,#23017,#23018,
#23019,#23020,#23021,#23022,#23023,#23024,#23025,#23026,#23027,#23028,#23029,
#23030,#23031,#23032,#23033,#23034,#23035,#23036,#23037,#23038,#23039,#23040,
#23041,#23042,#23043,#23044,#23045,#23046,#23047,#23048,#23049,#23050,#23051,
#23052,#23053,#23054,#23055,#23056,#23057,#23058,#23059,#23060,#23061,#23062,
#23063,#23064,#23065,#23066,#23067,#23068,#23069,#23070,#23071,#23072,#23073,
#23074,#23075,#23076,#23077,#23078,#23079,#23080,#23081,#23082,#23083,#23084,
#23085,#23086,#23087,#23088,#23089,#23090,#23091,#23092,#23093,#23094,#23095,
#23096,#23097,#23098,#23099,#23100,#23101,#23102,#23103,#23104,#23105,#23106,
#23107,#23108,#23109,#23110,#23111,#23112,#23113,#23114,#23115,#23116,#23117,
#23118,#23119,#23120,#23121,#23122,#23123,#23124,#23125,#23126,#23127,#23128,
#23129,#23130,#23131,#23132,#23133,#23134,#23135,#23136));
#25038=AXIS2_PLACEMENT_3D('',#41661,#30021,#30022);
#25039=AXIS2_PLACEMENT_3D('',#41662,#30023,#30024);
#25040=AXIS2_PLACEMENT_3D('',#41684,#30026,#30027);
#25041=AXIS2_PLACEMENT_3D('',#41687,#30029,#30030);
#25042=AXIS2_PLACEMENT_3D('',#41689,#30031,#30032);
#25043=AXIS2_PLACEMENT_3D('',#41703,#30033,#30034);
#25044=AXIS2_PLACEMENT_3D('',#41751,#30036,#30037);
#25045=AXIS2_PLACEMENT_3D('',#41805,#30039,#30040);
#25046=AXIS2_PLACEMENT_3D('',#41853,#30042,#30043);
#25047=AXIS2_PLACEMENT_3D('',#41901,#30045,#30046);
#25048=AXIS2_PLACEMENT_3D('',#41955,#30048,#30049);
#25049=AXIS2_PLACEMENT_3D('',#42003,#30051,#30052);
#25050=AXIS2_PLACEMENT_3D('',#42051,#30054,#30055);
#25051=AXIS2_PLACEMENT_3D('',#42099,#30057,#30058);
#25052=AXIS2_PLACEMENT_3D('',#42153,#30060,#30061);
#25053=AXIS2_PLACEMENT_3D('',#42201,#30063,#30064);
#25054=AXIS2_PLACEMENT_3D('',#42249,#30066,#30067);
#25055=AXIS2_PLACEMENT_3D('',#42303,#30069,#30070);
#25056=AXIS2_PLACEMENT_3D('',#42351,#30072,#30073);
#25057=AXIS2_PLACEMENT_3D('',#42399,#30075,#30076);
#25058=AXIS2_PLACEMENT_3D('',#42450,#30078,#30079);
#25059=AXIS2_PLACEMENT_3D('',#42501,#30081,#30082);
#25060=AXIS2_PLACEMENT_3D('',#42549,#30084,#30085);
#25061=AXIS2_PLACEMENT_3D('',#42597,#30087,#30088);
#25062=AXIS2_PLACEMENT_3D('',#42651,#30090,#30091);
#25063=AXIS2_PLACEMENT_3D('',#42699,#30093,#30094);
#25064=AXIS2_PLACEMENT_3D('',#42747,#30096,#30097);
#25065=AXIS2_PLACEMENT_3D('',#42801,#30099,#30100);
#25066=AXIS2_PLACEMENT_3D('',#42849,#30102,#30103);
#25067=AXIS2_PLACEMENT_3D('',#42897,#30105,#30106);
#25068=AXIS2_PLACEMENT_3D('',#42945,#30108,#30109);
#25069=AXIS2_PLACEMENT_3D('',#42999,#30111,#30112);
#25070=AXIS2_PLACEMENT_3D('',#43047,#30114,#30115);
#25071=AXIS2_PLACEMENT_3D('',#43095,#30117,#30118);
#25072=AXIS2_PLACEMENT_3D('',#43149,#30120,#30121);
#25073=AXIS2_PLACEMENT_3D('',#43197,#30123,#30124);
#25074=AXIS2_PLACEMENT_3D('',#43245,#30126,#30127);
#25075=AXIS2_PLACEMENT_3D('',#43293,#30129,#30130);
#25076=AXIS2_PLACEMENT_3D('',#43347,#30132,#30133);
#25077=AXIS2_PLACEMENT_3D('',#43395,#30135,#30136);
#25078=AXIS2_PLACEMENT_3D('',#43443,#30138,#30139);
#25079=AXIS2_PLACEMENT_3D('',#43497,#30141,#30142);
#25080=AXIS2_PLACEMENT_3D('',#43545,#30144,#30145);
#25081=AXIS2_PLACEMENT_3D('',#43593,#30147,#30148);
#25082=AXIS2_PLACEMENT_3D('',#43644,#30150,#30151);
#25083=AXIS2_PLACEMENT_3D('',#43695,#30153,#30154);
#25084=AXIS2_PLACEMENT_3D('',#43743,#30156,#30157);
#25085=AXIS2_PLACEMENT_3D('',#43791,#30159,#30160);
#25086=AXIS2_PLACEMENT_3D('',#43845,#30162,#30163);
#25087=AXIS2_PLACEMENT_3D('',#43893,#30165,#30166);
#25088=AXIS2_PLACEMENT_3D('',#43941,#30168,#30169);
#25089=AXIS2_PLACEMENT_3D('',#43995,#30171,#30172);
#25090=AXIS2_PLACEMENT_3D('',#44043,#30174,#30175);
#25091=AXIS2_PLACEMENT_3D('',#44091,#30177,#30178);
#25092=AXIS2_PLACEMENT_3D('',#44139,#30180,#30181);
#25093=AXIS2_PLACEMENT_3D('',#44193,#30183,#30184);
#25094=AXIS2_PLACEMENT_3D('',#44241,#30186,#30187);
#25095=AXIS2_PLACEMENT_3D('',#44289,#30189,#30190);
#25096=AXIS2_PLACEMENT_3D('',#44343,#30192,#30193);
#25097=AXIS2_PLACEMENT_3D('',#44391,#30195,#30196);
#25098=AXIS2_PLACEMENT_3D('',#44439,#30198,#30199);
#25099=AXIS2_PLACEMENT_3D('',#44487,#30201,#30202);
#25100=AXIS2_PLACEMENT_3D('',#44541,#30204,#30205);
#25101=AXIS2_PLACEMENT_3D('',#44553,#30207,#30208);
#25102=AXIS2_PLACEMENT_3D('',#44559,#30209,#30210);
#25103=AXIS2_PLACEMENT_3D('',#44584,#30212,#30213);
#25104=AXIS2_PLACEMENT_3D('',#44609,#30215,#30216);
#25105=AXIS2_PLACEMENT_3D('',#44633,#30218,#30219);
#25106=AXIS2_PLACEMENT_3D('',#44657,#30221,#30222);
#25107=AXIS2_PLACEMENT_3D('',#44682,#30224,#30225);
#25108=AXIS2_PLACEMENT_3D('',#44707,#30227,#30228);
#25109=AXIS2_PLACEMENT_3D('',#44731,#30230,#30231);
#25110=AXIS2_PLACEMENT_3D('',#44756,#30233,#30234);
#25111=AXIS2_PLACEMENT_3D('',#44781,#30236,#30237);
#25112=AXIS2_PLACEMENT_3D('',#44805,#30239,#30240);
#25113=AXIS2_PLACEMENT_3D('',#44829,#30242,#30243);
#25114=AXIS2_PLACEMENT_3D('',#44854,#30245,#30246);
#25115=AXIS2_PLACEMENT_3D('',#44879,#30248,#30249);
#25116=AXIS2_PLACEMENT_3D('',#44903,#30251,#30252);
#25117=AXIS2_PLACEMENT_3D('',#44928,#30254,#30255);
#25118=AXIS2_PLACEMENT_3D('',#44953,#30257,#30258);
#25119=AXIS2_PLACEMENT_3D('',#44977,#30260,#30261);
#25120=AXIS2_PLACEMENT_3D('',#45002,#30263,#30264);
#25121=AXIS2_PLACEMENT_3D('',#45026,#30266,#30267);
#25122=AXIS2_PLACEMENT_3D('',#45051,#30269,#30270);
#25123=AXIS2_PLACEMENT_3D('',#45075,#30272,#30273);
#25124=AXIS2_PLACEMENT_3D('',#45100,#30275,#30276);
#25125=AXIS2_PLACEMENT_3D('',#45125,#30278,#30279);
#25126=AXIS2_PLACEMENT_3D('',#45149,#30281,#30282);
#25127=AXIS2_PLACEMENT_3D('',#45174,#30284,#30285);
#25128=AXIS2_PLACEMENT_3D('',#45199,#30287,#30288);
#25129=AXIS2_PLACEMENT_3D('',#45223,#30290,#30291);
#25130=AXIS2_PLACEMENT_3D('',#45247,#30293,#30294);
#25131=AXIS2_PLACEMENT_3D('',#45272,#30296,#30297);
#25132=AXIS2_PLACEMENT_3D('',#45297,#30299,#30300);
#25133=AXIS2_PLACEMENT_3D('',#45321,#30302,#30303);
#25134=AXIS2_PLACEMENT_3D('',#45346,#30305,#30306);
#25135=AXIS2_PLACEMENT_3D('',#45371,#30308,#30309);
#25136=AXIS2_PLACEMENT_3D('',#45395,#30311,#30312);
#25137=AXIS2_PLACEMENT_3D('',#45419,#30314,#30315);
#25138=AXIS2_PLACEMENT_3D('',#45444,#30317,#30318);
#25139=AXIS2_PLACEMENT_3D('',#45469,#30320,#30321);
#25140=AXIS2_PLACEMENT_3D('',#45493,#30323,#30324);
#25141=AXIS2_PLACEMENT_3D('',#45518,#30326,#30327);
#25142=AXIS2_PLACEMENT_3D('',#45543,#30329,#30330);
#25143=AXIS2_PLACEMENT_3D('',#45567,#30332,#30333);
#25144=AXIS2_PLACEMENT_3D('',#45592,#30335,#30336);
#25145=AXIS2_PLACEMENT_3D('',#45616,#30338,#30339);
#25146=AXIS2_PLACEMENT_3D('',#45641,#30341,#30342);
#25147=AXIS2_PLACEMENT_3D('',#45665,#30344,#30345);
#25148=AXIS2_PLACEMENT_3D('',#45690,#30347,#30348);
#25149=AXIS2_PLACEMENT_3D('',#45715,#30350,#30351);
#25150=AXIS2_PLACEMENT_3D('',#45739,#30353,#30354);
#25151=AXIS2_PLACEMENT_3D('',#45764,#30356,#30357);
#25152=AXIS2_PLACEMENT_3D('',#45789,#30359,#30360);
#25153=AXIS2_PLACEMENT_3D('',#45813,#30362,#30363);
#25154=AXIS2_PLACEMENT_3D('',#45837,#30365,#30366);
#25155=AXIS2_PLACEMENT_3D('',#45862,#30368,#30369);
#25156=AXIS2_PLACEMENT_3D('',#45887,#30371,#30372);
#25157=AXIS2_PLACEMENT_3D('',#45911,#30374,#30375);
#25158=AXIS2_PLACEMENT_3D('',#45936,#30377,#30378);
#25159=AXIS2_PLACEMENT_3D('',#45961,#30380,#30381);
#25160=AXIS2_PLACEMENT_3D('',#45985,#30383,#30384);
#25161=AXIS2_PLACEMENT_3D('',#46040,#30385,#30386);
#25162=AXIS2_PLACEMENT_3D('',#46042,#30387,#30388);
#25163=AXIS2_PLACEMENT_3D('',#47664,#30389,#30390);
#25164=AXIS2_PLACEMENT_3D('',#47718,#30391,#30392);
#25165=AXIS2_PLACEMENT_3D('',#47719,#30393,#30394);
#25166=AXIS2_PLACEMENT_3D('',#49232,#30395,#30396);
#25167=AXIS2_PLACEMENT_3D('',#49235,#30397,#30398);
#25168=AXIS2_PLACEMENT_3D('',#49239,#30401,#30402);
#25169=AXIS2_PLACEMENT_3D('',#49247,#30405,#30406);
#25170=AXIS2_PLACEMENT_3D('',#49253,#30408,#30409);
#25171=AXIS2_PLACEMENT_3D('',#49256,#30410,#30411);
#25172=AXIS2_PLACEMENT_3D('',#49260,#30414,#30415);
#25173=AXIS2_PLACEMENT_3D('',#49268,#30418,#30419);
#25174=AXIS2_PLACEMENT_3D('',#49274,#30421,#30422);
#25175=AXIS2_PLACEMENT_3D('',#49277,#30423,#30424);
#25176=AXIS2_PLACEMENT_3D('',#49281,#30427,#30428);
#25177=AXIS2_PLACEMENT_3D('',#49289,#30431,#30432);
#25178=AXIS2_PLACEMENT_3D('',#49295,#30434,#30435);
#25179=AXIS2_PLACEMENT_3D('',#49298,#30436,#30437);
#25180=AXIS2_PLACEMENT_3D('',#49302,#30440,#30441);
#25181=AXIS2_PLACEMENT_3D('',#49310,#30444,#30445);
#25182=AXIS2_PLACEMENT_3D('',#49316,#30447,#30448);
#25183=AXIS2_PLACEMENT_3D('',#49319,#30449,#30450);
#25184=AXIS2_PLACEMENT_3D('',#49323,#30453,#30454);
#25185=AXIS2_PLACEMENT_3D('',#49331,#30457,#30458);
#25186=AXIS2_PLACEMENT_3D('',#49337,#30460,#30461);
#25187=AXIS2_PLACEMENT_3D('',#49340,#30462,#30463);
#25188=AXIS2_PLACEMENT_3D('',#49344,#30466,#30467);
#25189=AXIS2_PLACEMENT_3D('',#49352,#30470,#30471);
#25190=AXIS2_PLACEMENT_3D('',#49358,#30473,#30474);
#25191=AXIS2_PLACEMENT_3D('',#49361,#30475,#30476);
#25192=AXIS2_PLACEMENT_3D('',#49365,#30479,#30480);
#25193=AXIS2_PLACEMENT_3D('',#49373,#30483,#30484);
#25194=AXIS2_PLACEMENT_3D('',#49379,#30486,#30487);
#25195=AXIS2_PLACEMENT_3D('',#49382,#30488,#30489);
#25196=AXIS2_PLACEMENT_3D('',#49386,#30492,#30493);
#25197=AXIS2_PLACEMENT_3D('',#49394,#30496,#30497);
#25198=AXIS2_PLACEMENT_3D('',#49400,#30499,#30500);
#25199=AXIS2_PLACEMENT_3D('',#49403,#30501,#30502);
#25200=AXIS2_PLACEMENT_3D('',#49407,#30505,#30506);
#25201=AXIS2_PLACEMENT_3D('',#49415,#30509,#30510);
#25202=AXIS2_PLACEMENT_3D('',#49421,#30512,#30513);
#25203=AXIS2_PLACEMENT_3D('',#49424,#30514,#30515);
#25204=AXIS2_PLACEMENT_3D('',#49428,#30518,#30519);
#25205=AXIS2_PLACEMENT_3D('',#49436,#30522,#30523);
#25206=AXIS2_PLACEMENT_3D('',#49442,#30525,#30526);
#25207=AXIS2_PLACEMENT_3D('',#49445,#30527,#30528);
#25208=AXIS2_PLACEMENT_3D('',#49449,#30531,#30532);
#25209=AXIS2_PLACEMENT_3D('',#49457,#30535,#30536);
#25210=AXIS2_PLACEMENT_3D('',#49463,#30538,#30539);
#25211=AXIS2_PLACEMENT_3D('',#49466,#30540,#30541);
#25212=AXIS2_PLACEMENT_3D('',#49470,#30544,#30545);
#25213=AXIS2_PLACEMENT_3D('',#49478,#30548,#30549);
#25214=AXIS2_PLACEMENT_3D('',#49484,#30551,#30552);
#25215=AXIS2_PLACEMENT_3D('',#49487,#30553,#30554);
#25216=AXIS2_PLACEMENT_3D('',#49491,#30557,#30558);
#25217=AXIS2_PLACEMENT_3D('',#49499,#30561,#30562);
#25218=AXIS2_PLACEMENT_3D('',#49505,#30564,#30565);
#25219=AXIS2_PLACEMENT_3D('',#49508,#30566,#30567);
#25220=AXIS2_PLACEMENT_3D('',#49512,#30570,#30571);
#25221=AXIS2_PLACEMENT_3D('',#49520,#30574,#30575);
#25222=AXIS2_PLACEMENT_3D('',#49526,#30577,#30578);
#25223=AXIS2_PLACEMENT_3D('',#49529,#30579,#30580);
#25224=AXIS2_PLACEMENT_3D('',#49533,#30583,#30584);
#25225=AXIS2_PLACEMENT_3D('',#49541,#30587,#30588);
#25226=AXIS2_PLACEMENT_3D('',#49547,#30590,#30591);
#25227=AXIS2_PLACEMENT_3D('',#49550,#30592,#30593);
#25228=AXIS2_PLACEMENT_3D('',#49554,#30596,#30597);
#25229=AXIS2_PLACEMENT_3D('',#49562,#30600,#30601);
#25230=AXIS2_PLACEMENT_3D('',#49568,#30603,#30604);
#25231=AXIS2_PLACEMENT_3D('',#49571,#30605,#30606);
#25232=AXIS2_PLACEMENT_3D('',#49575,#30609,#30610);
#25233=AXIS2_PLACEMENT_3D('',#49583,#30613,#30614);
#25234=AXIS2_PLACEMENT_3D('',#49589,#30616,#30617);
#25235=AXIS2_PLACEMENT_3D('',#49592,#30618,#30619);
#25236=AXIS2_PLACEMENT_3D('',#49597,#30622,#30623);
#25237=AXIS2_PLACEMENT_3D('',#49598,#30624,#30625);
#25238=AXIS2_PLACEMENT_3D('',#49606,#30628,#30629);
#25239=AXIS2_PLACEMENT_3D('',#49612,#30631,#30632);
#25240=AXIS2_PLACEMENT_3D('',#49615,#30633,#30634);
#25241=AXIS2_PLACEMENT_3D('',#49619,#30637,#30638);
#25242=AXIS2_PLACEMENT_3D('',#49627,#30641,#30642);
#25243=AXIS2_PLACEMENT_3D('',#49633,#30644,#30645);
#25244=AXIS2_PLACEMENT_3D('',#49636,#30646,#30647);
#25245=AXIS2_PLACEMENT_3D('',#49640,#30650,#30651);
#25246=AXIS2_PLACEMENT_3D('',#49648,#30654,#30655);
#25247=AXIS2_PLACEMENT_3D('',#49654,#30657,#30658);
#25248=AXIS2_PLACEMENT_3D('',#49657,#30659,#30660);
#25249=AXIS2_PLACEMENT_3D('',#49661,#30663,#30664);
#25250=AXIS2_PLACEMENT_3D('',#49669,#30667,#30668);
#25251=AXIS2_PLACEMENT_3D('',#49675,#30670,#30671);
#25252=AXIS2_PLACEMENT_3D('',#49678,#30672,#30673);
#25253=AXIS2_PLACEMENT_3D('',#49682,#30676,#30677);
#25254=AXIS2_PLACEMENT_3D('',#49690,#30680,#30681);
#25255=AXIS2_PLACEMENT_3D('',#49696,#30683,#30684);
#25256=AXIS2_PLACEMENT_3D('',#49699,#30685,#30686);
#25257=AXIS2_PLACEMENT_3D('',#49703,#30689,#30690);
#25258=AXIS2_PLACEMENT_3D('',#49711,#30693,#30694);
#25259=AXIS2_PLACEMENT_3D('',#49717,#30696,#30697);
#25260=AXIS2_PLACEMENT_3D('',#49720,#30698,#30699);
#25261=AXIS2_PLACEMENT_3D('',#49724,#30702,#30703);
#25262=AXIS2_PLACEMENT_3D('',#49732,#30706,#30707);
#25263=AXIS2_PLACEMENT_3D('',#49738,#30709,#30710);
#25264=AXIS2_PLACEMENT_3D('',#49741,#30711,#30712);
#25265=AXIS2_PLACEMENT_3D('',#49745,#30715,#30716);
#25266=AXIS2_PLACEMENT_3D('',#49753,#30719,#30720);
#25267=AXIS2_PLACEMENT_3D('',#49759,#30722,#30723);
#25268=AXIS2_PLACEMENT_3D('',#49762,#30724,#30725);
#25269=AXIS2_PLACEMENT_3D('',#49766,#30728,#30729);
#25270=AXIS2_PLACEMENT_3D('',#49774,#30732,#30733);
#25271=AXIS2_PLACEMENT_3D('',#49780,#30735,#30736);
#25272=AXIS2_PLACEMENT_3D('',#49783,#30737,#30738);
#25273=AXIS2_PLACEMENT_3D('',#49787,#30741,#30742);
#25274=AXIS2_PLACEMENT_3D('',#49795,#30745,#30746);
#25275=AXIS2_PLACEMENT_3D('',#49801,#30748,#30749);
#25276=AXIS2_PLACEMENT_3D('',#49804,#30750,#30751);
#25277=AXIS2_PLACEMENT_3D('',#49808,#30754,#30755);
#25278=AXIS2_PLACEMENT_3D('',#49816,#30758,#30759);
#25279=AXIS2_PLACEMENT_3D('',#49822,#30761,#30762);
#25280=AXIS2_PLACEMENT_3D('',#49825,#30763,#30764);
#25281=AXIS2_PLACEMENT_3D('',#49829,#30767,#30768);
#25282=AXIS2_PLACEMENT_3D('',#49837,#30771,#30772);
#25283=AXIS2_PLACEMENT_3D('',#49843,#30774,#30775);
#25284=AXIS2_PLACEMENT_3D('',#49846,#30776,#30777);
#25285=AXIS2_PLACEMENT_3D('',#49850,#30780,#30781);
#25286=AXIS2_PLACEMENT_3D('',#49858,#30784,#30785);
#25287=AXIS2_PLACEMENT_3D('',#49864,#30787,#30788);
#25288=AXIS2_PLACEMENT_3D('',#49867,#30789,#30790);
#25289=AXIS2_PLACEMENT_3D('',#49871,#30793,#30794);
#25290=AXIS2_PLACEMENT_3D('',#49879,#30797,#30798);
#25291=AXIS2_PLACEMENT_3D('',#49885,#30800,#30801);
#25292=AXIS2_PLACEMENT_3D('',#49888,#30802,#30803);
#25293=AXIS2_PLACEMENT_3D('',#49892,#30806,#30807);
#25294=AXIS2_PLACEMENT_3D('',#49900,#30810,#30811);
#25295=AXIS2_PLACEMENT_3D('',#49906,#30813,#30814);
#25296=AXIS2_PLACEMENT_3D('',#49909,#30815,#30816);
#25297=AXIS2_PLACEMENT_3D('',#49913,#30819,#30820);
#25298=AXIS2_PLACEMENT_3D('',#49921,#30823,#30824);
#25299=AXIS2_PLACEMENT_3D('',#49927,#30826,#30827);
#25300=AXIS2_PLACEMENT_3D('',#49930,#30828,#30829);
#25301=AXIS2_PLACEMENT_3D('',#49934,#30832,#30833);
#25302=AXIS2_PLACEMENT_3D('',#49942,#30836,#30837);
#25303=AXIS2_PLACEMENT_3D('',#49948,#30839,#30840);
#25304=AXIS2_PLACEMENT_3D('',#49951,#30841,#30842);
#25305=AXIS2_PLACEMENT_3D('',#49955,#30845,#30846);
#25306=AXIS2_PLACEMENT_3D('',#49963,#30849,#30850);
#25307=AXIS2_PLACEMENT_3D('',#49969,#30852,#30853);
#25308=AXIS2_PLACEMENT_3D('',#49970,#30854,#30855);
#25309=AXIS2_PLACEMENT_3D('',#49971,#30856,#30857);
#25310=AXIS2_PLACEMENT_3D('',#49972,#30858,#30859);
#25311=AXIS2_PLACEMENT_3D('',#49973,#30860,#30861);
#25312=AXIS2_PLACEMENT_3D('',#49974,#30862,#30863);
#25313=AXIS2_PLACEMENT_3D('',#49975,#30864,#30865);
#25314=AXIS2_PLACEMENT_3D('',#49976,#30866,#30867);
#25315=AXIS2_PLACEMENT_3D('',#49977,#30868,#30869);
#25316=AXIS2_PLACEMENT_3D('',#49978,#30870,#30871);
#25317=AXIS2_PLACEMENT_3D('',#49979,#30872,#30873);
#25318=AXIS2_PLACEMENT_3D('',#49980,#30874,#30875);
#25319=AXIS2_PLACEMENT_3D('',#49981,#30876,#30877);
#25320=AXIS2_PLACEMENT_3D('',#49982,#30878,#30879);
#25321=AXIS2_PLACEMENT_3D('',#49983,#30880,#30881);
#25322=AXIS2_PLACEMENT_3D('',#49984,#30882,#30883);
#25323=AXIS2_PLACEMENT_3D('',#49985,#30884,#30885);
#25324=AXIS2_PLACEMENT_3D('',#49986,#30886,#30887);
#25325=AXIS2_PLACEMENT_3D('',#49989,#30889,#30890);
#25326=AXIS2_PLACEMENT_3D('',#49990,#30891,#30892);
#25327=AXIS2_PLACEMENT_3D('',#49991,#30893,#30894);
#25328=AXIS2_PLACEMENT_3D('',#49992,#30895,#30896);
#25329=AXIS2_PLACEMENT_3D('',#49993,#30897,#30898);
#25330=AXIS2_PLACEMENT_3D('',#49994,#30899,#30900);
#25331=AXIS2_PLACEMENT_3D('',#49995,#30901,#30902);
#25332=AXIS2_PLACEMENT_3D('',#49996,#30903,#30904);
#25333=AXIS2_PLACEMENT_3D('',#49997,#30905,#30906);
#25334=AXIS2_PLACEMENT_3D('',#49998,#30907,#30908);
#25335=AXIS2_PLACEMENT_3D('',#49999,#30909,#30910);
#25336=AXIS2_PLACEMENT_3D('',#50000,#30911,#30912);
#25337=AXIS2_PLACEMENT_3D('',#50001,#30913,#30914);
#25338=AXIS2_PLACEMENT_3D('',#50002,#30915,#30916);
#25339=AXIS2_PLACEMENT_3D('',#50003,#30917,#30918);
#25340=AXIS2_PLACEMENT_3D('',#50004,#30919,#30920);
#25341=AXIS2_PLACEMENT_3D('',#50005,#30921,#30922);
#25342=AXIS2_PLACEMENT_3D('',#50006,#30923,#30924);
#25343=AXIS2_PLACEMENT_3D('',#50008,#30925,#30926);
#25344=AXIS2_PLACEMENT_3D('',#50012,#30928,#30929);
#25345=AXIS2_PLACEMENT_3D('',#50015,#30931,#30932);
#25346=AXIS2_PLACEMENT_3D('',#50016,#30933,#30934);
#25347=AXIS2_PLACEMENT_3D('',#50024,#30937,#30938);
#25348=AXIS2_PLACEMENT_3D('',#50029,#30940,#30941);
#25349=AXIS2_PLACEMENT_3D('',#50030,#30942,#30943);
#25350=AXIS2_PLACEMENT_3D('',#50032,#30944,#30945);
#25351=AXIS2_PLACEMENT_3D('',#50034,#30947,#30948);
#25352=AXIS2_PLACEMENT_3D('',#50038,#30950,#30951);
#25353=AXIS2_PLACEMENT_3D('',#50039,#30952,#30953);
#25354=AXIS2_PLACEMENT_3D('',#50048,#30958,#30959);
#25355=AXIS2_PLACEMENT_3D('',#50054,#30963,#30964);
#25356=AXIS2_PLACEMENT_3D('',#50060,#30968,#30969);
#25357=AXIS2_PLACEMENT_3D('',#50066,#30973,#30974);
#25358=AXIS2_PLACEMENT_3D('',#50072,#30978,#30979);
#25359=AXIS2_PLACEMENT_3D('',#50075,#30982,#30983);
#25360=AXIS2_PLACEMENT_3D('',#50076,#30984,#30985);
#25361=AXIS2_PLACEMENT_3D('',#50078,#30986,#30987);
#25362=AXIS2_PLACEMENT_3D('',#50079,#30988,#30989);
#25363=AXIS2_PLACEMENT_3D('',#50081,#30991,#30992);
#25364=AXIS2_PLACEMENT_3D('',#50082,#30993,#30994);
#25365=AXIS2_PLACEMENT_3D('',#50083,#30995,#30996);
#25366=AXIS2_PLACEMENT_3D('',#50085,#30997,#30998);
#25367=AXIS2_PLACEMENT_3D('',#50087,#31000,#31001);
#25368=AXIS2_PLACEMENT_3D('',#50088,#31002,#31003);
#30021=DIRECTION('axis',(0.,0.,1.));
#30022=DIRECTION('refdir',(1.,0.,0.));
#30023=DIRECTION('center_axis',(0.,0.,1.));
#30024=DIRECTION('ref_axis',(1.,0.,0.));
#30025=DIRECTION('',(0.,0.,-1.));
#30026=DIRECTION('center_axis',(0.,0.,-1.));
#30027=DIRECTION('ref_axis',(1.,0.,0.));
#30028=DIRECTION('',(0.,0.,-1.));
#30029=DIRECTION('center_axis',(0.,0.,1.));
#30030=DIRECTION('ref_axis',(1.,0.,0.));
#30031=DIRECTION('center_axis',(0.,0.,-1.));
#30032=DIRECTION('ref_axis',(1.,0.,0.));
#30033=DIRECTION('center_axis',(0.,0.,1.));
#30034=DIRECTION('ref_axis',(1.,0.,0.));
#30035=DIRECTION('',(0.,0.,-1.));
#30036=DIRECTION('center_axis',(0.,0.,1.));
#30037=DIRECTION('ref_axis',(1.,0.,0.));
#30038=DIRECTION('',(0.,0.,-1.));
#30039=DIRECTION('center_axis',(0.,0.,1.));
#30040=DIRECTION('ref_axis',(1.,0.,0.));
#30041=DIRECTION('',(0.,0.,-1.));
#30042=DIRECTION('center_axis',(0.,0.,1.));
#30043=DIRECTION('ref_axis',(1.,0.,0.));
#30044=DIRECTION('',(0.,0.,-1.));
#30045=DIRECTION('center_axis',(0.,0.,1.));
#30046=DIRECTION('ref_axis',(1.,0.,0.));
#30047=DIRECTION('',(0.,0.,-1.));
#30048=DIRECTION('center_axis',(0.,0.,1.));
#30049=DIRECTION('ref_axis',(1.,0.,0.));
#30050=DIRECTION('',(0.,0.,-1.));
#30051=DIRECTION('center_axis',(0.,0.,1.));
#30052=DIRECTION('ref_axis',(1.,0.,0.));
#30053=DIRECTION('',(0.,0.,-1.));
#30054=DIRECTION('center_axis',(0.,0.,1.));
#30055=DIRECTION('ref_axis',(1.,0.,0.));
#30056=DIRECTION('',(0.,0.,-1.));
#30057=DIRECTION('center_axis',(0.,0.,1.));
#30058=DIRECTION('ref_axis',(1.,0.,0.));
#30059=DIRECTION('',(0.,0.,-1.));
#30060=DIRECTION('center_axis',(0.,0.,1.));
#30061=DIRECTION('ref_axis',(1.,0.,0.));
#30062=DIRECTION('',(0.,0.,-1.));
#30063=DIRECTION('center_axis',(0.,0.,1.));
#30064=DIRECTION('ref_axis',(1.,0.,0.));
#30065=DIRECTION('',(0.,0.,-1.));
#30066=DIRECTION('center_axis',(0.,0.,1.));
#30067=DIRECTION('ref_axis',(1.,0.,0.));
#30068=DIRECTION('',(0.,0.,-1.));
#30069=DIRECTION('center_axis',(0.,0.,1.));
#30070=DIRECTION('ref_axis',(1.,0.,0.));
#30071=DIRECTION('',(0.,0.,-1.));
#30072=DIRECTION('center_axis',(0.,0.,1.));
#30073=DIRECTION('ref_axis',(1.,0.,0.));
#30074=DIRECTION('',(0.,0.,-1.));
#30075=DIRECTION('center_axis',(0.,0.,1.));
#30076=DIRECTION('ref_axis',(1.,0.,0.));
#30077=DIRECTION('',(0.,0.,-1.));
#30078=DIRECTION('center_axis',(0.,0.,1.));
#30079=DIRECTION('ref_axis',(1.,0.,0.));
#30080=DIRECTION('',(0.,0.,-1.));
#30081=DIRECTION('center_axis',(0.,0.,1.));
#30082=DIRECTION('ref_axis',(1.,0.,0.));
#30083=DIRECTION('',(0.,0.,-1.));
#30084=DIRECTION('center_axis',(0.,0.,1.));
#30085=DIRECTION('ref_axis',(1.,0.,0.));
#30086=DIRECTION('',(0.,0.,-1.));
#30087=DIRECTION('center_axis',(0.,0.,1.));
#30088=DIRECTION('ref_axis',(1.,0.,0.));
#30089=DIRECTION('',(0.,0.,-1.));
#30090=DIRECTION('center_axis',(0.,0.,1.));
#30091=DIRECTION('ref_axis',(1.,0.,0.));
#30092=DIRECTION('',(0.,0.,-1.));
#30093=DIRECTION('center_axis',(0.,0.,1.));
#30094=DIRECTION('ref_axis',(1.,0.,0.));
#30095=DIRECTION('',(0.,0.,-1.));
#30096=DIRECTION('center_axis',(0.,0.,1.));
#30097=DIRECTION('ref_axis',(1.,0.,0.));
#30098=DIRECTION('',(0.,0.,-1.));
#30099=DIRECTION('center_axis',(0.,0.,1.));
#30100=DIRECTION('ref_axis',(1.,0.,0.));
#30101=DIRECTION('',(0.,0.,-1.));
#30102=DIRECTION('center_axis',(0.,0.,1.));
#30103=DIRECTION('ref_axis',(1.,0.,0.));
#30104=DIRECTION('',(0.,0.,-1.));
#30105=DIRECTION('center_axis',(0.,0.,1.));
#30106=DIRECTION('ref_axis',(1.,0.,0.));
#30107=DIRECTION('',(0.,0.,-1.));
#30108=DIRECTION('center_axis',(0.,0.,1.));
#30109=DIRECTION('ref_axis',(1.,0.,0.));
#30110=DIRECTION('',(0.,0.,-1.));
#30111=DIRECTION('center_axis',(0.,0.,1.));
#30112=DIRECTION('ref_axis',(1.,0.,0.));
#30113=DIRECTION('',(0.,0.,-1.));
#30114=DIRECTION('center_axis',(0.,0.,1.));
#30115=DIRECTION('ref_axis',(1.,0.,0.));
#30116=DIRECTION('',(0.,0.,-1.));
#30117=DIRECTION('center_axis',(0.,0.,1.));
#30118=DIRECTION('ref_axis',(1.,0.,0.));
#30119=DIRECTION('',(0.,0.,-1.));
#30120=DIRECTION('center_axis',(0.,0.,1.));
#30121=DIRECTION('ref_axis',(1.,0.,0.));
#30122=DIRECTION('',(0.,0.,-1.));
#30123=DIRECTION('center_axis',(0.,0.,1.));
#30124=DIRECTION('ref_axis',(1.,0.,0.));
#30125=DIRECTION('',(0.,0.,-1.));
#30126=DIRECTION('center_axis',(0.,0.,1.));
#30127=DIRECTION('ref_axis',(1.,0.,0.));
#30128=DIRECTION('',(0.,0.,-1.));
#30129=DIRECTION('center_axis',(0.,0.,1.));
#30130=DIRECTION('ref_axis',(1.,0.,0.));
#30131=DIRECTION('',(0.,0.,-1.));
#30132=DIRECTION('center_axis',(0.,0.,1.));
#30133=DIRECTION('ref_axis',(1.,0.,0.));
#30134=DIRECTION('',(0.,0.,-1.));
#30135=DIRECTION('center_axis',(0.,0.,1.));
#30136=DIRECTION('ref_axis',(1.,0.,0.));
#30137=DIRECTION('',(0.,0.,-1.));
#30138=DIRECTION('center_axis',(0.,0.,1.));
#30139=DIRECTION('ref_axis',(1.,0.,0.));
#30140=DIRECTION('',(0.,0.,-1.));
#30141=DIRECTION('center_axis',(0.,0.,1.));
#30142=DIRECTION('ref_axis',(1.,0.,0.));
#30143=DIRECTION('',(0.,0.,-1.));
#30144=DIRECTION('center_axis',(0.,0.,1.));
#30145=DIRECTION('ref_axis',(1.,0.,0.));
#30146=DIRECTION('',(0.,0.,-1.));
#30147=DIRECTION('center_axis',(0.,0.,1.));
#30148=DIRECTION('ref_axis',(1.,0.,0.));
#30149=DIRECTION('',(0.,0.,-1.));
#30150=DIRECTION('center_axis',(0.,0.,1.));
#30151=DIRECTION('ref_axis',(1.,0.,0.));
#30152=DIRECTION('',(0.,0.,-1.));
#30153=DIRECTION('center_axis',(0.,0.,1.));
#30154=DIRECTION('ref_axis',(1.,0.,0.));
#30155=DIRECTION('',(0.,0.,-1.));
#30156=DIRECTION('center_axis',(0.,0.,1.));
#30157=DIRECTION('ref_axis',(1.,0.,0.));
#30158=DIRECTION('',(0.,0.,-1.));
#30159=DIRECTION('center_axis',(0.,0.,1.));
#30160=DIRECTION('ref_axis',(1.,0.,0.));
#30161=DIRECTION('',(0.,0.,-1.));
#30162=DIRECTION('center_axis',(0.,0.,1.));
#30163=DIRECTION('ref_axis',(1.,0.,0.));
#30164=DIRECTION('',(0.,0.,-1.));
#30165=DIRECTION('center_axis',(0.,0.,1.));
#30166=DIRECTION('ref_axis',(1.,0.,0.));
#30167=DIRECTION('',(0.,0.,-1.));
#30168=DIRECTION('center_axis',(0.,0.,1.));
#30169=DIRECTION('ref_axis',(1.,0.,0.));
#30170=DIRECTION('',(0.,0.,-1.));
#30171=DIRECTION('center_axis',(0.,0.,1.));
#30172=DIRECTION('ref_axis',(1.,0.,0.));
#30173=DIRECTION('',(0.,0.,-1.));
#30174=DIRECTION('center_axis',(0.,0.,1.));
#30175=DIRECTION('ref_axis',(1.,0.,0.));
#30176=DIRECTION('',(0.,0.,-1.));
#30177=DIRECTION('center_axis',(0.,0.,1.));
#30178=DIRECTION('ref_axis',(1.,0.,0.));
#30179=DIRECTION('',(0.,0.,-1.));
#30180=DIRECTION('center_axis',(0.,0.,1.));
#30181=DIRECTION('ref_axis',(1.,0.,0.));
#30182=DIRECTION('',(0.,0.,-1.));
#30183=DIRECTION('center_axis',(0.,0.,1.));
#30184=DIRECTION('ref_axis',(1.,0.,0.));
#30185=DIRECTION('',(0.,0.,-1.));
#30186=DIRECTION('center_axis',(0.,0.,1.));
#30187=DIRECTION('ref_axis',(1.,0.,0.));
#30188=DIRECTION('',(0.,0.,-1.));
#30189=DIRECTION('center_axis',(0.,0.,1.));
#30190=DIRECTION('ref_axis',(1.,0.,0.));
#30191=DIRECTION('',(0.,0.,-1.));
#30192=DIRECTION('center_axis',(0.,0.,1.));
#30193=DIRECTION('ref_axis',(1.,0.,0.));
#30194=DIRECTION('',(0.,0.,-1.));
#30195=DIRECTION('center_axis',(0.,0.,1.));
#30196=DIRECTION('ref_axis',(1.,0.,0.));
#30197=DIRECTION('',(0.,0.,-1.));
#30198=DIRECTION('center_axis',(0.,0.,1.));
#30199=DIRECTION('ref_axis',(1.,0.,0.));
#30200=DIRECTION('',(0.,0.,-1.));
#30201=DIRECTION('center_axis',(0.,0.,1.));
#30202=DIRECTION('ref_axis',(1.,0.,0.));
#30203=DIRECTION('',(0.,0.,-1.));
#30204=DIRECTION('center_axis',(0.,0.,1.));
#30205=DIRECTION('ref_axis',(-0.222283644230434,-0.974982041633402,0.));
#30206=DIRECTION('',(0.,0.,1.));
#30207=DIRECTION('center_axis',(0.,0.,1.));
#30208=DIRECTION('ref_axis',(1.,-9.62097198987423E-13,0.));
#30209=DIRECTION('center_axis',(0.,0.,1.));
#30210=DIRECTION('ref_axis',(1.,-9.62097198987423E-13,0.));
#30211=DIRECTION('',(0.,0.,1.));
#30212=DIRECTION('center_axis',(0.,0.,1.));
#30213=DIRECTION('ref_axis',(1.,-9.62097198987423E-13,0.));
#30214=DIRECTION('',(0.,0.,1.));
#30215=DIRECTION('center_axis',(0.,0.,1.));
#30216=DIRECTION('ref_axis',(1.,-9.62097198987423E-13,0.));
#30217=DIRECTION('',(0.,0.,1.));
#30218=DIRECTION('center_axis',(0.,0.,1.));
#30219=DIRECTION('ref_axis',(1.,-9.62097198987423E-13,0.));
#30220=DIRECTION('',(0.,0.,1.));
#30221=DIRECTION('center_axis',(0.,0.,1.));
#30222=DIRECTION('ref_axis',(1.,-9.62097198987423E-13,0.));
#30223=DIRECTION('',(0.,0.,1.));
#30224=DIRECTION('center_axis',(0.,0.,1.));
#30225=DIRECTION('ref_axis',(1.,-9.62097198987423E-13,0.));
#30226=DIRECTION('',(0.,0.,1.));
#30227=DIRECTION('center_axis',(0.,0.,1.));
#30228=DIRECTION('ref_axis',(1.,-9.62097198987423E-13,0.));
#30229=DIRECTION('',(0.,0.,1.));
#30230=DIRECTION('center_axis',(0.,0.,1.));
#30231=DIRECTION('ref_axis',(1.,-9.62097198987423E-13,0.));
#30232=DIRECTION('',(0.,0.,1.));
#30233=DIRECTION('center_axis',(0.,0.,1.));
#30234=DIRECTION('ref_axis',(1.,-9.62097198987423E-13,0.));
#30235=DIRECTION('',(0.,0.,1.));
#30236=DIRECTION('center_axis',(0.,0.,1.));
#30237=DIRECTION('ref_axis',(1.,-9.62097198987423E-13,0.));
#30238=DIRECTION('',(0.,0.,1.));
#30239=DIRECTION('center_axis',(0.,0.,1.));
#30240=DIRECTION('ref_axis',(1.,-9.62097198987423E-13,0.));
#30241=DIRECTION('',(0.,0.,1.));
#30242=DIRECTION('center_axis',(0.,0.,1.));
#30243=DIRECTION('ref_axis',(1.,-9.62097198987423E-13,0.));
#30244=DIRECTION('',(0.,0.,1.));
#30245=DIRECTION('center_axis',(0.,0.,1.));
#30246=DIRECTION('ref_axis',(1.,-9.62097198987423E-13,0.));
#30247=DIRECTION('',(0.,0.,1.));
#30248=DIRECTION('center_axis',(0.,0.,1.));
#30249=DIRECTION('ref_axis',(1.,-9.62097198987423E-13,0.));
#30250=DIRECTION('',(0.,0.,1.));
#30251=DIRECTION('center_axis',(0.,0.,1.));
#30252=DIRECTION('ref_axis',(1.,-9.62097198987423E-13,0.));
#30253=DIRECTION('',(0.,0.,1.));
#30254=DIRECTION('center_axis',(0.,0.,1.));
#30255=DIRECTION('ref_axis',(1.,-9.62097198987423E-13,0.));
#30256=DIRECTION('',(0.,0.,1.));
#30257=DIRECTION('center_axis',(0.,0.,1.));
#30258=DIRECTION('ref_axis',(1.,-9.62097198987423E-13,0.));
#30259=DIRECTION('',(0.,0.,1.));
#30260=DIRECTION('center_axis',(0.,0.,1.));
#30261=DIRECTION('ref_axis',(1.,-9.62097198987423E-13,0.));
#30262=DIRECTION('',(0.,0.,1.));
#30263=DIRECTION('center_axis',(0.,0.,1.));
#30264=DIRECTION('ref_axis',(1.,-9.62097198987423E-13,0.));
#30265=DIRECTION('',(0.,0.,1.));
#30266=DIRECTION('center_axis',(0.,0.,1.));
#30267=DIRECTION('ref_axis',(1.,-9.62097198987423E-13,0.));
#30268=DIRECTION('',(0.,0.,1.));
#30269=DIRECTION('center_axis',(0.,0.,1.));
#30270=DIRECTION('ref_axis',(1.,-9.62097198987423E-13,0.));
#30271=DIRECTION('',(0.,0.,1.));
#30272=DIRECTION('center_axis',(0.,0.,1.));
#30273=DIRECTION('ref_axis',(1.,-9.62097198987423E-13,0.));
#30274=DIRECTION('',(0.,0.,1.));
#30275=DIRECTION('center_axis',(0.,0.,1.));
#30276=DIRECTION('ref_axis',(1.,-9.62097198987423E-13,0.));
#30277=DIRECTION('',(0.,0.,1.));
#30278=DIRECTION('center_axis',(0.,0.,1.));
#30279=DIRECTION('ref_axis',(1.,-9.62097198987423E-13,0.));
#30280=DIRECTION('',(0.,0.,1.));
#30281=DIRECTION('center_axis',(0.,0.,1.));
#30282=DIRECTION('ref_axis',(1.,-9.62097198987423E-13,0.));
#30283=DIRECTION('',(0.,0.,1.));
#30284=DIRECTION('center_axis',(0.,0.,1.));
#30285=DIRECTION('ref_axis',(1.,-9.62097198987423E-13,0.));
#30286=DIRECTION('',(0.,0.,1.));
#30287=DIRECTION('center_axis',(0.,0.,1.));
#30288=DIRECTION('ref_axis',(1.,-9.62097198987423E-13,0.));
#30289=DIRECTION('',(0.,0.,1.));
#30290=DIRECTION('center_axis',(0.,0.,1.));
#30291=DIRECTION('ref_axis',(1.,-9.62097198987423E-13,0.));
#30292=DIRECTION('',(0.,0.,1.));
#30293=DIRECTION('center_axis',(0.,0.,1.));
#30294=DIRECTION('ref_axis',(1.,-9.62097198987423E-13,0.));
#30295=DIRECTION('',(0.,0.,1.));
#30296=DIRECTION('center_axis',(0.,0.,1.));
#30297=DIRECTION('ref_axis',(1.,-9.62097198987423E-13,0.));
#30298=DIRECTION('',(0.,0.,1.));
#30299=DIRECTION('center_axis',(0.,0.,1.));
#30300=DIRECTION('ref_axis',(1.,-9.62097198987423E-13,0.));
#30301=DIRECTION('',(0.,0.,1.));
#30302=DIRECTION('center_axis',(0.,0.,1.));
#30303=DIRECTION('ref_axis',(1.,-9.62097198987423E-13,0.));
#30304=DIRECTION('',(0.,0.,1.));
#30305=DIRECTION('center_axis',(0.,0.,1.));
#30306=DIRECTION('ref_axis',(1.,-9.62097198987423E-13,0.));
#30307=DIRECTION('',(0.,0.,1.));
#30308=DIRECTION('center_axis',(0.,0.,1.));
#30309=DIRECTION('ref_axis',(1.,-9.62097198987423E-13,0.));
#30310=DIRECTION('',(0.,0.,1.));
#30311=DIRECTION('center_axis',(0.,0.,1.));
#30312=DIRECTION('ref_axis',(1.,-9.62097198987423E-13,0.));
#30313=DIRECTION('',(0.,0.,1.));
#30314=DIRECTION('center_axis',(0.,0.,1.));
#30315=DIRECTION('ref_axis',(1.,-9.62097198987423E-13,0.));
#30316=DIRECTION('',(0.,0.,1.));
#30317=DIRECTION('center_axis',(0.,0.,1.));
#30318=DIRECTION('ref_axis',(1.,-9.62097198987423E-13,0.));
#30319=DIRECTION('',(0.,0.,1.));
#30320=DIRECTION('center_axis',(0.,0.,1.));
#30321=DIRECTION('ref_axis',(1.,-9.62097198987423E-13,0.));
#30322=DIRECTION('',(0.,0.,1.));
#30323=DIRECTION('center_axis',(0.,0.,1.));
#30324=DIRECTION('ref_axis',(1.,-9.62097198987423E-13,0.));
#30325=DIRECTION('',(0.,0.,1.));
#30326=DIRECTION('center_axis',(0.,0.,1.));
#30327=DIRECTION('ref_axis',(1.,-9.62097198987423E-13,0.));
#30328=DIRECTION('',(0.,0.,1.));
#30329=DIRECTION('center_axis',(0.,0.,1.));
#30330=DIRECTION('ref_axis',(1.,-9.62097198987423E-13,0.));
#30331=DIRECTION('',(0.,0.,1.));
#30332=DIRECTION('center_axis',(0.,0.,1.));
#30333=DIRECTION('ref_axis',(1.,-9.62097198987423E-13,0.));
#30334=DIRECTION('',(0.,0.,1.));
#30335=DIRECTION('center_axis',(0.,0.,1.));
#30336=DIRECTION('ref_axis',(1.,-9.62097198987423E-13,0.));
#30337=DIRECTION('',(0.,0.,1.));
#30338=DIRECTION('center_axis',(0.,0.,1.));
#30339=DIRECTION('ref_axis',(1.,-9.62097198987423E-13,0.));
#30340=DIRECTION('',(0.,0.,1.));
#30341=DIRECTION('center_axis',(0.,0.,1.));
#30342=DIRECTION('ref_axis',(1.,-9.62097198987423E-13,0.));
#30343=DIRECTION('',(0.,0.,1.));
#30344=DIRECTION('center_axis',(0.,0.,1.));
#30345=DIRECTION('ref_axis',(1.,-9.62097198987423E-13,0.));
#30346=DIRECTION('',(0.,0.,1.));
#30347=DIRECTION('center_axis',(0.,0.,1.));
#30348=DIRECTION('ref_axis',(1.,-9.62097198987423E-13,0.));
#30349=DIRECTION('',(0.,0.,1.));
#30350=DIRECTION('center_axis',(0.,0.,1.));
#30351=DIRECTION('ref_axis',(1.,-9.62097198987423E-13,0.));
#30352=DIRECTION('',(0.,0.,1.));
#30353=DIRECTION('center_axis',(0.,0.,1.));
#30354=DIRECTION('ref_axis',(1.,-9.62097198987423E-13,0.));
#30355=DIRECTION('',(0.,0.,1.));
#30356=DIRECTION('center_axis',(0.,0.,1.));
#30357=DIRECTION('ref_axis',(1.,-9.62097198987423E-13,0.));
#30358=DIRECTION('',(0.,0.,1.));
#30359=DIRECTION('center_axis',(0.,0.,1.));
#30360=DIRECTION('ref_axis',(1.,-9.62097198987423E-13,0.));
#30361=DIRECTION('',(0.,0.,1.));
#30362=DIRECTION('center_axis',(0.,0.,1.));
#30363=DIRECTION('ref_axis',(1.,-9.62097198987423E-13,0.));
#30364=DIRECTION('',(0.,0.,1.));
#30365=DIRECTION('center_axis',(0.,0.,1.));
#30366=DIRECTION('ref_axis',(1.,-9.62097198987423E-13,0.));
#30367=DIRECTION('',(0.,0.,1.));
#30368=DIRECTION('center_axis',(0.,0.,1.));
#30369=DIRECTION('ref_axis',(1.,-9.62097198987423E-13,0.));
#30370=DIRECTION('',(0.,0.,1.));
#30371=DIRECTION('center_axis',(0.,0.,1.));
#30372=DIRECTION('ref_axis',(1.,-9.62097198987423E-13,0.));
#30373=DIRECTION('',(0.,0.,1.));
#30374=DIRECTION('center_axis',(0.,0.,1.));
#30375=DIRECTION('ref_axis',(1.,-9.62097198987423E-13,0.));
#30376=DIRECTION('',(0.,0.,1.));
#30377=DIRECTION('center_axis',(0.,0.,1.));
#30378=DIRECTION('ref_axis',(1.,-9.62097198987423E-13,0.));
#30379=DIRECTION('',(0.,0.,1.));
#30380=DIRECTION('center_axis',(0.,0.,1.));
#30381=DIRECTION('ref_axis',(1.,-9.62097198987423E-13,0.));
#30382=DIRECTION('',(0.,0.,1.));
#30383=DIRECTION('center_axis',(0.,0.,1.));
#30384=DIRECTION('ref_axis',(1.,0.,0.));
#30385=DIRECTION('center_axis',(0.,0.,1.));
#30386=DIRECTION('ref_axis',(1.,0.,0.));
#30387=DIRECTION('center_axis',(0.,0.,1.));
#30388=DIRECTION('ref_axis',(1.,0.,0.));
#30389=DIRECTION('center_axis',(0.,0.,1.));
#30390=DIRECTION('ref_axis',(1.,0.,0.));
#30391=DIRECTION('center_axis',(0.,0.,-1.));
#30392=DIRECTION('ref_axis',(1.,-9.62097198987423E-13,0.));
#30393=DIRECTION('center_axis',(0.,0.,1.));
#30394=DIRECTION('ref_axis',(-0.710035149338663,0.70416623513459,0.));
#30395=DIRECTION('center_axis',(0.,0.,1.));
#30396=DIRECTION('ref_axis',(0.984807753012208,-0.17364817766693,0.));
#30397=DIRECTION('center_axis',(0.,0.,-1.));
#30398=DIRECTION('ref_axis',(1.,0.,0.));
#30399=DIRECTION('',(-0.996089805327885,-0.0883464754353932,0.));
#30400=DIRECTION('',(0.905801965515954,-0.423701309022563,0.));
#30401=DIRECTION('center_axis',(-0.423701309022563,-0.905801965515954,0.));
#30402=DIRECTION('ref_axis',(0.905801965515954,-0.423701309022563,0.));
#30403=DIRECTION('',(0.,0.,1.));
#30404=DIRECTION('',(0.,0.,1.));
#30405=DIRECTION('center_axis',(-0.0883464754353932,0.996089805327885,0.));
#30406=DIRECTION('ref_axis',(-0.996089805327885,-0.0883464754353932,0.));
#30407=DIRECTION('',(0.,0.,-1.));
#30408=DIRECTION('center_axis',(0.,0.,1.));
#30409=DIRECTION('ref_axis',(0.939692620785908,-0.342020143325669,0.));
#30410=DIRECTION('center_axis',(0.,0.,-1.));
#30411=DIRECTION('ref_axis',(1.,0.,0.));
#30412=DIRECTION('',(-0.996298167445974,0.0859648855277176,0.));
#30413=DIRECTION('',(0.818465838146947,-0.574555194725812,0.));
#30414=DIRECTION('center_axis',(-0.574555194725812,-0.818465838146947,0.));
#30415=DIRECTION('ref_axis',(0.818465838146947,-0.574555194725812,0.));
#30416=DIRECTION('',(0.,0.,1.));
#30417=DIRECTION('',(0.,0.,1.));
#30418=DIRECTION('center_axis',(0.0859648855277176,0.996298167445974,0.));
#30419=DIRECTION('ref_axis',(-0.996298167445974,0.0859648855277176,0.));
#30420=DIRECTION('',(0.,0.,-1.));
#30421=DIRECTION('center_axis',(0.,0.,1.));
#30422=DIRECTION('ref_axis',(0.866025403784438,-0.5,0.));
#30423=DIRECTION('center_axis',(0.,0.,-1.));
#30424=DIRECTION('ref_axis',(1.,0.,0.));
#30425=DIRECTION('',(-0.966234513897416,0.257664246944399,0.));
#30426=DIRECTION('',(0.706261040449543,-0.707951511576272,0.));
#30427=DIRECTION('center_axis',(-0.707951511576272,-0.706261040449543,0.));
#30428=DIRECTION('ref_axis',(0.706261040449543,-0.707951511576272,0.));
#30429=DIRECTION('',(0.,0.,1.));
#30430=DIRECTION('',(0.,0.,1.));
#30431=DIRECTION('center_axis',(0.257664246944399,0.966234513897416,0.));
#30432=DIRECTION('ref_axis',(-0.966234513897416,0.257664246944399,0.));
#30433=DIRECTION('',(0.,0.,-1.));
#30434=DIRECTION('center_axis',(0.,0.,1.));
#30435=DIRECTION('ref_axis',(0.766044443118978,-0.64278760968654,0.));
#30436=DIRECTION('center_axis',(0.,0.,-1.));
#30437=DIRECTION('ref_axis',(1.,0.,0.));
#30438=DIRECTION('',(-0.906812313582341,0.421534610602074,0.));
#30439=DIRECTION('',(0.572596858423411,-0.819837079988238,0.));
#30440=DIRECTION('center_axis',(-0.819837079988238,-0.572596858423411,0.));
#30441=DIRECTION('ref_axis',(0.572596858423411,-0.819837079988238,0.));
#30442=DIRECTION('',(0.,0.,1.));
#30443=DIRECTION('',(0.,0.,1.));
#30444=DIRECTION('center_axis',(0.421534610602074,0.906812313582341,0.));
#30445=DIRECTION('ref_axis',(-0.906812313582341,0.421534610602074,0.));
#30446=DIRECTION('',(0.,0.,-1.));
#30447=DIRECTION('center_axis',(0.,0.,1.));
#30448=DIRECTION('ref_axis',(0.642787609686539,-0.766044443118978,0.));
#30449=DIRECTION('center_axis',(0.,0.,-1.));
#30450=DIRECTION('ref_axis',(1.,0.,0.));
#30451=DIRECTION('',(-0.819837079988238,0.572596858423411,0.));
#30452=DIRECTION('',(0.421534610602074,-0.906812313582341,0.));
#30453=DIRECTION('center_axis',(-0.906812313582341,-0.421534610602074,0.));
#30454=DIRECTION('ref_axis',(0.421534610602074,-0.906812313582341,0.));
#30455=DIRECTION('',(0.,0.,1.));
#30456=DIRECTION('',(0.,0.,1.));
#30457=DIRECTION('center_axis',(0.572596858423411,0.819837079988238,0.));
#30458=DIRECTION('ref_axis',(-0.819837079988238,0.572596858423411,0.));
#30459=DIRECTION('',(0.,0.,-1.));
#30460=DIRECTION('center_axis',(0.,0.,1.));
#30461=DIRECTION('ref_axis',(0.5,-0.866025403784438,0.));
#30462=DIRECTION('center_axis',(0.,0.,-1.));
#30463=DIRECTION('ref_axis',(1.,0.,0.));
#30464=DIRECTION('',(-0.707951511576272,0.706261040449544,0.));
#30465=DIRECTION('',(0.257664246944398,-0.966234513897416,0.));
#30466=DIRECTION('center_axis',(-0.966234513897416,-0.257664246944398,0.));
#30467=DIRECTION('ref_axis',(0.257664246944398,-0.966234513897416,0.));
#30468=DIRECTION('',(0.,0.,1.));
#30469=DIRECTION('',(0.,0.,1.));
#30470=DIRECTION('center_axis',(0.706261040449544,0.707951511576272,0.));
#30471=DIRECTION('ref_axis',(-0.707951511576272,0.706261040449544,0.));
#30472=DIRECTION('',(0.,0.,-1.));
#30473=DIRECTION('center_axis',(0.,0.,1.));
#30474=DIRECTION('ref_axis',(0.342020143325668,-0.939692620785909,0.));
#30475=DIRECTION('center_axis',(0.,0.,-1.));
#30476=DIRECTION('ref_axis',(1.,0.,0.));
#30477=DIRECTION('',(-0.57455519472581,0.818465838146948,0.));
#30478=DIRECTION('',(0.0859648855277162,-0.996298167445974,0.));
#30479=DIRECTION('center_axis',(-0.996298167445974,-0.0859648855277162,
0.));
#30480=DIRECTION('ref_axis',(0.0859648855277162,-0.996298167445974,0.));
#30481=DIRECTION('',(0.,0.,1.));
#30482=DIRECTION('',(0.,0.,1.));
#30483=DIRECTION('center_axis',(0.818465838146948,0.57455519472581,0.));
#30484=DIRECTION('ref_axis',(-0.57455519472581,0.818465838146948,0.));
#30485=DIRECTION('',(0.,0.,-1.));
#30486=DIRECTION('center_axis',(0.,0.,1.));
#30487=DIRECTION('ref_axis',(0.17364817766693,-0.984807753012208,0.));
#30488=DIRECTION('center_axis',(0.,0.,-1.));
#30489=DIRECTION('ref_axis',(1.,0.,0.));
#30490=DIRECTION('',(-0.423701309022563,0.905801965515955,0.));
#30491=DIRECTION('',(-0.0883464754353936,-0.996089805327885,0.));
#30492=DIRECTION('center_axis',(-0.996089805327885,0.0883464754353937,0.));
#30493=DIRECTION('ref_axis',(-0.0883464754353937,-0.996089805327885,0.));
#30494=DIRECTION('',(0.,0.,1.));
#30495=DIRECTION('',(0.,0.,1.));
#30496=DIRECTION('center_axis',(0.905801965515955,0.423701309022563,0.));
#30497=DIRECTION('ref_axis',(-0.423701309022563,0.905801965515955,0.));
#30498=DIRECTION('',(0.,0.,-1.));
#30499=DIRECTION('center_axis',(0.,0.,1.));
#30500=DIRECTION('ref_axis',(-1.94289029309402E-16,-1.,0.));
#30501=DIRECTION('center_axis',(0.,0.,-1.));
#30502=DIRECTION('ref_axis',(1.,0.,0.));
#30503=DIRECTION('',(-0.259973473447872,0.96561575852067,0.));
#30504=DIRECTION('',(-0.259973473447873,-0.96561575852067,0.));
#30505=DIRECTION('center_axis',(-0.96561575852067,0.259973473447873,0.));
#30506=DIRECTION('ref_axis',(-0.259973473447873,-0.96561575852067,0.));
#30507=DIRECTION('',(0.,0.,1.));
#30508=DIRECTION('',(0.,0.,1.));
#30509=DIRECTION('center_axis',(0.96561575852067,0.259973473447872,0.));
#30510=DIRECTION('ref_axis',(-0.259973473447872,0.96561575852067,0.));
#30511=DIRECTION('',(0.,0.,-1.));
#30512=DIRECTION('center_axis',(0.,0.,1.));
#30513=DIRECTION('ref_axis',(-0.17364817766693,-0.984807753012208,0.));
#30514=DIRECTION('center_axis',(0.,0.,-1.));
#30515=DIRECTION('ref_axis',(1.,0.,0.));
#30516=DIRECTION('',(-0.0883464754353933,0.996089805327885,0.));
#30517=DIRECTION('',(-0.423701309022563,-0.905801965515955,0.));
#30518=DIRECTION('center_axis',(-0.905801965515955,0.423701309022563,0.));
#30519=DIRECTION('ref_axis',(-0.423701309022563,-0.905801965515955,0.));
#30520=DIRECTION('',(0.,0.,1.));
#30521=DIRECTION('',(0.,0.,1.));
#30522=DIRECTION('center_axis',(0.996089805327885,0.0883464754353932,0.));
#30523=DIRECTION('ref_axis',(-0.0883464754353932,0.996089805327885,0.));
#30524=DIRECTION('',(0.,0.,-1.));
#30525=DIRECTION('center_axis',(0.,0.,1.));
#30526=DIRECTION('ref_axis',(-0.342020143325669,-0.939692620785908,0.));
#30527=DIRECTION('center_axis',(0.,0.,-1.));
#30528=DIRECTION('ref_axis',(1.,0.,0.));
#30529=DIRECTION('',(0.0859648855277175,0.996298167445974,0.));
#30530=DIRECTION('',(-0.574555194725811,-0.818465838146947,0.));
#30531=DIRECTION('center_axis',(-0.818465838146947,0.574555194725811,0.));
#30532=DIRECTION('ref_axis',(-0.574555194725811,-0.818465838146947,0.));
#30533=DIRECTION('',(0.,0.,1.));
#30534=DIRECTION('',(0.,0.,1.));
#30535=DIRECTION('center_axis',(0.996298167445974,-0.0859648855277175,0.));
#30536=DIRECTION('ref_axis',(0.0859648855277175,0.996298167445974,0.));
#30537=DIRECTION('',(0.,0.,-1.));
#30538=DIRECTION('center_axis',(0.,0.,1.));
#30539=DIRECTION('ref_axis',(-0.5,-0.866025403784438,0.));
#30540=DIRECTION('center_axis',(0.,0.,-1.));
#30541=DIRECTION('ref_axis',(1.,0.,0.));
#30542=DIRECTION('',(0.257664246944399,0.966234513897416,0.));
#30543=DIRECTION('',(-0.707951511576272,-0.706261040449543,0.));
#30544=DIRECTION('center_axis',(-0.706261040449543,0.707951511576272,0.));
#30545=DIRECTION('ref_axis',(-0.707951511576272,-0.706261040449543,0.));
#30546=DIRECTION('',(0.,0.,1.));
#30547=DIRECTION('',(0.,0.,1.));
#30548=DIRECTION('center_axis',(0.966234513897416,-0.257664246944399,0.));
#30549=DIRECTION('ref_axis',(0.257664246944399,0.966234513897416,0.));
#30550=DIRECTION('',(0.,0.,-1.));
#30551=DIRECTION('center_axis',(0.,0.,1.));
#30552=DIRECTION('ref_axis',(-0.642787609686539,-0.766044443118978,0.));
#30553=DIRECTION('center_axis',(0.,0.,-1.));
#30554=DIRECTION('ref_axis',(1.,0.,0.));
#30555=DIRECTION('',(0.421534610602074,0.906812313582341,0.));
#30556=DIRECTION('',(-0.819837079988238,-0.572596858423411,0.));
#30557=DIRECTION('center_axis',(-0.572596858423411,0.819837079988238,0.));
#30558=DIRECTION('ref_axis',(-0.819837079988238,-0.572596858423411,0.));
#30559=DIRECTION('',(0.,0.,1.));
#30560=DIRECTION('',(0.,0.,1.));
#30561=DIRECTION('center_axis',(0.906812313582341,-0.421534610602074,0.));
#30562=DIRECTION('ref_axis',(0.421534610602074,0.906812313582341,0.));
#30563=DIRECTION('',(0.,0.,-1.));
#30564=DIRECTION('center_axis',(0.,0.,1.));
#30565=DIRECTION('ref_axis',(-0.766044443118978,-0.642787609686539,0.));
#30566=DIRECTION('center_axis',(0.,0.,-1.));
#30567=DIRECTION('ref_axis',(1.,0.,0.));
#30568=DIRECTION('',(0.572596858423411,0.819837079988238,0.));
#30569=DIRECTION('',(-0.906812313582341,-0.421534610602074,0.));
#30570=DIRECTION('center_axis',(-0.421534610602074,0.906812313582341,0.));
#30571=DIRECTION('ref_axis',(-0.906812313582341,-0.421534610602074,0.));
#30572=DIRECTION('',(0.,0.,1.));
#30573=DIRECTION('',(0.,0.,1.));
#30574=DIRECTION('center_axis',(0.819837079988238,-0.572596858423411,0.));
#30575=DIRECTION('ref_axis',(0.572596858423411,0.819837079988238,0.));
#30576=DIRECTION('',(0.,0.,-1.));
#30577=DIRECTION('center_axis',(0.,0.,1.));
#30578=DIRECTION('ref_axis',(-0.866025403784439,-0.5,0.));
#30579=DIRECTION('center_axis',(0.,0.,-1.));
#30580=DIRECTION('ref_axis',(1.,0.,0.));
#30581=DIRECTION('',(0.706261040449544,0.707951511576271,0.));
#30582=DIRECTION('',(-0.966234513897416,-0.257664246944398,0.));
#30583=DIRECTION('center_axis',(-0.257664246944398,0.966234513897416,0.));
#30584=DIRECTION('ref_axis',(-0.966234513897416,-0.257664246944398,0.));
#30585=DIRECTION('',(0.,0.,1.));
#30586=DIRECTION('',(0.,0.,1.));
#30587=DIRECTION('center_axis',(0.707951511576271,-0.706261040449544,0.));
#30588=DIRECTION('ref_axis',(0.706261040449544,0.707951511576271,0.));
#30589=DIRECTION('',(0.,0.,-1.));
#30590=DIRECTION('center_axis',(0.,0.,1.));
#30591=DIRECTION('ref_axis',(-0.939692620785909,-0.342020143325669,0.));
#30592=DIRECTION('center_axis',(0.,0.,-1.));
#30593=DIRECTION('ref_axis',(1.,0.,0.));
#30594=DIRECTION('',(0.818465838146948,0.574555194725811,0.));
#30595=DIRECTION('',(-0.996298167445974,-0.0859648855277167,0.));
#30596=DIRECTION('center_axis',(-0.0859648855277167,0.996298167445974,0.));
#30597=DIRECTION('ref_axis',(-0.996298167445974,-0.0859648855277167,0.));
#30598=DIRECTION('',(0.,0.,1.));
#30599=DIRECTION('',(0.,0.,1.));
#30600=DIRECTION('center_axis',(0.574555194725811,-0.818465838146948,0.));
#30601=DIRECTION('ref_axis',(0.818465838146948,0.574555194725811,0.));
#30602=DIRECTION('',(0.,0.,-1.));
#30603=DIRECTION('center_axis',(0.,0.,1.));
#30604=DIRECTION('ref_axis',(-0.984807753012208,-0.17364817766693,0.));
#30605=DIRECTION('center_axis',(0.,0.,-1.));
#30606=DIRECTION('ref_axis',(1.,0.,0.));
#30607=DIRECTION('',(0.905801965515955,0.423701309022563,0.));
#30608=DIRECTION('',(-0.996089805327885,0.0883464754353936,0.));
#30609=DIRECTION('center_axis',(0.0883464754353936,0.996089805327885,0.));
#30610=DIRECTION('ref_axis',(-0.996089805327885,0.0883464754353936,0.));
#30611=DIRECTION('',(0.,0.,1.));
#30612=DIRECTION('',(0.,0.,1.));
#30613=DIRECTION('center_axis',(0.423701309022563,-0.905801965515955,0.));
#30614=DIRECTION('ref_axis',(0.905801965515955,0.423701309022563,0.));
#30615=DIRECTION('',(0.,0.,-1.));
#30616=DIRECTION('center_axis',(0.,0.,1.));
#30617=DIRECTION('ref_axis',(-1.,1.11022302462516E-16,0.));
#30618=DIRECTION('center_axis',(0.,0.,-1.));
#30619=DIRECTION('ref_axis',(1.,0.,0.));
#30620=DIRECTION('',(0.96561575852067,0.259973473447872,0.));
#30621=DIRECTION('',(-0.96561575852067,0.259973473447873,0.));
#30622=DIRECTION('center_axis',(0.,0.,-1.));
#30623=DIRECTION('ref_axis',(1.,0.,0.));
#30624=DIRECTION('center_axis',(0.259973473447873,0.96561575852067,0.));
#30625=DIRECTION('ref_axis',(-0.96561575852067,0.259973473447873,0.));
#30626=DIRECTION('',(0.,0.,1.));
#30627=DIRECTION('',(0.,0.,1.));
#30628=DIRECTION('center_axis',(0.259973473447872,-0.96561575852067,0.));
#30629=DIRECTION('ref_axis',(0.96561575852067,0.259973473447872,0.));
#30630=DIRECTION('',(0.,0.,-1.));
#30631=DIRECTION('center_axis',(0.,0.,1.));
#30632=DIRECTION('ref_axis',(-0.984807753012208,0.173648177666931,0.));
#30633=DIRECTION('center_axis',(0.,0.,-1.));
#30634=DIRECTION('ref_axis',(1.,0.,0.));
#30635=DIRECTION('',(0.996089805327885,0.0883464754353928,0.));
#30636=DIRECTION('',(-0.905801965515954,0.423701309022564,0.));
#30637=DIRECTION('center_axis',(0.423701309022564,0.905801965515954,0.));
#30638=DIRECTION('ref_axis',(-0.905801965515954,0.423701309022564,0.));
#30639=DIRECTION('',(0.,0.,1.));
#30640=DIRECTION('',(0.,0.,1.));
#30641=DIRECTION('center_axis',(0.0883464754353928,-0.996089805327885,0.));
#30642=DIRECTION('ref_axis',(0.996089805327885,0.0883464754353928,0.));
#30643=DIRECTION('',(0.,0.,-1.));
#30644=DIRECTION('center_axis',(0.,0.,1.));
#30645=DIRECTION('ref_axis',(-0.939692620785908,0.342020143325669,0.));
#30646=DIRECTION('center_axis',(0.,0.,-1.));
#30647=DIRECTION('ref_axis',(1.,0.,0.));
#30648=DIRECTION('',(0.996298167445974,-0.085964885527717,0.));
#30649=DIRECTION('',(-0.818465838146948,0.574555194725811,0.));
#30650=DIRECTION('center_axis',(0.574555194725811,0.818465838146948,0.));
#30651=DIRECTION('ref_axis',(-0.818465838146948,0.574555194725811,0.));
#30652=DIRECTION('',(0.,0.,1.));
#30653=DIRECTION('',(0.,0.,1.));
#30654=DIRECTION('center_axis',(-0.085964885527717,-0.996298167445974,0.));
#30655=DIRECTION('ref_axis',(0.996298167445974,-0.085964885527717,0.));
#30656=DIRECTION('',(0.,0.,-1.));
#30657=DIRECTION('center_axis',(0.,0.,1.));
#30658=DIRECTION('ref_axis',(-0.866025403784439,0.5,0.));
#30659=DIRECTION('center_axis',(0.,0.,-1.));
#30660=DIRECTION('ref_axis',(1.,0.,0.));
#30661=DIRECTION('',(0.966234513897416,-0.257664246944398,0.));
#30662=DIRECTION('',(-0.706261040449544,0.707951511576272,0.));
#30663=DIRECTION('center_axis',(0.707951511576272,0.706261040449544,0.));
#30664=DIRECTION('ref_axis',(-0.706261040449544,0.707951511576272,0.));
#30665=DIRECTION('',(0.,0.,1.));
#30666=DIRECTION('',(0.,0.,1.));
#30667=DIRECTION('center_axis',(-0.257664246944398,-0.966234513897416,0.));
#30668=DIRECTION('ref_axis',(0.966234513897416,-0.257664246944398,0.));
#30669=DIRECTION('',(0.,0.,-1.));
#30670=DIRECTION('center_axis',(0.,0.,1.));
#30671=DIRECTION('ref_axis',(-0.766044443118978,0.642787609686539,0.));
#30672=DIRECTION('center_axis',(0.,0.,-1.));
#30673=DIRECTION('ref_axis',(1.,0.,0.));
#30674=DIRECTION('',(0.906812313582341,-0.421534610602074,0.));
#30675=DIRECTION('',(-0.572596858423411,0.819837079988238,0.));
#30676=DIRECTION('center_axis',(0.819837079988238,0.572596858423411,0.));
#30677=DIRECTION('ref_axis',(-0.572596858423411,0.819837079988238,0.));
#30678=DIRECTION('',(0.,0.,1.));
#30679=DIRECTION('',(0.,0.,1.));
#30680=DIRECTION('center_axis',(-0.421534610602074,-0.906812313582341,0.));
#30681=DIRECTION('ref_axis',(0.906812313582341,-0.421534610602074,0.));
#30682=DIRECTION('',(0.,0.,-1.));
#30683=DIRECTION('center_axis',(0.,0.,1.));
#30684=DIRECTION('ref_axis',(-0.642787609686539,0.766044443118978,0.));
#30685=DIRECTION('center_axis',(0.,0.,-1.));
#30686=DIRECTION('ref_axis',(1.,0.,0.));
#30687=DIRECTION('',(0.819837079988238,-0.572596858423411,0.));
#30688=DIRECTION('',(-0.421534610602074,0.906812313582341,0.));
#30689=DIRECTION('center_axis',(0.906812313582341,0.421534610602074,0.));
#30690=DIRECTION('ref_axis',(-0.421534610602074,0.906812313582341,0.));
#30691=DIRECTION('',(0.,0.,1.));
#30692=DIRECTION('',(0.,0.,1.));
#30693=DIRECTION('center_axis',(-0.572596858423411,-0.819837079988238,0.));
#30694=DIRECTION('ref_axis',(0.819837079988238,-0.572596858423411,0.));
#30695=DIRECTION('',(0.,0.,-1.));
#30696=DIRECTION('center_axis',(0.,0.,1.));
#30697=DIRECTION('ref_axis',(-0.5,0.866025403784439,0.));
#30698=DIRECTION('center_axis',(0.,0.,-1.));
#30699=DIRECTION('ref_axis',(1.,0.,0.));
#30700=DIRECTION('',(0.707951511576272,-0.706261040449544,0.));
#30701=DIRECTION('',(-0.257664246944398,0.966234513897416,0.));
#30702=DIRECTION('center_axis',(0.966234513897416,0.257664246944398,0.));
#30703=DIRECTION('ref_axis',(-0.257664246944398,0.966234513897416,0.));
#30704=DIRECTION('',(0.,0.,1.));
#30705=DIRECTION('',(0.,0.,1.));
#30706=DIRECTION('center_axis',(-0.706261040449544,-0.707951511576272,0.));
#30707=DIRECTION('ref_axis',(0.707951511576272,-0.706261040449544,0.));
#30708=DIRECTION('',(0.,0.,-1.));
#30709=DIRECTION('center_axis',(0.,0.,1.));
#30710=DIRECTION('ref_axis',(-0.342020143325669,0.939692620785909,0.));
#30711=DIRECTION('center_axis',(0.,0.,-1.));
#30712=DIRECTION('ref_axis',(1.,0.,0.));
#30713=DIRECTION('',(0.574555194725811,-0.818465838146948,0.));
#30714=DIRECTION('',(-0.0859648855277167,0.996298167445974,0.));
#30715=DIRECTION('center_axis',(0.996298167445974,0.0859648855277167,0.));
#30716=DIRECTION('ref_axis',(-0.0859648855277167,0.996298167445974,0.));
#30717=DIRECTION('',(0.,0.,1.));
#30718=DIRECTION('',(0.,0.,1.));
#30719=DIRECTION('center_axis',(-0.818465838146948,-0.574555194725811,0.));
#30720=DIRECTION('ref_axis',(0.574555194725811,-0.818465838146948,0.));
#30721=DIRECTION('',(0.,0.,-1.));
#30722=DIRECTION('center_axis',(0.,0.,1.));
#30723=DIRECTION('ref_axis',(-0.17364817766693,0.984807753012208,0.));
#30724=DIRECTION('center_axis',(0.,0.,-1.));
#30725=DIRECTION('ref_axis',(1.,0.,0.));
#30726=DIRECTION('',(0.423701309022563,-0.905801965515955,0.));
#30727=DIRECTION('',(0.0883464754353932,0.996089805327885,0.));
#30728=DIRECTION('center_axis',(0.996089805327885,-0.0883464754353932,0.));
#30729=DIRECTION('ref_axis',(0.0883464754353932,0.996089805327885,0.));
#30730=DIRECTION('',(0.,0.,1.));
#30731=DIRECTION('',(0.,0.,1.));
#30732=DIRECTION('center_axis',(-0.905801965515955,-0.423701309022563,0.));
#30733=DIRECTION('ref_axis',(0.423701309022563,-0.905801965515955,0.));
#30734=DIRECTION('',(0.,0.,-1.));
#30735=DIRECTION('center_axis',(0.,0.,1.));
#30736=DIRECTION('ref_axis',(5.55111512312578E-17,1.,0.));
#30737=DIRECTION('center_axis',(0.,0.,-1.));
#30738=DIRECTION('ref_axis',(1.,0.,0.));
#30739=DIRECTION('',(0.259973473447872,-0.96561575852067,0.));
#30740=DIRECTION('',(0.259973473447872,0.96561575852067,0.));
#30741=DIRECTION('center_axis',(0.96561575852067,-0.259973473447873,0.));
#30742=DIRECTION('ref_axis',(0.259973473447873,0.96561575852067,0.));
#30743=DIRECTION('',(0.,0.,1.));
#30744=DIRECTION('',(0.,0.,1.));
#30745=DIRECTION('center_axis',(-0.96561575852067,-0.259973473447872,0.));
#30746=DIRECTION('ref_axis',(0.259973473447872,-0.96561575852067,0.));
#30747=DIRECTION('',(0.,0.,-1.));
#30748=DIRECTION('center_axis',(0.,0.,1.));
#30749=DIRECTION('ref_axis',(0.17364817766693,0.984807753012208,0.));
#30750=DIRECTION('center_axis',(0.,0.,-1.));
#30751=DIRECTION('ref_axis',(1.,0.,0.));
#30752=DIRECTION('',(0.0883464754353931,-0.996089805327885,0.));
#30753=DIRECTION('',(0.423701309022563,0.905801965515954,0.));
#30754=DIRECTION('center_axis',(0.905801965515954,-0.423701309022563,0.));
#30755=DIRECTION('ref_axis',(0.423701309022563,0.905801965515954,0.));
#30756=DIRECTION('',(0.,0.,1.));
#30757=DIRECTION('',(0.,0.,1.));
#30758=DIRECTION('center_axis',(-0.996089805327885,-0.0883464754353932,
0.));
#30759=DIRECTION('ref_axis',(0.0883464754353932,-0.996089805327885,0.));
#30760=DIRECTION('',(0.,0.,-1.));
#30761=DIRECTION('center_axis',(0.,0.,1.));
#30762=DIRECTION('ref_axis',(0.342020143325669,0.939692620785908,0.));
#30763=DIRECTION('center_axis',(0.,0.,-1.));
#30764=DIRECTION('ref_axis',(1.,0.,0.));
#30765=DIRECTION('',(-0.085964885527717,-0.996298167445974,0.));
#30766=DIRECTION('',(0.574555194725811,0.818465838146948,0.));
#30767=DIRECTION('center_axis',(0.818465838146948,-0.574555194725811,0.));
#30768=DIRECTION('ref_axis',(0.574555194725811,0.818465838146948,0.));
#30769=DIRECTION('',(0.,0.,1.));
#30770=DIRECTION('',(0.,0.,1.));
#30771=DIRECTION('center_axis',(-0.996298167445974,0.085964885527717,0.));
#30772=DIRECTION('ref_axis',(-0.085964885527717,-0.996298167445974,0.));
#30773=DIRECTION('',(0.,0.,-1.));
#30774=DIRECTION('center_axis',(0.,0.,1.));
#30775=DIRECTION('ref_axis',(0.5,0.866025403784439,0.));
#30776=DIRECTION('center_axis',(0.,0.,-1.));
#30777=DIRECTION('ref_axis',(1.,0.,0.));
#30778=DIRECTION('',(-0.257664246944398,-0.966234513897416,0.));
#30779=DIRECTION('',(0.707951511576272,0.706261040449544,0.));
#30780=DIRECTION('center_axis',(0.706261040449544,-0.707951511576272,0.));
#30781=DIRECTION('ref_axis',(0.707951511576272,0.706261040449544,0.));
#30782=DIRECTION('',(0.,0.,1.));
#30783=DIRECTION('',(0.,0.,1.));
#30784=DIRECTION('center_axis',(-0.966234513897416,0.257664246944398,0.));
#30785=DIRECTION('ref_axis',(-0.257664246944398,-0.966234513897416,0.));
#30786=DIRECTION('',(0.,0.,-1.));
#30787=DIRECTION('center_axis',(0.,0.,1.));
#30788=DIRECTION('ref_axis',(0.642787609686539,0.766044443118978,0.));
#30789=DIRECTION('center_axis',(0.,0.,-1.));
#30790=DIRECTION('ref_axis',(1.,0.,0.));
#30791=DIRECTION('',(-0.421534610602074,-0.906812313582341,0.));
#30792=DIRECTION('',(0.819837079988238,0.572596858423411,0.));
#30793=DIRECTION('center_axis',(0.572596858423411,-0.819837079988238,0.));
#30794=DIRECTION('ref_axis',(0.819837079988238,0.572596858423411,0.));
#30795=DIRECTION('',(0.,0.,1.));
#30796=DIRECTION('',(0.,0.,1.));
#30797=DIRECTION('center_axis',(-0.906812313582341,0.421534610602074,0.));
#30798=DIRECTION('ref_axis',(-0.421534610602074,-0.906812313582341,0.));
#30799=DIRECTION('',(0.,0.,-1.));
#30800=DIRECTION('center_axis',(0.,0.,1.));
#30801=DIRECTION('ref_axis',(0.766044443118978,0.642787609686539,0.));
#30802=DIRECTION('center_axis',(0.,0.,-1.));
#30803=DIRECTION('ref_axis',(1.,0.,0.));
#30804=DIRECTION('',(-0.572596858423411,-0.819837079988238,0.));
#30805=DIRECTION('',(0.906812313582341,0.421534610602074,0.));
#30806=DIRECTION('center_axis',(0.421534610602074,-0.906812313582341,0.));
#30807=DIRECTION('ref_axis',(0.906812313582341,0.421534610602074,0.));
#30808=DIRECTION('',(0.,0.,1.));
#30809=DIRECTION('',(0.,0.,1.));
#30810=DIRECTION('center_axis',(-0.819837079988238,0.572596858423411,0.));
#30811=DIRECTION('ref_axis',(-0.572596858423411,-0.819837079988238,0.));
#30812=DIRECTION('',(0.,0.,-1.));
#30813=DIRECTION('center_axis',(0.,0.,1.));
#30814=DIRECTION('ref_axis',(0.866025403784439,0.5,0.));
#30815=DIRECTION('center_axis',(0.,0.,-1.));
#30816=DIRECTION('ref_axis',(1.,0.,0.));
#30817=DIRECTION('',(-0.706261040449544,-0.707951511576272,0.));
#30818=DIRECTION('',(0.966234513897416,0.257664246944398,0.));
#30819=DIRECTION('center_axis',(0.257664246944398,-0.966234513897416,0.));
#30820=DIRECTION('ref_axis',(0.966234513897416,0.257664246944398,0.));
#30821=DIRECTION('',(0.,0.,1.));
#30822=DIRECTION('',(0.,0.,1.));
#30823=DIRECTION('center_axis',(-0.707951511576272,0.706261040449544,0.));
#30824=DIRECTION('ref_axis',(-0.706261040449544,-0.707951511576272,0.));
#30825=DIRECTION('',(0.,0.,-1.));
#30826=DIRECTION('center_axis',(0.,0.,1.));
#30827=DIRECTION('ref_axis',(0.939692620785909,0.342020143325669,0.));
#30828=DIRECTION('center_axis',(0.,0.,-1.));
#30829=DIRECTION('ref_axis',(1.,0.,0.));
#30830=DIRECTION('',(-0.818465838146948,-0.574555194725811,0.));
#30831=DIRECTION('',(0.996298167445974,0.0859648855277167,0.));
#30832=DIRECTION('center_axis',(0.0859648855277167,-0.996298167445974,0.));
#30833=DIRECTION('ref_axis',(0.996298167445974,0.0859648855277167,0.));
#30834=DIRECTION('',(0.,0.,1.));
#30835=DIRECTION('',(0.,0.,1.));
#30836=DIRECTION('center_axis',(-0.574555194725811,0.818465838146948,0.));
#30837=DIRECTION('ref_axis',(-0.818465838146948,-0.574555194725811,0.));
#30838=DIRECTION('',(0.,0.,-1.));
#30839=DIRECTION('center_axis',(0.,0.,1.));
#30840=DIRECTION('ref_axis',(0.984807753012208,0.17364817766693,0.));
#30841=DIRECTION('center_axis',(0.,0.,-1.));
#30842=DIRECTION('ref_axis',(1.,0.,0.));
#30843=DIRECTION('',(-0.905801965515955,-0.423701309022563,0.));
#30844=DIRECTION('',(0.996089805327885,-0.0883464754353932,0.));
#30845=DIRECTION('center_axis',(-0.0883464754353933,-0.996089805327885,
0.));
#30846=DIRECTION('ref_axis',(0.996089805327885,-0.0883464754353933,0.));
#30847=DIRECTION('',(0.,0.,1.));
#30848=DIRECTION('',(0.,0.,1.));
#30849=DIRECTION('center_axis',(-0.423701309022563,0.905801965515955,0.));
#30850=DIRECTION('ref_axis',(-0.905801965515954,-0.423701309022563,0.));
#30851=DIRECTION('',(0.,0.,-1.));
#30852=DIRECTION('center_axis',(0.,0.,1.));
#30853=DIRECTION('ref_axis',(1.,0.,0.));
#30854=DIRECTION('center_axis',(0.,0.,1.));
#30855=DIRECTION('ref_axis',(1.,0.,0.));
#30856=DIRECTION('center_axis',(0.,0.,1.));
#30857=DIRECTION('ref_axis',(1.,0.,0.));
#30858=DIRECTION('center_axis',(0.,0.,1.));
#30859=DIRECTION('ref_axis',(1.,0.,0.));
#30860=DIRECTION('center_axis',(0.,0.,1.));
#30861=DIRECTION('ref_axis',(1.,0.,0.));
#30862=DIRECTION('center_axis',(0.,0.,1.));
#30863=DIRECTION('ref_axis',(1.,0.,0.));
#30864=DIRECTION('center_axis',(0.,0.,1.));
#30865=DIRECTION('ref_axis',(1.,0.,0.));
#30866=DIRECTION('center_axis',(0.,0.,1.));
#30867=DIRECTION('ref_axis',(1.,0.,0.));
#30868=DIRECTION('center_axis',(0.,0.,1.));
#30869=DIRECTION('ref_axis',(1.,0.,0.));
#30870=DIRECTION('center_axis',(0.,0.,1.));
#30871=DIRECTION('ref_axis',(1.,0.,0.));
#30872=DIRECTION('center_axis',(0.,0.,1.));
#30873=DIRECTION('ref_axis',(1.,0.,0.));
#30874=DIRECTION('center_axis',(0.,0.,1.));
#30875=DIRECTION('ref_axis',(1.,0.,0.));
#30876=DIRECTION('center_axis',(0.,0.,1.));
#30877=DIRECTION('ref_axis',(1.,0.,0.));
#30878=DIRECTION('center_axis',(0.,0.,1.));
#30879=DIRECTION('ref_axis',(1.,0.,0.));
#30880=DIRECTION('center_axis',(0.,0.,1.));
#30881=DIRECTION('ref_axis',(1.,0.,0.));
#30882=DIRECTION('center_axis',(0.,0.,1.));
#30883=DIRECTION('ref_axis',(1.,0.,0.));
#30884=DIRECTION('center_axis',(0.,0.,1.));
#30885=DIRECTION('ref_axis',(1.,0.,0.));
#30886=DIRECTION('center_axis',(0.,0.,1.));
#30887=DIRECTION('ref_axis',(1.,0.,0.));
#30888=DIRECTION('',(0.,0.,-1.));
#30889=DIRECTION('center_axis',(0.,0.,1.));
#30890=DIRECTION('ref_axis',(1.,0.,0.));
#30891=DIRECTION('center_axis',(0.,0.,1.));
#30892=DIRECTION('ref_axis',(1.,0.,0.));
#30893=DIRECTION('center_axis',(0.,0.,1.));
#30894=DIRECTION('ref_axis',(1.,0.,0.));
#30895=DIRECTION('center_axis',(0.,0.,1.));
#30896=DIRECTION('ref_axis',(1.,0.,0.));
#30897=DIRECTION('center_axis',(0.,0.,1.));
#30898=DIRECTION('ref_axis',(1.,0.,0.));
#30899=DIRECTION('center_axis',(0.,0.,1.));
#30900=DIRECTION('ref_axis',(1.,0.,0.));
#30901=DIRECTION('center_axis',(0.,0.,1.));
#30902=DIRECTION('ref_axis',(1.,0.,0.));
#30903=DIRECTION('center_axis',(0.,0.,1.));
#30904=DIRECTION('ref_axis',(1.,0.,0.));
#30905=DIRECTION('center_axis',(0.,0.,1.));
#30906=DIRECTION('ref_axis',(1.,0.,0.));
#30907=DIRECTION('center_axis',(0.,0.,1.));
#30908=DIRECTION('ref_axis',(1.,0.,0.));
#30909=DIRECTION('center_axis',(0.,0.,1.));
#30910=DIRECTION('ref_axis',(1.,0.,0.));
#30911=DIRECTION('center_axis',(0.,0.,1.));
#30912=DIRECTION('ref_axis',(1.,0.,0.));
#30913=DIRECTION('center_axis',(0.,0.,1.));
#30914=DIRECTION('ref_axis',(1.,0.,0.));
#30915=DIRECTION('center_axis',(0.,0.,1.));
#30916=DIRECTION('ref_axis',(1.,0.,0.));
#30917=DIRECTION('center_axis',(0.,0.,1.));
#30918=DIRECTION('ref_axis',(1.,0.,0.));
#30919=DIRECTION('center_axis',(0.,0.,1.));
#30920=DIRECTION('ref_axis',(1.,0.,0.));
#30921=DIRECTION('center_axis',(0.,0.,1.));
#30922=DIRECTION('ref_axis',(1.,0.,0.));
#30923=DIRECTION('center_axis',(0.,0.,1.));
#30924=DIRECTION('ref_axis',(1.,0.,0.));
#30925=DIRECTION('center_axis',(0.,0.,1.));
#30926=DIRECTION('ref_axis',(1.,0.,0.));
#30927=DIRECTION('',(0.,0.,-1.));
#30928=DIRECTION('center_axis',(0.,0.,-1.));
#30929=DIRECTION('ref_axis',(1.,0.,0.));
#30930=DIRECTION('',(0.,0.,1.));
#30931=DIRECTION('center_axis',(0.,0.,1.));
#30932=DIRECTION('ref_axis',(1.,0.,0.));
#30933=DIRECTION('center_axis',(-0.259973473447872,-0.96561575852067,0.));
#30934=DIRECTION('ref_axis',(0.96561575852067,-0.259973473447872,0.));
#30935=DIRECTION('',(0.96561575852067,-0.259973473447872,0.));
#30936=DIRECTION('',(0.,0.,1.));
#30937=DIRECTION('center_axis',(-0.259973473447872,0.96561575852067,0.));
#30938=DIRECTION('ref_axis',(-0.96561575852067,-0.259973473447872,0.));
#30939=DIRECTION('',(-0.96561575852067,-0.259973473447872,0.));
#30940=DIRECTION('center_axis',(0.,0.,1.));
#30941=DIRECTION('ref_axis',(1.,0.,0.));
#30942=DIRECTION('center_axis',(0.,0.,-1.));
#30943=DIRECTION('ref_axis',(1.,0.,0.));
#30944=DIRECTION('center_axis',(0.,0.,1.));
#30945=DIRECTION('ref_axis',(1.,0.,0.));
#30946=DIRECTION('',(-0.707106781186549,-8.65956056235495E-17,-0.707106781186546));
#30947=DIRECTION('center_axis',(0.,0.,1.));
#30948=DIRECTION('ref_axis',(1.,0.,0.));
#30949=DIRECTION('',(-0.844694227521705,-1.0344520819927E-16,0.535249158795705));
#30950=DIRECTION('center_axis',(0.,0.,-1.));
#30951=DIRECTION('ref_axis',(1.,0.,0.));
#30952=DIRECTION('center_axis',(0.5,0.866025403784439,0.));
#30953=DIRECTION('ref_axis',(0.866025403784439,-0.5,0.));
#30954=DIRECTION('',(0.866025403784439,-0.5,0.));
#30955=DIRECTION('',(0.,0.,-1.));
#30956=DIRECTION('',(0.866025403784439,-0.5,0.));
#30957=DIRECTION('',(0.,0.,-1.));
#30958=DIRECTION('center_axis',(-0.5,0.866025403784439,0.));
#30959=DIRECTION('ref_axis',(0.866025403784439,0.5,0.));
#30960=DIRECTION('',(0.866025403784439,0.5,0.));
#30961=DIRECTION('',(0.,0.,-1.));
#30962=DIRECTION('',(0.866025403784439,0.5,0.));
#30963=DIRECTION('center_axis',(-1.,-1.92296268638356E-16,0.));
#30964=DIRECTION('ref_axis',(-1.92296268638356E-16,1.,0.));
#30965=DIRECTION('',(-1.92296268638356E-16,1.,0.));
#30966=DIRECTION('',(0.,0.,-1.));
#30967=DIRECTION('',(-1.92296268638356E-16,1.,0.));
#30968=DIRECTION('center_axis',(-0.5,-0.866025403784439,0.));
#30969=DIRECTION('ref_axis',(-0.866025403784439,0.5,0.));
#30970=DIRECTION('',(-0.866025403784439,0.5,0.));
#30971=DIRECTION('',(0.,0.,-1.));
#30972=DIRECTION('',(-0.866025403784439,0.5,0.));
#30973=DIRECTION('center_axis',(0.5,-0.866025403784439,0.));
#30974=DIRECTION('ref_axis',(-0.866025403784439,-0.5,0.));
#30975=DIRECTION('',(-0.866025403784439,-0.5,0.));
#30976=DIRECTION('',(0.,0.,-1.));
#30977=DIRECTION('',(-0.866025403784439,-0.5,0.));
#30978=DIRECTION('center_axis',(1.,-3.84592537276713E-16,0.));
#30979=DIRECTION('ref_axis',(-3.84592537276713E-16,-1.,0.));
#30980=DIRECTION('',(-3.84592537276713E-16,-1.,0.));
#30981=DIRECTION('',(-3.84592537276713E-16,-1.,0.));
#30982=DIRECTION('center_axis',(0.,0.,-1.));
#30983=DIRECTION('ref_axis',(-1.,0.,0.));
#30984=DIRECTION('center_axis',(0.,0.,-1.));
#30985=DIRECTION('ref_axis',(-1.,0.,0.));
#30986=DIRECTION('center_axis',(0.,0.,1.));
#30987=DIRECTION('ref_axis',(1.,0.,0.));
#30988=DIRECTION('center_axis',(0.,0.,1.));
#30989=DIRECTION('ref_axis',(1.,0.,0.));
#30990=DIRECTION('',(0.707106781186547,8.65956056235493E-17,-0.707106781186548));
#30991=DIRECTION('center_axis',(0.,0.,1.));
#30992=DIRECTION('ref_axis',(0.952238475886209,-0.30535534225212,0.));
#30993=DIRECTION('center_axis',(0.,0.,1.));
#30994=DIRECTION('ref_axis',(1.,0.,0.));
#30995=DIRECTION('center_axis',(0.,0.,1.));
#30996=DIRECTION('ref_axis',(1.,0.,0.));
#30997=DIRECTION('center_axis',(0.,0.,1.));
#30998=DIRECTION('ref_axis',(1.,0.,0.));
#30999=DIRECTION('',(0.707106781186548,8.65956056235494E-17,-0.707106781186547));
#31000=DIRECTION('center_axis',(0.,0.,-1.));
#31001=DIRECTION('ref_axis',(-1.,0.,0.));
#31002=DIRECTION('center_axis',(0.,0.,1.));
#31003=DIRECTION('ref_axis',(1.,0.,0.));
#41661=CARTESIAN_POINT('',(0.,0.,0.));
#41662=CARTESIAN_POINT('Origin',(0.,0.,-1.487));
#41663=CARTESIAN_POINT('',(-0.146158606821014,-8.60648302992845E-5,-2.90158449541571));
#41664=CARTESIAN_POINT('',(-0.146182739311418,-0.000106450303776882,-2.90871550458429));
#41665=CARTESIAN_POINT('',(-0.14635,-1.79227059055215E-17,-1.487));
#41666=CARTESIAN_POINT('',(0.0262268935511073,-0.144224038131951,-2.93765));
#41667=CARTESIAN_POINT('Ctrl Pts',(-0.146158606821014,-8.60648302992845E-5,
-2.90158449541571));
#41668=CARTESIAN_POINT('Ctrl Pts',(-0.145999351227507,0.0299154702969904,
-2.90321100897527));
#41669=CARTESIAN_POINT('Ctrl Pts',(-0.137018833441673,0.0600042754394542,
-2.90483752253483));
#41670=CARTESIAN_POINT('Ctrl Pts',(-0.119884214267969,0.0843568428068597,
-2.90646403609438));
#41671=CARTESIAN_POINT('Ctrl Pts',(-0.0919771182949038,0.124019786454636,
-2.90911313319704));
#41672=CARTESIAN_POINT('Ctrl Pts',(-0.0424400239805762,0.148466483988013,
-2.91176223029968));
#41673=CARTESIAN_POINT('Ctrl Pts',(0.00601684655231771,0.146471621494668,
-2.91441132740233));
#41674=CARTESIAN_POINT('Ctrl Pts',(0.0544737170852115,0.144476759001322,
-2.91706042450498));
#41675=CARTESIAN_POINT('Ctrl Pts',(0.101850363836672,0.116040336481254,
-2.91970952160764));
#41676=CARTESIAN_POINT('Ctrl Pts',(0.126406665804976,0.0742301586072307,
-2.92235861871029));
#41677=CARTESIAN_POINT('Ctrl Pts',(0.150962967773281,0.0324199807332077,
-2.92500771581294));
#41678=CARTESIAN_POINT('Ctrl Pts',(0.15269892495843,-0.02276395249477,-2.92765681291559));
#41679=CARTESIAN_POINT('Ctrl Pts',(0.130844409959043,-0.0660664516720163,
-2.93030591001824));
#41680=CARTESIAN_POINT('Ctrl Pts',(0.110648657916751,-0.106082280722433,
-2.93275394001216));
#41681=CARTESIAN_POINT('Ctrl Pts',(0.0703075776504436,-0.135951836020819,
-2.93520197000608));
#41682=CARTESIAN_POINT('Ctrl Pts',(0.0262268935511073,-0.144224038131951,
-2.93765));
#41683=CARTESIAN_POINT('',(-0.14635,-1.79227059055215E-17,-2.93765));
#41684=CARTESIAN_POINT('Origin',(0.,0.,-2.93765));
#41685=CARTESIAN_POINT('',(-0.14635,-1.79227059055215E-17,-2.96765));
#41686=CARTESIAN_POINT('',(-0.14635,-1.79227059055215E-17,-1.487));
#41687=CARTESIAN_POINT('Origin',(0.,0.,-2.96765));
#41688=CARTESIAN_POINT('',(0.128823493644022,-0.0694465980833372,-2.93765));
#41689=CARTESIAN_POINT('Origin',(0.,0.,-2.93765));
#41690=CARTESIAN_POINT('Ctrl Pts',(0.128823493644022,-0.069446598083337,
-2.93765));
#41691=CARTESIAN_POINT('Ctrl Pts',(0.151941943903563,-0.0265618548091487,
-2.93500090289735));
#41692=CARTESIAN_POINT('Ctrl Pts',(0.151761457505771,0.0284019287429394,
-2.9323518057947));
#41693=CARTESIAN_POINT('Ctrl Pts',(0.128356941858912,0.0707835761050192,
-2.92970270869205));
#41694=CARTESIAN_POINT('Ctrl Pts',(0.104952426212054,0.113165223467099,
-2.9270536115894));
#41695=CARTESIAN_POINT('Ctrl Pts',(0.0583238813161294,0.142964734639171,
-2.92440451448675));
#41696=CARTESIAN_POINT('Ctrl Pts',(0.00992989165371453,0.146282598160944,
-2.9217554173841));
#41697=CARTESIAN_POINT('Ctrl Pts',(-0.0384640980087004,0.149600461682717,
-2.91910632028145));
#41698=CARTESIAN_POINT('Ctrl Pts',(-0.088623532437606,0.126436677554191,
-2.9164572231788));
#41699=CARTESIAN_POINT('Ctrl Pts',(-0.11757903185869,0.0875226022274051,
-2.91380812607615));
#41700=CARTESIAN_POINT('Ctrl Pts',(-0.136133705765244,0.0625864763618698,
-2.91211058557886));
#41701=CARTESIAN_POINT('Ctrl Pts',(-0.145981530992649,0.0311828998997731,
-2.91041304508157));
#41702=CARTESIAN_POINT('Ctrl Pts',(-0.146182739311418,-0.000106450303776882,
-2.90871550458429));
#41703=CARTESIAN_POINT('Origin',(0.,0.,-1.487));
#41704=CARTESIAN_POINT('',(-0.146537174558168,-7.96020625374039E-5,-2.85158449541571));
#41705=CARTESIAN_POINT('',(-0.146561971875871,-5.90665209240155E-5,-2.85871550458428));
#41706=CARTESIAN_POINT('',(-0.14635,-1.79227059055215E-17,-1.487));
#41707=CARTESIAN_POINT('Ctrl Pts',(-0.146537174558168,-7.96020625374039E-5,
-2.85158449541571));
#41708=CARTESIAN_POINT('Ctrl Pts',(-0.146249092612562,0.0438734690207087,
-2.85398309302603));
#41709=CARTESIAN_POINT('Ctrl Pts',(-0.125145271349427,0.0880663097270068,
-2.85638169063635));
#41710=CARTESIAN_POINT('Ctrl Pts',(-0.0906335957691385,0.115214904500943,
-2.85878028824667));
#41711=CARTESIAN_POINT('Ctrl Pts',(-0.0525176652796136,0.145198784851356,
-2.86142938534933));
#41712=CARTESIAN_POINT('Ctrl Pts',(0.00195287717864085,0.154392461047573,
-2.86407848245198));
#41713=CARTESIAN_POINT('Ctrl Pts',(0.0477983995988501,0.138579477442402,
-2.86672757955463));
#41714=CARTESIAN_POINT('Ctrl Pts',(0.0936439220190594,0.122766493837231,
-2.86937667665728));
#41715=CARTESIAN_POINT('Ctrl Pts',(0.130864424401223,0.0819468504306727,
-2.87202577375993));
#41716=CARTESIAN_POINT('Ctrl Pts',(0.142390573434243,0.0348407087048676,
-2.87467487086258));
#41717=CARTESIAN_POINT('Ctrl Pts',(0.153916722467262,-0.0122654330209376,
-2.87732396796523));
#41718=CARTESIAN_POINT('Ctrl Pts',(0.139748518151136,-0.0656580730659899,
-2.87997306506788));
#41719=CARTESIAN_POINT('Ctrl Pts',(0.106383941342532,-0.10085284189918,
-2.88262216217053));
#41720=CARTESIAN_POINT('Ctrl Pts',(0.0730193645339283,-0.13604761073237,
-2.88527125927318));
#41721=CARTESIAN_POINT('Ctrl Pts',(0.0204584152328461,-0.153044508353697,
-2.88792035637583));
#41722=CARTESIAN_POINT('Ctrl Pts',(-0.027195887990429,-0.144046802896069,
-2.89056945347848));
#41723=CARTESIAN_POINT('Ctrl Pts',(-0.0748501912137042,-0.13504909743844,
-2.89321855058113));
#41724=CARTESIAN_POINT('Ctrl Pts',(-0.117597848359172,-0.100056788901855,
-2.89586764768378));
#41725=CARTESIAN_POINT('Ctrl Pts',(-0.135833128116005,-0.055121039752474,
-2.89851674478643));
#41726=CARTESIAN_POINT('Ctrl Pts',(-0.142872166799927,-0.0377752967328191,
-2.89953932832952));
#41727=CARTESIAN_POINT('Ctrl Pts',(-0.146258730271021,-0.0189479279290693,
-2.90056191187262));
#41728=CARTESIAN_POINT('Ctrl Pts',(-0.146158606821014,-8.60648302992845E-5,
-2.90158449541571));
#41729=CARTESIAN_POINT('Ctrl Pts',(-0.146182739311418,-0.000106450303776882,
-2.90871550458429));
#41730=CARTESIAN_POINT('Ctrl Pts',(-0.146295526667645,-0.0176457007141658,
-2.90776394797892));
#41731=CARTESIAN_POINT('Ctrl Pts',(-0.143377187945856,-0.0351490593508527,
-2.90681239137356));
#41732=CARTESIAN_POINT('Ctrl Pts',(-0.137262197911326,-0.0514572684605561,
-2.9058608347682));
#41733=CARTESIAN_POINT('Ctrl Pts',(-0.120238300129616,-0.0968586972966848,
-2.90321173766555));
#41734=CARTESIAN_POINT('Ctrl Pts',(-0.0784389401529336,-0.132997188443895,
-2.90056264056289));
#41735=CARTESIAN_POINT('Ctrl Pts',(-0.0310416975091987,-0.143270901492602,
-2.89791354346024));
#41736=CARTESIAN_POINT('Ctrl Pts',(0.0163555451345362,-0.153544614541308,
-2.89526444635759));
#41737=CARTESIAN_POINT('Ctrl Pts',(0.0693506704453232,-0.13795354949151,
-2.89261534925494));
#41738=CARTESIAN_POINT('Ctrl Pts',(0.103645083731081,-0.103662905171766,
-2.88996625215229));
#41739=CARTESIAN_POINT('Ctrl Pts',(0.137939497016838,-0.0693722608520209,
-2.88731715504964));
#41740=CARTESIAN_POINT('Ctrl Pts',(0.153533198277566,-0.0163820372623291,
-2.88466805794699));
#41741=CARTESIAN_POINT('Ctrl Pts',(0.143272624045871,0.0310148776620776,
-2.88201896084434));
#41742=CARTESIAN_POINT('Ctrl Pts',(0.133012049814177,0.0784117925864847,
-2.87936986374169));
#41743=CARTESIAN_POINT('Ctrl Pts',(0.0968972000900611,0.120215398845607,
-2.87672076663904));
#41744=CARTESIAN_POINT('Ctrl Pts',(0.0514913441008033,0.137250642800901,
-2.87407166953639));
#41745=CARTESIAN_POINT('Ctrl Pts',(0.0060854881115459,0.154285886756194,
-2.87142257243374));
#41746=CARTESIAN_POINT('Ctrl Pts',(-0.0486113741428529,0.14655276840766,
-2.86877347533109));
#41747=CARTESIAN_POINT('Ctrl Pts',(-0.087516338371486,0.117599867637059,
-2.86612437822844));
#41748=CARTESIAN_POINT('Ctrl Pts',(-0.123785546700601,0.0906084846451613,
-2.86365475368039));
#41749=CARTESIAN_POINT('Ctrl Pts',(-0.146330131439324,0.0451751432555005,
-2.86118512913233));
#41750=CARTESIAN_POINT('Ctrl Pts',(-0.146561971875871,-5.90665209240155E-5,
-2.85871550458428));
#41751=CARTESIAN_POINT('Origin',(0.,0.,-1.487));
#41752=CARTESIAN_POINT('',(-0.146403203488696,0.000129450652049418,-2.80158449541571));
#41753=CARTESIAN_POINT('',(-0.146363430029852,0.000133824904544822,-2.80871550458428));
#41754=CARTESIAN_POINT('',(-0.14635,-1.79227059055215E-17,-1.487));
#41755=CARTESIAN_POINT('Ctrl Pts',(-0.146403203488696,0.000129450652049418,
-2.80158449541571));
#41756=CARTESIAN_POINT('Ctrl Pts',(-0.146491477515772,0.00970999864112991,
-2.80210607997414));
#41757=CARTESIAN_POINT('Ctrl Pts',(-0.145631706000451,0.01927477608682,
-2.80262766453258));
#41758=CARTESIAN_POINT('Ctrl Pts',(-0.143766246362832,0.0286392135733044,
-2.80314924909101));
#41759=CARTESIAN_POINT('Ctrl Pts',(-0.134291687269365,0.0762006373391004,
-2.80579834619366));
#41760=CARTESIAN_POINT('Ctrl Pts',(-0.098874759612967,0.118594163677882,
-2.80844744329632));
#41761=CARTESIAN_POINT('Ctrl Pts',(-0.053757403740153,0.136378441311147,
-2.81109654039897));
#41762=CARTESIAN_POINT('Ctrl Pts',(-0.0086400478673393,0.154162718944412,
-2.81374563750162));
#41763=CARTESIAN_POINT('Ctrl Pts',(0.0461777362218906,0.147337747872162,
-2.81639473460426));
#41764=CARTESIAN_POINT('Ctrl Pts',(0.085556925217133,0.119033402370627,
-2.81904383170692));
#41765=CARTESIAN_POINT('Ctrl Pts',(0.124936114212376,0.0907290568690924,
-2.82169292880957));
#41766=CARTESIAN_POINT('Ctrl Pts',(0.148876708113631,0.0409453369382727,
-2.82434202591222));
#41767=CARTESIAN_POINT('Ctrl Pts',(0.146399723101655,-0.00748730274776978,
-2.82699112301487));
#41768=CARTESIAN_POINT('Ctrl Pts',(0.143922738089679,-0.0559199424338124,
-2.82964022011752));
#41769=CARTESIAN_POINT('Ctrl Pts',(0.115028174164472,-0.103001501875078,
-2.83228931722017));
#41770=CARTESIAN_POINT('Ctrl Pts',(0.0729668743621239,-0.127140752828838,
-2.83493841432282));
#41771=CARTESIAN_POINT('Ctrl Pts',(0.0309055745597762,-0.151280003782598,
-2.83758751142547));
#41772=CARTESIAN_POINT('Ctrl Pts',(-0.0243224611197121,-0.152476946248854,
-2.84023660852812));
#41773=CARTESIAN_POINT('Ctrl Pts',(-0.0673900900429651,-0.130182626839244,
-2.84288570563077));
#41774=CARTESIAN_POINT('Ctrl Pts',(-0.110457718966218,-0.107888307429635,
-2.84553480273342));
#41775=CARTESIAN_POINT('Ctrl Pts',(-0.141364941133235,-0.0621027261441617,
-2.84818389983607));
#41776=CARTESIAN_POINT('Ctrl Pts',(-0.145937892956347,-0.0138228932491204,
-2.85083299693872));
#41777=CARTESIAN_POINT('Ctrl Pts',(-0.146370312783083,-0.00925753638929341,
-2.85108349643105));
#41778=CARTESIAN_POINT('Ctrl Pts',(-0.146567260630468,-0.00466987679026642,
-2.85133399592338));
#41779=CARTESIAN_POINT('Ctrl Pts',(-0.146537174558168,-7.96020625374039E-5,
-2.85158449541571));
#41780=CARTESIAN_POINT('Ctrl Pts',(-0.146561971875871,-5.90665209240155E-5,
-2.85871550458428));
#41781=CARTESIAN_POINT('Ctrl Pts',(-0.146578820184024,-0.0033463270036002,
-2.85853603202968));
#41782=CARTESIAN_POINT('Ctrl Pts',(-0.146477829990726,-0.00663253582850726,
-2.85835655947508));
#41783=CARTESIAN_POINT('Ctrl Pts',(-0.14625570520285,-0.0099105386052108,
-2.85817708692048));
#41784=CARTESIAN_POINT('Ctrl Pts',(-0.142977041602714,-0.0582953608842119,
-2.85552798981783));
#41785=CARTESIAN_POINT('Ctrl Pts',(-0.113306648199574,-0.104892322249546,
-2.85287889271518));
#41786=CARTESIAN_POINT('Ctrl Pts',(-0.0708513314510232,-0.128331785211355,
-2.85022979561253));
#41787=CARTESIAN_POINT('Ctrl Pts',(-0.0283960147024727,-0.151771248173164,
-2.84758069850988));
#41788=CARTESIAN_POINT('Ctrl Pts',(0.0268442253914879,-0.152053212731447,
-2.84493160140723));
#41789=CARTESIAN_POINT('Ctrl Pts',(0.0695367248469116,-0.12904869809198,
-2.84228250430458));
#41790=CARTESIAN_POINT('Ctrl Pts',(0.112229224302335,-0.106044183452514,
-2.83963340720193));
#41791=CARTESIAN_POINT('Ctrl Pts',(0.142373983119222,-0.0597531896152975,
-2.83698431009928));
#41792=CARTESIAN_POINT('Ctrl Pts',(0.146146788437797,-0.011404249008567,
-2.83433521299663));
#41793=CARTESIAN_POINT('Ctrl Pts',(0.149919593756371,0.0369446915981632,
-2.83168611589398));
#41794=CARTESIAN_POINT('Ctrl Pts',(0.127320445576634,0.0873515789744077,
-2.82903701879133));
#41795=CARTESIAN_POINT('Ctrl Pts',(0.0887131716818962,0.116700100359139,
-2.82638792168868));
#41796=CARTESIAN_POINT('Ctrl Pts',(0.0501058977871583,0.14604862174387,
-2.82373882458603));
#41797=CARTESIAN_POINT('Ctrl Pts',(-0.00450950182258007,0.154338777137088,
-2.82108972748338));
#41798=CARTESIAN_POINT('Ctrl Pts',(-0.0500868268902308,0.137768810843643,
-2.81844063038073));
#41799=CARTESIAN_POINT('Ctrl Pts',(-0.0956641519578814,0.121198844550198,
-2.81579153327808));
#41800=CARTESIAN_POINT('Ctrl Pts',(-0.132203402483444,0.0797687565700892,
-2.81314243617543));
#41801=CARTESIAN_POINT('Ctrl Pts',(-0.142947943413378,0.0324780508505072,
-2.81049333907278));
#41802=CARTESIAN_POINT('Ctrl Pts',(-0.145351531590539,0.0218989687009335,
-2.80990072757661));
#41803=CARTESIAN_POINT('Ctrl Pts',(-0.146464271988682,0.0110266029474243,
-2.80930811608045));
#41804=CARTESIAN_POINT('Ctrl Pts',(-0.146363430029852,0.000133824904544822,
-2.80871550458428));
#41805=CARTESIAN_POINT('Origin',(0.,0.,-1.487));
#41806=CARTESIAN_POINT('',(-0.146109113220983,9.39517128401013E-6,-2.75158449541571));
#41807=CARTESIAN_POINT('',(-0.146109487156769,-1.22079509434409E-5,-2.75871550458428));
#41808=CARTESIAN_POINT('',(-0.14635,-1.79227059055215E-17,-1.487));
#41809=CARTESIAN_POINT('Ctrl Pts',(-0.146109113220983,9.39517128401013E-6,
-2.75158449541571));
#41810=CARTESIAN_POINT('Ctrl Pts',(-0.146122761734058,0.0238929355757029,
-2.75287816402491));
#41811=CARTESIAN_POINT('Ctrl Pts',(-0.140597949611965,0.047770526414132,
-2.7541718326341));
#41812=CARTESIAN_POINT('Ctrl Pts',(-0.129500331978527,0.0686920815018531,
-2.7554655012433));
#41813=CARTESIAN_POINT('Ctrl Pts',(-0.106775295203236,0.111533989059758,
-2.75811459834595));
#41814=CARTESIAN_POINT('Ctrl Pts',(-0.0606821498632086,0.141980530548785,
-2.7607636954486));
#41815=CARTESIAN_POINT('Ctrl Pts',(-0.0123588683584905,0.146069149401598,
-2.76341279255126));
#41816=CARTESIAN_POINT('Ctrl Pts',(0.0359644131462274,0.150157768254412,
-2.76606188965391));
#41817=CARTESIAN_POINT('Ctrl Pts',(0.0865178308156365,0.127888464471012,
-2.76871098675656));
#41818=CARTESIAN_POINT('Ctrl Pts',(0.116117964761986,0.0894737743849098,
-2.77136008385921));
#41819=CARTESIAN_POINT('Ctrl Pts',(0.145718098708336,0.0510590842988072,
-2.77400918096186));
#41820=CARTESIAN_POINT('Ctrl Pts',(0.154364948931627,-0.00350099208999865,
-2.77665827806451));
#41821=CARTESIAN_POINT('Ctrl Pts',(0.138093134336948,-0.0491856107813916,
-2.77930737516716));
#41822=CARTESIAN_POINT('Ctrl Pts',(0.121821319742268,-0.0948702294727843,
-2.78195647226981));
#41823=CARTESIAN_POINT('Ctrl Pts',(0.0806308403296187,-0.131679390466764,
-2.78460556937246));
#41824=CARTESIAN_POINT('Ctrl Pts',(0.0334113427175706,-0.142732687816649,
-2.78725466647511));
#41825=CARTESIAN_POINT('Ctrl Pts',(-0.0138081548944779,-0.153785985166534,
-2.78990376357776));
#41826=CARTESIAN_POINT('Ctrl Pts',(-0.0670566707059247,-0.139083418872324,
-2.79255286068041));
#41827=CARTESIAN_POINT('Ctrl Pts',(-0.10191483334638,-0.105367475128813,
-2.79520195778306));
#41828=CARTESIAN_POINT('Ctrl Pts',(-0.129909721948874,-0.0782899122932978,
-2.79732947032728));
#41829=CARTESIAN_POINT('Ctrl Pts',(-0.146043138956694,-0.0389490375769943,
-2.79945698287149));
#41830=CARTESIAN_POINT('Ctrl Pts',(-0.146403203488696,0.000129450652049418,
-2.80158449541571));
#41831=CARTESIAN_POINT('Ctrl Pts',(-0.146363430029852,0.000133824904544822,
-2.80871550458428));
#41832=CARTESIAN_POINT('Ctrl Pts',(-0.146013487380734,-0.0376663889030354,
-2.8066590189778));
#41833=CARTESIAN_POINT('Ctrl Pts',(-0.131049162627967,-0.075712414620085,
-2.80460253337131));
#41834=CARTESIAN_POINT('Ctrl Pts',(-0.104699336383414,-0.102601106132693,
-2.80254604776482));
#41835=CARTESIAN_POINT('Ctrl Pts',(-0.070756357089213,-0.137238233937254,
-2.79989695066217));
#41836=CARTESIAN_POINT('Ctrl Pts',(-0.0179205671665077,-0.153361166087323,
-2.79724785355952));
#41837=CARTESIAN_POINT('Ctrl Pts',(0.0295779366406567,-0.143576053231004,
-2.79459875645687));
#41838=CARTESIAN_POINT('Ctrl Pts',(0.0770764404478212,-0.133790940374685,
-2.79194965935422));
#41839=CARTESIAN_POINT('Ctrl Pts',(0.119237658139444,-0.0980977825119792,
-2.78930056225157));
#41840=CARTESIAN_POINT('Ctrl Pts',(0.136726768918096,-0.0528651917123114,
-2.78665146514892));
#41841=CARTESIAN_POINT('Ctrl Pts',(0.154215879696748,-0.00763260091264373,
-2.78400236804627));
#41842=CARTESIAN_POINT('Ctrl Pts',(0.147032883562428,0.0471394228239861,
-2.78135327094362));
#41843=CARTESIAN_POINT('Ctrl Pts',(0.118471849500886,0.0863328363546023,
-2.77870417384097));
#41844=CARTESIAN_POINT('Ctrl Pts',(0.0899108154393433,0.125526249885218,
-2.77605507673832));
#41845=CARTESIAN_POINT('Ctrl Pts',(0.0399717434505784,0.149141053209821,
-2.77340597963567));
#41846=CARTESIAN_POINT('Ctrl Pts',(-0.00844368115681214,0.146347674830144,
-2.77075688253302));
#41847=CARTESIAN_POINT('Ctrl Pts',(-0.056859105764203,0.143554296450466,
-2.76810778543037));
#41848=CARTESIAN_POINT('Ctrl Pts',(-0.103750882990219,0.114352736366508,
-2.76545868832772));
#41849=CARTESIAN_POINT('Ctrl Pts',(-0.127614793689341,0.0721346115032102,
-2.76280959122507));
#41850=CARTESIAN_POINT('Ctrl Pts',(-0.13990840596606,0.0503857345205872,
-2.76144489567814));
#41851=CARTESIAN_POINT('Ctrl Pts',(-0.146090776026834,0.0251824610964542,
-2.76008020013121));
#41852=CARTESIAN_POINT('Ctrl Pts',(-0.146109487156769,-1.22079509434409E-5,
-2.75871550458428));
#41853=CARTESIAN_POINT('Origin',(0.,0.,-1.487));
#41854=CARTESIAN_POINT('',(-0.146368629392587,-0.000133465523585494,-2.70158449541571));
#41855=CARTESIAN_POINT('',(-0.146408351835359,-0.000128600226034899,-2.70871550458428));
#41856=CARTESIAN_POINT('',(-0.14635,-1.79227059055215E-17,-1.487));
#41857=CARTESIAN_POINT('Ctrl Pts',(-0.146368629392587,-0.000133465523585494,
-2.70158449541571));
#41858=CARTESIAN_POINT('Ctrl Pts',(-0.14601683807807,0.0378336302900692,
-2.70365024807567));
#41859=CARTESIAN_POINT('Ctrl Pts',(-0.13090301761128,0.0760490326861501,
-2.70571600073563));
#41860=CARTESIAN_POINT('Ctrl Pts',(-0.104340252656597,0.102966255230573,
-2.7077817533956));
#41861=CARTESIAN_POINT('Ctrl Pts',(-0.0702764728809716,0.137484587282563,
-2.71043085049825));
#41862=CARTESIAN_POINT('Ctrl Pts',(-0.017384676891153,0.153422838553933,
-2.71307994760089));
#41863=CARTESIAN_POINT('Ctrl Pts',(0.0300793525132317,0.143471845993703,
-2.71572904470354));
#41864=CARTESIAN_POINT('Ctrl Pts',(0.0775433819176172,0.133520853433473,
-2.71837814180619));
#41865=CARTESIAN_POINT('Ctrl Pts',(0.119579644736569,0.0976806170416416,
-2.72102723890885));
#41866=CARTESIAN_POINT('Ctrl Pts',(0.136910624647343,0.0523872016738897,
-2.7236763360115));
#41867=CARTESIAN_POINT('Ctrl Pts',(0.154241604558118,0.00709378630613784,
-2.72632543311415));
#41868=CARTESIAN_POINT('Ctrl Pts',(0.146867301560715,-0.0476528080375341,
-2.7289745302168));
#41869=CARTESIAN_POINT('Ctrl Pts',(0.118169515957076,-0.0867462018737963,
-2.73162362731945));
#41870=CARTESIAN_POINT('Ctrl Pts',(0.0894717303534362,-0.125839595710059,
-2.7342727244221));
#41871=CARTESIAN_POINT('Ctrl Pts',(0.0394504621435592,-0.149279789038911,
-2.73692182152475));
#41872=CARTESIAN_POINT('Ctrl Pts',(-0.00895490847948087,-0.146317284193646,
-2.7395709186274));
#41873=CARTESIAN_POINT('Ctrl Pts',(-0.0573602791025203,-0.143354779348381,
-2.74222001573005));
#41874=CARTESIAN_POINT('Ctrl Pts',(-0.104149752138723,-0.113989576329,-2.7448691128327));
#41875=CARTESIAN_POINT('Ctrl Pts',(-0.127866024551547,-0.0716883380059181,
-2.74751820993535));
#41876=CARTESIAN_POINT('Ctrl Pts',(-0.140000616127923,-0.0500446226154691,
-2.7488736384288));
#41877=CARTESIAN_POINT('Ctrl Pts',(-0.146094813126366,-0.0250143481262689,
-2.75022906692226));
#41878=CARTESIAN_POINT('Ctrl Pts',(-0.146109113220983,9.39517128401013E-6,
-2.75158449541571));
#41879=CARTESIAN_POINT('Ctrl Pts',(-0.146109487156769,-1.22079509434409E-5,
-2.75871550458428));
#41880=CARTESIAN_POINT('Ctrl Pts',(-0.146127097388187,-0.0237245093453919,
-2.75743110302856));
#41881=CARTESIAN_POINT('Ctrl Pts',(-0.140685008674315,-0.0474291890808367,
-2.75614670147284));
#41882=CARTESIAN_POINT('Ctrl Pts',(-0.129739522674641,-0.0682392408035371,
-2.75486229991711));
#41883=CARTESIAN_POINT('Ctrl Pts',(-0.107164296788595,-0.11116027860435,
-2.75221320281446));
#41884=CARTESIAN_POINT('Ctrl Pts',(-0.0611778008442754,-0.14176766456334,
-2.74956410571181));
#41885=CARTESIAN_POINT('Ctrl Pts',(-0.0128690985436487,-0.14602508011577,
-2.74691500860916));
#41886=CARTESIAN_POINT('Ctrl Pts',(0.035439603756978,-0.150282495668201,
-2.74426591150651));
#41887=CARTESIAN_POINT('Ctrl Pts',(0.0860705124139122,-0.128189940814073,
-2.74161681440386));
#41888=CARTESIAN_POINT('Ctrl Pts',(0.115804670657886,-0.0898788962079824,
-2.73896771730121));
#41889=CARTESIAN_POINT('Ctrl Pts',(0.145538828901859,-0.0515678516018915,
-2.73631862019856));
#41890=CARTESIAN_POINT('Ctrl Pts',(0.154376236732872,0.00296168275616224,
-2.73366952309591));
#41891=CARTESIAN_POINT('Ctrl Pts',(0.138264124904087,0.0487028694361347,
-2.73102042599326));
#41892=CARTESIAN_POINT('Ctrl Pts',(0.122152013075302,0.0944440561161064,
-2.72837132889061));
#41893=CARTESIAN_POINT('Ctrl Pts',(0.081090381586721,0.131396895117997,
-2.72572223178796));
#41894=CARTESIAN_POINT('Ctrl Pts',(0.0339097881036398,0.142615090353666,
-2.72307313468531));
#41895=CARTESIAN_POINT('Ctrl Pts',(-0.0132708053794418,0.153833285589334,
-2.72042403758266));
#41896=CARTESIAN_POINT('Ctrl Pts',(-0.0665703608570236,0.13931683705878,
-2.71777494048001));
#41897=CARTESIAN_POINT('Ctrl Pts',(-0.10154610006969,0.105722879680012,
-2.71512584337736));
#41898=CARTESIAN_POINT('Ctrl Pts',(-0.129757767316244,0.0786257669842071,
-2.71298906377966));
#41899=CARTESIAN_POINT('Ctrl Pts',(-0.146047695012257,0.0391165514560332,
-2.71085228418197));
#41900=CARTESIAN_POINT('Ctrl Pts',(-0.146408351835359,-0.0001286002260349,
-2.70871550458428));
#41901=CARTESIAN_POINT('Origin',(0.,0.,-1.487));
#41902=CARTESIAN_POINT('',(-0.146559056518854,6.20051383258494E-5,-2.65158449541571));
#41903=CARTESIAN_POINT('',(-0.146533501836025,8.20954179803956E-5,-2.65871550458428));
#41904=CARTESIAN_POINT('',(-0.14635,-1.79227059055215E-17,-1.487));
#41905=CARTESIAN_POINT('Ctrl Pts',(-0.146559056518854,6.20051383258494E-5,
-2.65158449541571));
#41906=CARTESIAN_POINT('Ctrl Pts',(-0.146577480383996,0.00351919868299243,
-2.65177323502378));
#41907=CARTESIAN_POINT('Ctrl Pts',(-0.146465774681179,0.00697518102620523,
-2.65196197463186));
#41908=CARTESIAN_POINT('Ctrl Pts',(-0.146220135174594,0.0104216174415365,
-2.65215071423993));
#41909=CARTESIAN_POINT('Ctrl Pts',(-0.142772406783976,0.0587948487705055,
-2.65479981134258));
#41910=CARTESIAN_POINT('Ctrl Pts',(-0.112939510581635,0.10528751744827,
-2.65744890844523));
#41911=CARTESIAN_POINT('Ctrl Pts',(-0.0704025900606613,0.128578432691205,
-2.66009800554788));
#41912=CARTESIAN_POINT('Ctrl Pts',(-0.027865669539689,0.15186934793414,
-2.66274710265053));
#41913=CARTESIAN_POINT('Ctrl Pts',(0.027375275299915,0.151958509742246,
-2.66539619975318));
#41914=CARTESIAN_POINT('Ctrl Pts',(0.0699871595333896,0.128805029175963,
-2.66804529685583));
#41915=CARTESIAN_POINT('Ctrl Pts',(0.112599043766865,0.105651548609678,
-2.67069439395849));
#41916=CARTESIAN_POINT('Ctrl Pts',(0.142581867394211,0.0592554256690021,
-2.67334349106114));
#41917=CARTESIAN_POINT('Ctrl Pts',(0.146185731324473,0.0108935759831704,
-2.67599258816379));
#41918=CARTESIAN_POINT('Ctrl Pts',(0.149789595254736,-0.0374682737026606,
-2.67864168526644));
#41919=CARTESIAN_POINT('Ctrl Pts',(0.127014499487917,-0.087795850133647,
-2.68129078236909));
#41920=CARTESIAN_POINT('Ctrl Pts',(0.0883049329244487,-0.117009302458371,
-2.68393987947174));
#41921=CARTESIAN_POINT('Ctrl Pts',(0.0495953663609803,-0.146222754783096,
-2.68658897657439));
#41922=CARTESIAN_POINT('Ctrl Pts',(-0.00504867099913701,-0.154322083001559,
-2.68923807367704));
#41923=CARTESIAN_POINT('Ctrl Pts',(-0.0505678315451675,-0.137592995655226,
-2.69188717077969));
#41924=CARTESIAN_POINT('Ctrl Pts',(-0.0960869920911979,-0.120863908308893,
-2.69453626788234));
#41925=CARTESIAN_POINT('Ctrl Pts',(-0.132481275823141,-0.0793064053977654,
-2.69718536498499));
#41926=CARTESIAN_POINT('Ctrl Pts',(-0.143060535908398,-0.0319784475258966,
-2.69983446208764));
#41927=CARTESIAN_POINT('Ctrl Pts',(-0.145390141936173,-0.021556594291164,
-2.70041780653033));
#41928=CARTESIAN_POINT('Ctrl Pts',(-0.146467971154205,-0.0108549302842089,
-2.70100115097302));
#41929=CARTESIAN_POINT('Ctrl Pts',(-0.146368629392587,-0.000133465523585494,
-2.70158449541571));
#41930=CARTESIAN_POINT('Ctrl Pts',(-0.146408351835359,-0.0001286002260349,
-2.70871550458428));
#41931=CARTESIAN_POINT('Ctrl Pts',(-0.146494823460208,-0.00953807709170797,
-2.70820318707932));
#41932=CARTESIAN_POINT('Ctrl Pts',(-0.145665591675795,-0.0189323740934643,
-2.70769086957437));
#41933=CARTESIAN_POINT('Ctrl Pts',(-0.143865421359047,-0.0281367777804909,
-2.70717855206941));
#41934=CARTESIAN_POINT('Ctrl Pts',(-0.134557080487986,-0.0757310116352448,
-2.70452945496676));
#41935=CARTESIAN_POINT('Ctrl Pts',(-0.0992884757981104,-0.11824801311777,
-2.7018803578641));
#41936=CARTESIAN_POINT('Ctrl Pts',(-0.0542335261158874,-0.136189802744669,
-2.69923126076145));
#41937=CARTESIAN_POINT('Ctrl Pts',(-0.00917857643366479,-0.154131592371568,
-2.6965821636588));
#41938=CARTESIAN_POINT('Ctrl Pts',(0.0456627182409053,-0.14749817014284,
-2.69393306655615));
#41939=CARTESIAN_POINT('Ctrl Pts',(0.085140549564834,-0.119331573971797,
-2.6912839694535));
#41940=CARTESIAN_POINT('Ctrl Pts',(0.124618380888763,-0.0911649778007544,
-2.68863487235085));
#41941=CARTESIAN_POINT('Ctrl Pts',(0.14873274886205,-0.0414652076873958,
-2.6859857752482));
#41942=CARTESIAN_POINT('Ctrl Pts',(0.146424984348371,0.00697579280672859,
-2.68333667814555));
#41943=CARTESIAN_POINT('Ctrl Pts',(0.144117219834691,0.0554167933008527,
-2.6806875810429));
#41944=CARTESIAN_POINT('Ctrl Pts',(0.115387322834044,0.102599024175743,
-2.67803848394025));
#41945=CARTESIAN_POINT('Ctrl Pts',(0.0734106096394822,0.126885066572302,
-2.6753893868376));
#41946=CARTESIAN_POINT('Ctrl Pts',(0.0314338964449205,0.151171108968862,
-2.67274028973495));
#41947=CARTESIAN_POINT('Ctrl Pts',(-0.0237896329435564,0.15256096288709,
-2.6700911926323));
#41948=CARTESIAN_POINT('Ctrl Pts',(-0.0669348801970078,0.130417251695229,
-2.66744209552965));
#41949=CARTESIAN_POINT('Ctrl Pts',(-0.110080127450459,0.108273540503368,
-2.664792998427));
#41950=CARTESIAN_POINT('Ctrl Pts',(-0.141147092568885,0.0625962642014186,
-2.66214390132435));
#41951=CARTESIAN_POINT('Ctrl Pts',(-0.145888697266746,0.0143326807165443,
-2.6594948042217));
#41952=CARTESIAN_POINT('Ctrl Pts',(-0.146353652014044,0.00960002506664754,
-2.65923503767589));
#41953=CARTESIAN_POINT('Ctrl Pts',(-0.146565475951003,0.00484250084809524,
-2.65897527113009));
#41954=CARTESIAN_POINT('Ctrl Pts',(-0.146533501836025,8.20954179803956E-5,
-2.65871550458428));
#41955=CARTESIAN_POINT('Origin',(0.,0.,-1.487));
#41956=CARTESIAN_POINT('',(-0.146180868122056,9.89477992565866E-5,-2.60158449541571));
#41957=CARTESIAN_POINT('',(-0.146156100335505,8.29196033931501E-5,-2.60871550458429));
#41958=CARTESIAN_POINT('',(-0.14635,-1.79227059055215E-17,-1.487));
#41959=CARTESIAN_POINT('Ctrl Pts',(-0.146180868122056,9.89477992565866E-5,
-2.60158449541571));
#41960=CARTESIAN_POINT('Ctrl Pts',(-0.146290754520116,0.0178157742921191,
-2.60254531907455));
#41961=CARTESIAN_POINT('Ctrl Pts',(-0.143311879978458,0.0354969061612443,
-2.60350614273339));
#41962=CARTESIAN_POINT('Ctrl Pts',(-0.137079022290335,0.0519449678842955,
-2.60446696639222));
#41963=CARTESIAN_POINT('Ctrl Pts',(-0.119894344237327,0.0972940933496845,
-2.60711606349487));
#41964=CARTESIAN_POINT('Ctrl Pts',(-0.0779739962146589,0.133269840155799,
-2.60976516059752));
#41965=CARTESIAN_POINT('Ctrl Pts',(-0.0305423368863008,0.143373999379589,
-2.61241425770017));
#41966=CARTESIAN_POINT('Ctrl Pts',(0.0168893224420581,0.153478158603379,
-2.61506335480282));
#41967=CARTESIAN_POINT('Ctrl Pts',(0.0698322930761075,0.137710730244845,
-2.61771245190547));
#41968=CARTESIAN_POINT('Ctrl Pts',(0.104007323907182,0.103302539243917,
-2.62036154900813));
#41969=CARTESIAN_POINT('Ctrl Pts',(0.138182354738256,0.068894348242991,
-2.62301064611078));
#41970=CARTESIAN_POINT('Ctrl Pts',(0.153589445766355,0.0158453945996729,
-2.62565974321343));
#41971=CARTESIAN_POINT('Ctrl Pts',(0.143163020061337,-0.031516467560496,
-2.62830884031608));
#41972=CARTESIAN_POINT('Ctrl Pts',(0.132736594356318,-0.078878329720666,
-2.63095793741873));
#41973=CARTESIAN_POINT('Ctrl Pts',(0.0964766519181793,-0.120553100397687,
-2.63360703452138));
#41974=CARTESIAN_POINT('Ctrl Pts',(0.0510117316652691,-0.137429040865042,
-2.63625613162403));
#41975=CARTESIAN_POINT('Ctrl Pts',(0.00554681141235967,-0.154304981332397,
-2.63890522872668));
#41976=CARTESIAN_POINT('Ctrl Pts',(-0.049123086655321,-0.146382091590088,
-2.64155432582933));
#41977=CARTESIAN_POINT('Ctrl Pts',(-0.0879267553997137,-0.117293749728846,
-2.64420342293198));
#41978=CARTESIAN_POINT('Ctrl Pts',(-0.12396578813913,-0.0902778582269869,
-2.64666378042656));
#41979=CARTESIAN_POINT('Ctrl Pts',(-0.146318888092397,-0.0450050167475421,
-2.64912413792113));
#41980=CARTESIAN_POINT('Ctrl Pts',(-0.146559056518854,6.20051383258494E-5,
-2.65158449541571));
#41981=CARTESIAN_POINT('Ctrl Pts',(-0.146533501836025,8.20954179803956E-5,
-2.65871550458428));
#41982=CARTESIAN_POINT('Ctrl Pts',(-0.146239404188817,-0.0437040746677485,
-2.65632617402744));
#41983=CARTESIAN_POINT('Ctrl Pts',(-0.125319247018811,-0.0877340040481646,
-2.65393684347059));
#41984=CARTESIAN_POINT('Ctrl Pts',(-0.0910355793483402,-0.114897611025745,
-2.65154751291374));
#41985=CARTESIAN_POINT('Ctrl Pts',(-0.0530246124547761,-0.14501442861536,
-2.64889841581109));
#41986=CARTESIAN_POINT('Ctrl Pts',(0.00141356560964873,-0.154398173126793,
-2.64624931870844));
#41987=CARTESIAN_POINT('Ctrl Pts',(0.0473140127705487,-0.138745529377574,
-2.64360022160579));
#41988=CARTESIAN_POINT('Ctrl Pts',(0.0932144599314493,-0.123092885628354,
-2.64095112450314));
#41989=CARTESIAN_POINT('Ctrl Pts',(0.130577176188825,-0.0824038536184819,
-2.63830202740049));
#41990=CARTESIAN_POINT('Ctrl Pts',(0.142267898783137,-0.0353381196803642,
-2.63565293029784));
#41991=CARTESIAN_POINT('Ctrl Pts',(0.153958621377449,0.0117276142577528,
-2.63300383319519));
#41992=CARTESIAN_POINT('Ctrl Pts',(0.139977350308698,0.0651700501241154,
-2.63035473609254));
#41993=CARTESIAN_POINT('Ctrl Pts',(0.106735792117545,0.100480885783083,
-2.62770563898989));
#41994=CARTESIAN_POINT('Ctrl Pts',(0.0734942339263919,0.135791721442052,
-2.62505654188724));
#41995=CARTESIAN_POINT('Ctrl Pts',(0.0209923886128374,0.152970956893625,
-2.62240744478459));
#41996=CARTESIAN_POINT('Ctrl Pts',(-0.0266927894933914,0.144140323004268,
-2.61975834768194));
#41997=CARTESIAN_POINT('Ctrl Pts',(-0.07437796759962,0.135309689114912,
-2.61710925057929));
#41998=CARTESIAN_POINT('Ctrl Pts',(-0.117246478498522,0.100469185884624,
-2.61446015347664));
#41999=CARTESIAN_POINT('Ctrl Pts',(-0.135639143109211,0.0555964080072815,
-2.61181105637399));
#42000=CARTESIAN_POINT('Ctrl Pts',(-0.142803275345818,0.0381179990142528,
-2.61077920577742));
#42001=CARTESIAN_POINT('Ctrl Pts',(-0.146253974510039,0.0191175106607409,
-2.60974735518085));
#42002=CARTESIAN_POINT('Ctrl Pts',(-0.146156100335505,8.29196033931501E-5,
-2.60871550458429));
#42003=CARTESIAN_POINT('Origin',(0.,0.,-1.487));
#42004=CARTESIAN_POINT('',(-0.146198678720714,-0.000107744948522656,-2.55158449541571));
#42005=CARTESIAN_POINT('',(-0.146230181331583,-0.000119433189373819,-2.55871550458428));
#42006=CARTESIAN_POINT('',(-0.14635,-1.79227059055215E-17,-1.487));
#42007=CARTESIAN_POINT('Ctrl Pts',(-0.146198678720714,-0.000107744948522656,
-2.55158449541571));
#42008=CARTESIAN_POINT('Ctrl Pts',(-0.145981193910011,0.0318359205676525,
-2.55331740312531));
#42009=CARTESIAN_POINT('Ctrl Pts',(-0.135687907137135,0.0639071118611217,
-2.55505031083491));
#42010=CARTESIAN_POINT('Ctrl Pts',(-0.116406189831084,0.0890984680540818,
-2.55678321854451));
#42011=CARTESIAN_POINT('Ctrl Pts',(-0.0869302164906803,0.127608510067782,
-2.55943231564716));
#42012=CARTESIAN_POINT('Ctrl Pts',(-0.0364489496635117,0.15004088925777,
-2.56208141274981));
#42013=CARTESIAN_POINT('Ctrl Pts',(0.0118872785307486,0.146108283987278,
-2.56473050985246));
#42014=CARTESIAN_POINT('Ctrl Pts',(0.0602235067250097,0.142175678716785,
-2.56737960695512));
#42015=CARTESIAN_POINT('Ctrl Pts',(0.106414696286363,0.11187808898581,-2.57002870405777));
#42016=CARTESIAN_POINT('Ctrl Pts',(0.129277912503419,0.0691097632707052,
-2.57267780116042));
#42017=CARTESIAN_POINT('Ctrl Pts',(0.152141128720475,0.0263414375556003,
-2.57532689826307));
#42018=CARTESIAN_POINT('Ctrl Pts',(0.151676371593235,-0.0288976241436341,
-2.57797599536572));
#42019=CARTESIAN_POINT('Ctrl Pts',(0.128096775270796,-0.0712752004963703,
-2.58062509246837));
#42020=CARTESIAN_POINT('Ctrl Pts',(0.104517178948357,-0.113652776849106,
-2.58327418957102));
#42021=CARTESIAN_POINT('Ctrl Pts',(0.0578227434307195,-0.143168867855344,
-2.58592328667367));
#42022=CARTESIAN_POINT('Ctrl Pts',(0.00942718826804761,-0.146287614519936,
-2.58857238377632));
#42023=CARTESIAN_POINT('Ctrl Pts',(-0.038968366894625,-0.149406361184528,
-2.59122148087897));
#42024=CARTESIAN_POINT('Ctrl Pts',(-0.0890650417023317,-0.126127763507476,
-2.59387057798162));
#42025=CARTESIAN_POINT('Ctrl Pts',(-0.117888875064511,-0.0871272126066167,
-2.59651967508427));
#42026=CARTESIAN_POINT('Ctrl Pts',(-0.136258346068636,-0.0622721046854669,
-2.59820794852808));
#42027=CARTESIAN_POINT('Ctrl Pts',(-0.1459877855663,-0.0310314759797697,
-2.5998962219719));
#42028=CARTESIAN_POINT('Ctrl Pts',(-0.146180868122056,9.89477992565866E-5,
-2.60158449541571));
#42029=CARTESIAN_POINT('Ctrl Pts',(-0.146156100335505,8.29196033931501E-5,
-2.60871550458429));
#42030=CARTESIAN_POINT('Ctrl Pts',(-0.146002699574458,-0.0297504942499515,
-2.6070982580782));
#42031=CARTESIAN_POINT('Ctrl Pts',(-0.137132187551342,-0.0596676817879004,
-2.60548101157212));
#42032=CARTESIAN_POINT('Ctrl Pts',(-0.12017929978244,-0.0839397023494568,
-2.60386376506603));
#42033=CARTESIAN_POINT('Ctrl Pts',(-0.0924099735225071,-0.123697982304454,
-2.60121466796338));
#42034=CARTESIAN_POINT('Ctrl Pts',(-0.0429545026801662,-0.148309489690051,
-2.59856557086073));
#42035=CARTESIAN_POINT('Ctrl Pts',(0.00550720300589055,-0.146487570946361,
-2.59591647375808));
#42036=CARTESIAN_POINT('Ctrl Pts',(0.0539689086919474,-0.14466565220267,
-2.59326737665543));
#42037=CARTESIAN_POINT('Ctrl Pts',(0.10143684922172,-0.116410307329694,
-2.59061827955278));
#42038=CARTESIAN_POINT('Ctrl Pts',(0.126142581420765,-0.0746792265574484,
-2.58796918245013));
#42039=CARTESIAN_POINT('Ctrl Pts',(0.15084831361981,-0.0329481457852034,
-2.58532008534748));
#42040=CARTESIAN_POINT('Ctrl Pts',(0.152791837488128,0.0222586708863098,
-2.58267098824483));
#42041=CARTESIAN_POINT('Ctrl Pts',(0.131081867488292,0.0656237894554635,
-2.58002189114218));
#42042=CARTESIAN_POINT('Ctrl Pts',(0.109371897488455,0.108988908024618,
-2.57737279403953));
#42043=CARTESIAN_POINT('Ctrl Pts',(0.0640084336204636,0.140512328491412,
-2.57472369693687));
#42044=CARTESIAN_POINT('Ctrl Pts',(0.015794821771778,0.145737645554986,
-2.57207459983422));
#42045=CARTESIAN_POINT('Ctrl Pts',(-0.0324187900769076,0.150962962618561,
-2.56942550273157));
#42046=CARTESIAN_POINT('Ctrl Pts',(-0.0834825499062879,0.129890176278916,
-2.56677640562893));
#42047=CARTESIAN_POINT('Ctrl Pts',(-0.113978998654238,0.0921831090411383,
-2.56412730852628));
#42048=CARTESIAN_POINT('Ctrl Pts',(-0.134745923529105,0.0665060264716099,
-2.56232337387895));
#42049=CARTESIAN_POINT('Ctrl Pts',(-0.145975594133634,0.0331154724666765,
-2.56051943923161));
#42050=CARTESIAN_POINT('Ctrl Pts',(-0.146230181331583,-0.000119433189373819,
-2.55871550458428));
#42051=CARTESIAN_POINT('Origin',(0.,0.,-1.487));
#42052=CARTESIAN_POINT('',(-0.146571805443423,-4.82250285658153E-5,-2.50158449541571));
#42053=CARTESIAN_POINT('',(-0.14658585947319,-2.49429472847227E-5,-2.50871550458428));
#42054=CARTESIAN_POINT('',(-0.14635,-1.79227059055215E-17,-1.487));
#42055=CARTESIAN_POINT('Ctrl Pts',(-0.146571805443423,-4.82250285658153E-5,
-2.50158449541571));
#42056=CARTESIAN_POINT('Ctrl Pts',(-0.146375076469616,0.0458257689308958,
-2.50408948717608));
#42057=CARTESIAN_POINT('Ctrl Pts',(-0.123091181584723,0.0918718820885898,
-2.50659447893644));
#42058=CARTESIAN_POINT('Ctrl Pts',(-0.0859407318081494,0.118756594161564,
-2.5090994706968));
#42059=CARTESIAN_POINT('Ctrl Pts',(-0.0466531180034015,0.147187910377845,
-2.51174856779945));
#42060=CARTESIAN_POINT('Ctrl Pts',(0.00814235063893784,0.154189806754235,
-2.5143976649021));
#42061=CARTESIAN_POINT('Ctrl Pts',(0.0533168812526686,0.136551265882318,
-2.51704676200475));
#42062=CARTESIAN_POINT('Ctrl Pts',(0.0984914118663987,0.1189127250104,-2.51969585910741));
#42063=CARTESIAN_POINT('Ctrl Pts',(0.13404500445152,0.0766337468901765,
-2.52234495621006));
#42064=CARTESIAN_POINT('Ctrl Pts',(0.143673046859312,0.0291031552711476,
-2.52499405331271));
#42065=CARTESIAN_POINT('Ctrl Pts',(0.153301089267104,-0.0184274363478816,
-2.52764315041536));
#42066=CARTESIAN_POINT('Ctrl Pts',(0.137003581497565,-0.0712096414657163,
-2.53029224751801));
#42067=CARTESIAN_POINT('Ctrl Pts',(0.102254438951422,-0.105037934839297,
-2.53294134462066));
#42068=CARTESIAN_POINT('Ctrl Pts',(0.0675052964052803,-0.138866228212877,
-2.53559044172331));
#42069=CARTESIAN_POINT('Ctrl Pts',(0.0143045190825352,-0.153740609842205,
-2.53823953882596));
#42070=CARTESIAN_POINT('Ctrl Pts',(-0.0329504136852633,-0.142839799350687,
-2.54088863592861));
#42071=CARTESIAN_POINT('Ctrl Pts',(-0.0802053464530617,-0.131938988859169,
-2.54353773303126));
#42072=CARTESIAN_POINT('Ctrl Pts',(-0.121514434665913,-0.0952629862468065,
-2.54618683013391));
#42073=CARTESIAN_POINT('Ctrl Pts',(-0.13793363884552,-0.0496311325219192,
-2.54883592723656));
#42074=CARTESIAN_POINT('Ctrl Pts',(-0.14361221540529,-0.0338493703788515,
-2.54975211662961));
#42075=CARTESIAN_POINT('Ctrl Pts',(-0.146313663076552,-0.0169963809438984,
-2.55066830602266));
#42076=CARTESIAN_POINT('Ctrl Pts',(-0.146198678720714,-0.000107744948522656,
-2.55158449541571));
#42077=CARTESIAN_POINT('Ctrl Pts',(-0.146230181331583,-0.000119433189373819,
-2.55871550458428));
#42078=CARTESIAN_POINT('Ctrl Pts',(-0.146349458125579,-0.0156903378827077,
-2.55787034212896));
#42079=CARTESIAN_POINT('Ctrl Pts',(-0.144059680438183,-0.0312270774277224,
-2.55702517967364));
#42080=CARTESIAN_POINT('Ctrl Pts',(-0.139212983241851,-0.0459203987745881,
-2.55618001721832));
#42081=CARTESIAN_POINT('Ctrl Pts',(-0.124021381414995,-0.0919754912166281,
-2.55353092011567));
#42082=CARTESIAN_POINT('Ctrl Pts',(-0.083709040094762,-0.129744327964798,
-2.55088182301302));
#42083=CARTESIAN_POINT('Ctrl Pts',(-0.0367628980753028,-0.141906402434203,
-2.54823272591037));
#42084=CARTESIAN_POINT('Ctrl Pts',(0.0101832439441568,-0.154068476903608,
-2.54558362880772));
#42085=CARTESIAN_POINT('Ctrl Pts',(0.0637631866628425,-0.140623789094247,
-2.54293453170507));
#42086=CARTESIAN_POINT('Ctrl Pts',(0.099405568329131,-0.107737972469671,
-2.54028543460242));
#42087=CARTESIAN_POINT('Ctrl Pts',(0.135047949995419,-0.074852155845095,
-2.53763633749977));
#42088=CARTESIAN_POINT('Ctrl Pts',(0.15275277060931,-0.0225252104053042,
-2.53498724039712));
#42089=CARTESIAN_POINT('Ctrl Pts',(0.144400731605375,0.0252461172964389,
-2.53233814329447));
#42090=CARTESIAN_POINT('Ctrl Pts',(0.13604869260144,0.0730174449981818,
-2.52968904619182));
#42091=CARTESIAN_POINT('Ctrl Pts',(0.10163979397968,0.116233154961878,-2.52703994908917));
#42092=CARTESIAN_POINT('Ctrl Pts',(0.0569536997824638,0.135074845207396,
-2.52439085198652));
#42093=CARTESIAN_POINT('Ctrl Pts',(0.0122676055852467,0.153916535452915,
-2.52174175488387));
#42094=CARTESIAN_POINT('Ctrl Pts',(-0.0426956841874264,0.148384205980257,
-2.51909265778122));
#42095=CARTESIAN_POINT('Ctrl Pts',(-0.0827304151517853,0.121014941786237,
-2.51644356067857));
#42096=CARTESIAN_POINT('Ctrl Pts',(-0.121660741803148,0.094400690369656,
-2.51386754198047));
#42097=CARTESIAN_POINT('Ctrl Pts',(-0.146474792161809,0.0471376805651769,
-2.51129152328238));
#42098=CARTESIAN_POINT('Ctrl Pts',(-0.14658585947319,-2.49429472847227E-5,
-2.50871550458428));
#42099=CARTESIAN_POINT('Origin',(0.,0.,-1.487));
#42100=CARTESIAN_POINT('',(-0.146343637318237,0.000134580547271598,-2.45158449541571));
#42101=CARTESIAN_POINT('',(-0.146304536544652,0.000133297989308676,-2.45871550458428));
#42102=CARTESIAN_POINT('',(-0.14635,-1.79227059055215E-17,-1.487));
#42103=CARTESIAN_POINT('Ctrl Pts',(-0.146343637318237,0.000134580547271598,
-2.45158449541571));
#42104=CARTESIAN_POINT('Ctrl Pts',(-0.146449762957763,0.0116814355873594,
-2.45221247412419));
#42105=CARTESIAN_POINT('Ctrl Pts',(-0.145198490549426,0.0232055565890608,
-2.45284045283267));
#42106=CARTESIAN_POINT('Ctrl Pts',(-0.142502216361462,0.0343810467066606,
-2.45346843154114));
#42107=CARTESIAN_POINT('Ctrl Pts',(-0.131128117139851,0.081524298685688,
-2.45611752864379));
#42108=CARTESIAN_POINT('Ctrl Pts',(-0.0940397420577331,0.122463550881684,
-2.45876662574644));
#42109=CARTESIAN_POINT('Ctrl Pts',(-0.0482455430596612,0.13842436785282,
-2.46141572284909));
#42110=CARTESIAN_POINT('Ctrl Pts',(-0.00245134406158928,0.154385184823957,
-2.46406481995174));
#42111=CARTESIAN_POINT('Ctrl Pts',(0.0520486788524363,0.145367566570235,
-2.4667139170544));
#42112=CARTESIAN_POINT('Ctrl Pts',(0.0902612220216918,0.115506925505467,
-2.46936301415705));
#42113=CARTESIAN_POINT('Ctrl Pts',(0.128473765190947,0.0856462844406988,
-2.4720121112597));
#42114=CARTESIAN_POINT('Ctrl Pts',(0.150398828615432,0.0349426205648845,
-2.47466120836235));
#42115=CARTESIAN_POINT('Ctrl Pts',(0.145981741881279,-0.0133517443760076,
-2.477310305465));
#42116=CARTESIAN_POINT('Ctrl Pts',(0.141564655147125,-0.0616461093169007,
-2.47995940256765));
#42117=CARTESIAN_POINT('Ctrl Pts',(0.110805418254332,-0.107531175322872,
-2.4826084996703));
#42118=CARTESIAN_POINT('Ctrl Pts',(0.0678099876214229,-0.129964393659791,
-2.48525759677295));
#42119=CARTESIAN_POINT('Ctrl Pts',(0.0248145569885134,-0.152397611996709,
-2.4879066938756));
#42120=CARTESIAN_POINT('Ctrl Pts',(-0.0304170673845123,-0.151378982664575,
-2.49055579097825));
#42121=CARTESIAN_POINT('Ctrl Pts',(-0.072556074869304,-0.127375641470944,
-2.4932048880809));
#42122=CARTESIAN_POINT('Ctrl Pts',(-0.114695082354095,-0.103372300277313,
-2.49585398518355));
#42123=CARTESIAN_POINT('Ctrl Pts',(-0.143741472950652,-0.0563842472221864,
-2.4985030822862));
#42124=CARTESIAN_POINT('Ctrl Pts',(-0.146374788765353,-0.00795985266653731,
-2.50115217938885));
#42125=CARTESIAN_POINT('Ctrl Pts',(-0.146518035638578,-0.00532566687340771,
-2.50129628473114));
#42126=CARTESIAN_POINT('Ctrl Pts',(-0.146583122724603,-0.00268723075550709,
-2.50144039007342));
#42127=CARTESIAN_POINT('Ctrl Pts',(-0.146571805443423,-4.82250285658153E-5,
-2.50158449541571));
#42128=CARTESIAN_POINT('Ctrl Pts',(-0.14658585947319,-2.49429472847227E-5,
-2.50871550458428));
#42129=CARTESIAN_POINT('Ctrl Pts',(-0.146589010312864,-0.00136288714913549,
-2.50864242617973));
#42130=CARTESIAN_POINT('Ctrl Pts',(-0.146572280552286,-0.00270075056156342,
-2.50856934777517));
#42131=CARTESIAN_POINT('Ctrl Pts',(-0.146535428489023,-0.00403805946607697,
-2.50849626937062));
#42132=CARTESIAN_POINT('Ctrl Pts',(-0.145199538705858,-0.0525155976089924,
-2.50584717226796));
#42133=CARTESIAN_POINT('Ctrl Pts',(-0.117421586983486,-0.100264474979443,
-2.50319807516531));
#42134=CARTESIAN_POINT('Ctrl Pts',(-0.0759403346168386,-0.125387412865071,
-2.50054897806266));
#42135=CARTESIAN_POINT('Ctrl Pts',(-0.0344590822501911,-0.150510350750698,
-2.49789988096001));
#42136=CARTESIAN_POINT('Ctrl Pts',(0.0207254707607316,-0.153007349151502,
-2.49525078385736));
#42137=CARTESIAN_POINT('Ctrl Pts',(0.0643061003628465,-0.131733303241195,
-2.49260168675471));
#42138=CARTESIAN_POINT('Ctrl Pts',(0.107886729964961,-0.110459257330887,
-2.48995258965206));
#42139=CARTESIAN_POINT('Ctrl Pts',(0.139863436158269,-0.0654141671094696,
-2.48730349254941));
#42140=CARTESIAN_POINT('Ctrl Pts',(0.14557194019155,-0.0172553746867708,
-2.48465439544676));
#42141=CARTESIAN_POINT('Ctrl Pts',(0.151280444224832,0.0309034177359276,
-2.48200529834411));
#42142=CARTESIAN_POINT('Ctrl Pts',(0.130720746098087,0.0821759123599069,
-2.47935620124146));
#42143=CARTESIAN_POINT('Ctrl Pts',(0.0933213698922176,0.113048925904464,
-2.47670710413881));
#42144=CARTESIAN_POINT('Ctrl Pts',(0.0559219936863476,0.143921939449022,
-2.47405800703616));
#42145=CARTESIAN_POINT('Ctrl Pts',(0.00168293940135239,0.154395471914157,
-2.47140890993351));
#42146=CARTESIAN_POINT('Ctrl Pts',(-0.0445221675671624,0.139666439497234,
-2.46875981283086));
#42147=CARTESIAN_POINT('Ctrl Pts',(-0.0907272745356775,0.124937407080312,
-2.46611071572821));
#42148=CARTESIAN_POINT('Ctrl Pts',(-0.128898434187712,0.0850058097813312,
-2.46346161862556));
#42149=CARTESIAN_POINT('Ctrl Pts',(-0.141530637658034,0.0381839800285859,
-2.46081252152291));
#42150=CARTESIAN_POINT('Ctrl Pts',(-0.144863841843323,0.0258293089483245,
-2.4601135158767));
#42151=CARTESIAN_POINT('Ctrl Pts',(-0.146418894550156,0.01299490498715,
-2.45941451023049));
#42152=CARTESIAN_POINT('Ctrl Pts',(-0.146304536544652,0.000133297989308676,
-2.45871550458428));
#42153=CARTESIAN_POINT('Origin',(0.,0.,-1.487));
#42154=CARTESIAN_POINT('',(-0.146111815181358,-2.28850520822416E-5,-2.40158449541571));
#42155=CARTESIAN_POINT('',(-0.14612072978227,-4.38323123618543E-5,-2.40871550458428));
#42156=CARTESIAN_POINT('',(-0.14635,-1.79227059055215E-17,-1.487));
#42157=CARTESIAN_POINT('Ctrl Pts',(-0.146111815181358,-2.28850520822416E-5,
-2.40158449541571));
#42158=CARTESIAN_POINT('Ctrl Pts',(-0.146075798550186,0.0258236983025542,
-2.40298455817495));
#42159=CARTESIAN_POINT('Ctrl Pts',(-0.139550277491284,0.0516872750199038,
-2.40438462093419));
#42160=CARTESIAN_POINT('Ctrl Pts',(-0.126641700285093,0.0738296538626264,
-2.40578468369343));
#42161=CARTESIAN_POINT('Ctrl Pts',(-0.10221702771199,0.115725855479931,
-2.40843378079608));
#42162=CARTESIAN_POINT('Ctrl Pts',(-0.0549400816815103,0.144299625105766,
-2.41108287789873));
#42163=CARTESIAN_POINT('Ctrl Pts',(-0.00649171671651216,0.146447245295523,
-2.41373197500138));
#42164=CARTESIAN_POINT('Ctrl Pts',(0.0419566482484867,0.14859486548528,
-2.41638107210403));
#42165=CARTESIAN_POINT('Ctrl Pts',(0.0915764321480043,0.124316336238958,
-2.41903016920669));
#42166=CARTESIAN_POINT('Ctrl Pts',(0.119612372501939,0.0847456098274833,
-2.42167926630934));
#42167=CARTESIAN_POINT('Ctrl Pts',(0.147648312855873,0.0451748834160083,
-2.42432836341199));
#42168=CARTESIAN_POINT('Ctrl Pts',(0.154100409664225,-0.00968804016061831,
-2.42697746051464));
#42169=CARTESIAN_POINT('Ctrl Pts',(0.136009779496176,-0.0546834337068921,
-2.42962655761729));
#42170=CARTESIAN_POINT('Ctrl Pts',(0.117919149328128,-0.0996788272531659,
-2.43227565471994));
#42171=CARTESIAN_POINT('Ctrl Pts',(0.0752857921836774,-0.134806690769086,
-2.43492475182259));
#42172=CARTESIAN_POINT('Ctrl Pts',(0.0276610473873672,-0.143957648278959,
-2.43757384892524));
#42173=CARTESIAN_POINT('Ctrl Pts',(-0.0199636974089416,-0.153108605788832,
-2.44022294602789));
#42174=CARTESIAN_POINT('Ctrl Pts',(-0.0725798298571109,-0.136282657292659,
-2.44287204313054));
#42175=CARTESIAN_POINT('Ctrl Pts',(-0.106057984400644,-0.101196057163545,
-2.44552114023319));
#42176=CARTESIAN_POINT('Ctrl Pts',(-0.131600012997177,-0.0744268712250649,
-2.44754225862736));
#42177=CARTESIAN_POINT('Ctrl Pts',(-0.146002077199647,-0.0370284009381002,
-2.44956337702154));
#42178=CARTESIAN_POINT('Ctrl Pts',(-0.146343637318237,0.000134580547271598,
-2.45158449541571));
#42179=CARTESIAN_POINT('Ctrl Pts',(-0.146304536544652,0.000133297989308676,
-2.45871550458428));
#42180=CARTESIAN_POINT('Ctrl Pts',(-0.145985499680331,-0.0357481144981475,
-2.45676541312784));
#42181=CARTESIAN_POINT('Ctrl Pts',(-0.132673392532962,-0.0718412489811016,
-2.4548153216714));
#42182=CARTESIAN_POINT('Ctrl Pts',(-0.108729319967223,-0.0983202558284832,
-2.45286523021495));
#42183=CARTESIAN_POINT('Ctrl Pts',(-0.0762025515174788,-0.134290599726301,
-2.4502161331123));
#42184=CARTESIAN_POINT('Ctrl Pts',(-0.0240557673293792,-0.152519225315428,
-2.44756703600965));
#42185=CARTESIAN_POINT('Ctrl Pts',(0.0237969066489193,-0.144646620979046,
-2.444917938907));
#42186=CARTESIAN_POINT('Ctrl Pts',(0.0716495806272191,-0.136774016642663,
-2.44226884180435));
#42187=CARTESIAN_POINT('Ctrl Pts',(0.115208144395718,-0.102800182380768,
-2.4396197447017));
#42188=CARTESIAN_POINT('Ctrl Pts',(0.134496965778837,-0.0583052649680928,
-2.43697064759905));
#42189=CARTESIAN_POINT('Ctrl Pts',(0.153785787161955,-0.0138103475554188,
-2.4343215504964));
#42190=CARTESIAN_POINT('Ctrl Pts',(0.148804866159696,0.0412056530080348,
-2.43167245339375));
#42191=CARTESIAN_POINT('Ctrl Pts',(0.121838415960665,0.0815128095633379,
-2.4290233562911));
#42192=CARTESIAN_POINT('Ctrl Pts',(0.0948719657616343,0.121819966118641,
-2.42637425918845));
#42193=CARTESIAN_POINT('Ctrl Pts',(0.0459199863658311,0.147418278665793,
-2.4237251620858));
#42194=CARTESIAN_POINT('Ctrl Pts',(-0.00256850990682517,0.146568552164411,
-2.42107606498315));
#42195=CARTESIAN_POINT('Ctrl Pts',(-0.0510570061794814,0.145718825663028,
-2.4184269678805));
#42196=CARTESIAN_POINT('Ctrl Pts',(-0.0990820193289911,0.118421060113111,
-2.41577787077785));
#42197=CARTESIAN_POINT('Ctrl Pts',(-0.124619636836098,0.0771938070155387,
-2.4131287736752));
#42198=CARTESIAN_POINT('Ctrl Pts',(-0.138801120014761,0.0542995963029285,
-2.41165768397823));
#42199=CARTESIAN_POINT('Ctrl Pts',(-0.14604799843459,0.0271098463392561,
-2.41018659428125));
#42200=CARTESIAN_POINT('Ctrl Pts',(-0.14612072978227,-4.38323123618543E-5,
-2.40871550458428));
#42201=CARTESIAN_POINT('Origin',(0.,0.,-1.487));
#42202=CARTESIAN_POINT('',(-0.14642783004434,-0.00012476929814137,-2.35158449541571));
#42203=CARTESIAN_POINT('',(-0.146465637571143,-0.000114315844697511,-2.35871550458428));
#42204=CARTESIAN_POINT('',(-0.14635,-1.79227059055215E-17,-1.487));
#42205=CARTESIAN_POINT('Ctrl Pts',(-0.14642783004434,-0.00012476929814137,
-2.35158449541571));
#42206=CARTESIAN_POINT('Ctrl Pts',(-0.146066603696939,0.0397562668171756,
-2.35375664222571));
#42207=CARTESIAN_POINT('Ctrl Pts',(-0.129170826335352,0.0799065680416143,
-2.35592878903572));
#42208=CARTESIAN_POINT('Ctrl Pts',(-0.100127500298616,0.107067370027125,
-2.35810093584572));
#42209=CARTESIAN_POINT('Ctrl Pts',(-0.0647069704795052,0.14019201957387,
-2.36075003294837));
#42210=CARTESIAN_POINT('Ctrl Pts',(-0.0112186082459791,0.153996549344,-2.36339913005103));
#42211=CARTESIAN_POINT('Ctrl Pts',(0.0358082227771749,0.142150305037009,
-2.36604822715368));
#42212=CARTESIAN_POINT('Ctrl Pts',(0.0828350538003276,0.130304060730019,
-2.36869732425633));
#42213=CARTESIAN_POINT('Ctrl Pts',(0.123400353613109,0.092807042345909,
-2.37134642135898));
#42214=CARTESIAN_POINT('Ctrl Pts',(0.138901178545045,0.0468551025969656,
-2.37399551846163));
#42215=CARTESIAN_POINT('Ctrl Pts',(0.154402003476981,0.000903162848020875,
-2.37664461556428));
#42216=CARTESIAN_POINT('Ctrl Pts',(0.144838353528071,-0.053503698265758,
-2.37929371266693));
#42217=CARTESIAN_POINT('Ctrl Pts',(0.114596047171364,-0.0914149003897779,
-2.38194280976958));
#42218=CARTESIAN_POINT('Ctrl Pts',(0.0843537408146581,-0.129326102513797,
-2.38459190687223));
#42219=CARTESIAN_POINT('Ctrl Pts',(0.0334327780501559,-0.150741645648058,
-2.38724100397488));
#42220=CARTESIAN_POINT('Ctrl Pts',(-0.0148148677279785,-0.145840521580174,
-2.38989010107753));
#42221=CARTESIAN_POINT('Ctrl Pts',(-0.0630625135061135,-0.140939397512289,
-2.39253919818018));
#42222=CARTESIAN_POINT('Ctrl Pts',(-0.108636842297881,-0.109721606242258,
-2.39518829528283));
#42223=CARTESIAN_POINT('Ctrl Pts',(-0.130637807135901,-0.0665033938028552,
-2.39783739238548));
#42224=CARTESIAN_POINT('Ctrl Pts',(-0.141011137975052,-0.0461262503815869,
-2.39908642672889));
#42225=CARTESIAN_POINT('Ctrl Pts',(-0.146143946604733,-0.0230813301515235,
-2.4003354610723));
#42226=CARTESIAN_POINT('Ctrl Pts',(-0.146111815181358,-2.28850520822416E-5,
-2.40158449541571));
#42227=CARTESIAN_POINT('Ctrl Pts',(-0.14612072978227,-4.38323123618543E-5,
-2.40871550458428));
#42228=CARTESIAN_POINT('Ctrl Pts',(-0.146178971007376,-0.0217877372618158,
-2.4075374971786));
#42229=CARTESIAN_POINT('Ctrl Pts',(-0.141636892583024,-0.0435085119960741,
-2.40635948977292));
#42230=CARTESIAN_POINT('Ctrl Pts',(-0.132371493453238,-0.0629819454103503,
-2.40518148236724));
#42231=CARTESIAN_POINT('Ctrl Pts',(-0.111535510698569,-0.106773704093438,
-2.40253238526459));
#42232=CARTESIAN_POINT('Ctrl Pts',(-0.0668133233245271,-0.139200480814385,
-2.39988328816194));
#42233=CARTESIAN_POINT('Ctrl Pts',(-0.0187141926056368,-0.145391597837813,
-2.39723419105929));
#42234=CARTESIAN_POINT('Ctrl Pts',(0.0293849381132521,-0.15158271486124,
-2.39458509395664));
#42235=CARTESIAN_POINT('Ctrl Pts',(0.0808610121769882,-0.131538172187151,
-2.39193599685399));
#42236=CARTESIAN_POINT('Ctrl Pts',(0.112107486293538,-0.0944502474515405,
-2.38928689975134));
#42237=CARTESIAN_POINT('Ctrl Pts',(0.143353960410089,-0.0573623227159294,
-2.38663780264869));
#42238=CARTESIAN_POINT('Ctrl Pts',(0.154370834579451,-0.00323101591879572,
-2.38398870554604));
#42239=CARTESIAN_POINT('Ctrl Pts',(0.140105852549527,0.0431194597378418,
-2.38133960844339));
#42240=CARTESIAN_POINT('Ctrl Pts',(0.125840870519603,0.0894699353944787,
-2.37869051134074));
#42241=CARTESIAN_POINT('Ctrl Pts',(0.0862940322903931,0.128039579910621,
-2.37604141423809));
#42242=CARTESIAN_POINT('Ctrl Pts',(0.0396012226530549,0.141140642237083,
-2.37339231713544));
#42243=CARTESIAN_POINT('Ctrl Pts',(-0.0070915869842839,0.154241704563545,
-2.37074322003279));
#42244=CARTESIAN_POINT('Ctrl Pts',(-0.0609303680297501,0.141874184700328,
-2.36809412293014));
#42245=CARTESIAN_POINT('Ctrl Pts',(-0.097225057407312,0.109709734932038,
-2.36544502582749));
#42246=CARTESIAN_POINT('Ctrl Pts',(-0.127958281309316,0.0824738705847656,
-2.36320185207975));
#42247=CARTESIAN_POINT('Ctrl Pts',(-0.146112075293418,0.0410432507012986,
-2.36095867833202));
#42248=CARTESIAN_POINT('Ctrl Pts',(-0.146465637571143,-0.000114315844697511,
-2.35871550458428));
#42249=CARTESIAN_POINT('Origin',(0.,0.,-1.487));
#42250=CARTESIAN_POINT('',(-0.146518717508966,9.11058135677975E-5,-2.30158449541571));
#42251=CARTESIAN_POINT('',(-0.146485691396121,0.00010691274947015,-2.30871550458428));
#42252=CARTESIAN_POINT('',(-0.14635,-1.79227059055215E-17,-1.487));
#42253=CARTESIAN_POINT('Ctrl Pts',(-0.146518717508966,9.11058135677975E-5,
-2.30158449541571));
#42254=CARTESIAN_POINT('Ctrl Pts',(-0.146558146874483,0.0055010752982445,
-2.30187962917383));
#42255=CARTESIAN_POINT('Ctrl Pts',(-0.146284538842059,0.0109070158290159,
-2.30217476293194));
#42256=CARTESIAN_POINT('Ctrl Pts',(-0.145684637283403,0.0162765014723047,
-2.30246989669006));
#42257=CARTESIAN_POINT('Ctrl Pts',(-0.140299968680779,0.0644725768758163,
-2.30511899379271));
#42258=CARTESIAN_POINT('Ctrl Pts',(-0.10862676192489,0.10973158603861,-2.30776809089536));
#42259=CARTESIAN_POINT('Ctrl Pts',(-0.0651901131906062,0.131298085221265,
-2.31041718799801));
#42260=CARTESIAN_POINT('Ctrl Pts',(-0.0217534644563208,0.152864584403921,
-2.31306628510066));
#42261=CARTESIAN_POINT('Ctrl Pts',(0.0334466262563611,0.150738573606437,
-2.31571538220332));
#42262=CARTESIAN_POINT('Ctrl Pts',(0.0750958094203205,0.125895025509674,
-2.31836447930597));
#42263=CARTESIAN_POINT('Ctrl Pts',(0.11674499258428,0.101051477412912,-2.32101357640862));
#42264=CARTESIAN_POINT('Ctrl Pts',(0.144843268199517,0.0534903920168709,
-2.32366267351127));
#42265=CARTESIAN_POINT('Ctrl Pts',(0.146504976825077,0.00502292803633103,
-2.32631177061392));
#42266=CARTESIAN_POINT('Ctrl Pts',(0.148166685450637,-0.0434445359442082,
-2.32896086771657));
#42267=CARTESIAN_POINT('Ctrl Pts',(0.123391827086521,-0.0928183785092465,
-2.33160996481922));
#42268=CARTESIAN_POINT('Ctrl Pts',(0.0835419668319325,-0.120456124038701,
-2.33425906192187));
#42269=CARTESIAN_POINT('Ctrl Pts',(0.0436921065773438,-0.148093869568155,
-2.33690815902452));
#42270=CARTESIAN_POINT('Ctrl Pts',(-0.0112327555677177,-0.153995518062025,
-2.33955725612717));
#42271=CARTESIAN_POINT('Ctrl Pts',(-0.0560444878426382,-0.135454617577368,
-2.34220635322982));
#42272=CARTESIAN_POINT('Ctrl Pts',(-0.100856220117559,-0.11691371709271,
-2.34485545033247));
#42273=CARTESIAN_POINT('Ctrl Pts',(-0.135554822522338,-0.0739302676295245,
-2.34750454743512));
#42274=CARTESIAN_POINT('Ctrl Pts',(-0.14422777502238,-0.0262161582362525,
-2.35015364453777));
#42275=CARTESIAN_POINT('Ctrl Pts',(-0.145789275817825,-0.0176255865974496,
-2.35063059483042));
#42276=CARTESIAN_POINT('Ctrl Pts',(-0.146507146511952,-0.00888166904295471,
-2.35110754512306));
#42277=CARTESIAN_POINT('Ctrl Pts',(-0.14642783004434,-0.00012476929814137,
-2.35158449541571));
#42278=CARTESIAN_POINT('Ctrl Pts',(-0.146465637571143,-0.000114315844697511,
-2.35871550458428));
#42279=CARTESIAN_POINT('Ctrl Pts',(-0.146529617985541,-0.00756216401491792,
-2.35830958122937));
#42280=CARTESIAN_POINT('Ctrl Pts',(-0.146010706652304,-0.0150010706983251,
-2.35790365787445));
#42281=CARTESIAN_POINT('Ctrl Pts',(-0.144877966401556,-0.0223453032662951,
-2.35749773451953));
#42282=CARTESIAN_POINT('Ctrl Pts',(-0.137485588308582,-0.0702745120229723,
-2.35484863741688));
#42283=CARTESIAN_POINT('Ctrl Pts',(-0.103950234412977,-0.114171549862962,
-2.35219954031423));
#42284=CARTESIAN_POINT('Ctrl Pts',(-0.0596509676667877,-0.13390556292824,
-2.34955044321158));
#42285=CARTESIAN_POINT('Ctrl Pts',(-0.0153517009205988,-0.153639575993518,
-2.34690134610893));
#42286=CARTESIAN_POINT('Ctrl Pts',(0.0397114786761746,-0.149210564284086,
-2.34425224900628));
#42287=CARTESIAN_POINT('Ctrl Pts',(0.0802870080121162,-0.122649639506912,
-2.34160315190363));
#42288=CARTESIAN_POINT('Ctrl Pts',(0.120862537348058,-0.096088714729738,
-2.33895405480098));
#42289=CARTESIAN_POINT('Ctrl Pts',(0.146950416423168,-0.0473958768848222,
-2.33630495769833));
#42290=CARTESIAN_POINT('Ctrl Pts',(0.146586938642,0.00109870208863794,-2.33365586059568));
#42291=CARTESIAN_POINT('Ctrl Pts',(0.146223460860833,0.0495932810620981,
-2.33100676349303));
#42292=CARTESIAN_POINT('Ctrl Pts',(0.119408626223387,0.0978896011641026,
-2.32835766639038));
#42293=CARTESIAN_POINT('Ctrl Pts',(0.0784395177192075,0.123839330532312,
-2.32570856928773));
#42294=CARTESIAN_POINT('Ctrl Pts',(0.0374704092150271,0.149789059900522,
-2.32305947218508));
#42295=CARTESIAN_POINT('Ctrl Pts',(-0.0176529731558879,0.153392198534936,
-2.32041037508243));
#42296=CARTESIAN_POINT('Ctrl Pts',(-0.0616514577393187,0.132996373955571,
-2.31776127797978));
#42297=CARTESIAN_POINT('Ctrl Pts',(-0.105649942322749,0.112600549376206,
-2.31511218087712));
#42298=CARTESIAN_POINT('Ctrl Pts',(-0.138523529118695,0.0682057615830633,
-2.31246308377448));
#42299=CARTESIAN_POINT('Ctrl Pts',(-0.145196636626864,0.0201711288469323,
-2.30981398667183));
#42300=CARTESIAN_POINT('Ctrl Pts',(-0.146118999829862,0.0135317366820221,
-2.30944782597598));
#42301=CARTESIAN_POINT('Ctrl Pts',(-0.146540802124392,0.00682280517505123,
-2.30908166528013));
#42302=CARTESIAN_POINT('Ctrl Pts',(-0.146485691396121,0.00010691274947015,
-2.30871550458428));
#42303=CARTESIAN_POINT('Origin',(0.,0.,-1.487));
#42304=CARTESIAN_POINT('',(-0.14614553911452,7.41235706846755E-5,-2.25158449541571));
#42305=CARTESIAN_POINT('',(-0.146128142350211,5.51125628420172E-5,-2.25871550458428));
#42306=CARTESIAN_POINT('',(-0.14635,-1.79227059055215E-17,-1.487));
#42307=CARTESIAN_POINT('Ctrl Pts',(-0.14614553911452,7.41235706846755E-5,
-2.25158449541571));
#42308=CARTESIAN_POINT('Ctrl Pts',(-0.146235642754429,0.0197646966306404,
-2.25265171322459));
#42309=CARTESIAN_POINT('Ctrl Pts',(-0.142535886262011,0.039422814349067,
-2.25371893103347));
#42310=CARTESIAN_POINT('Ctrl Pts',(-0.134885835946401,0.0573999068084199,
-2.25478614884235));
#42311=CARTESIAN_POINT('Ctrl Pts',(-0.115896529398507,0.102023472074894,
-2.257435245945));
#42312=CARTESIAN_POINT('Ctrl Pts',(-0.0725673095232115,0.13628932448801,
-2.26008434304765));
#42313=CARTESIAN_POINT('Ctrl Pts',(-0.0247686330987405,0.144483399928831,
-2.2627334401503));
#42314=CARTESIAN_POINT('Ctrl Pts',(0.0230300433257305,0.152677475369652,
-2.26538253725296));
#42315=CARTESIAN_POINT('Ctrl Pts',(0.0752981762993759,0.134799773838178,
-2.2680316343556));
#42316=CARTESIAN_POINT('Ctrl Pts',(0.108065990226868,0.0990488757980672,
-2.27068073145825));
#42317=CARTESIAN_POINT('Ctrl Pts',(0.140833804154361,0.0632979777579564,
-2.2733298285609));
#42318=CARTESIAN_POINT('Ctrl Pts',(0.1541012990357,0.00967388320920951,
-2.27597892566356));
#42319=CARTESIAN_POINT('Ctrl Pts',(0.141784100761364,-0.0372317983968804,
-2.27862802276621));
#42320=CARTESIAN_POINT('Ctrl Pts',(0.129466902487028,-0.0841374800029696,
-2.28127711986886));
#42321=CARTESIAN_POINT('Ctrl Pts',(0.0915650110570157,-0.124324748666403,
-2.28392621697151));
#42322=CARTESIAN_POINT('Ctrl Pts',(0.0454599509400524,-0.139364022979758,
-2.28657531407416));
#42323=CARTESIAN_POINT('Ctrl Pts',(-0.000645109176910887,-0.154403297293113,
-2.28922441117681));
#42324=CARTESIAN_POINT('Ctrl Pts',(-0.0549533379808256,-0.144294577256392,
-2.29187350827946));
#42325=CARTESIAN_POINT('Ctrl Pts',(-0.0925593871581046,-0.113673646415916,
-2.29452260538211));
#42326=CARTESIAN_POINT('Ctrl Pts',(-0.125975776918769,-0.0864641686274881,
-2.29687656872664));
#42327=CARTESIAN_POINT('Ctrl Pts',(-0.146204232030531,-0.043058379840643,
-2.29923053207118));
#42328=CARTESIAN_POINT('Ctrl Pts',(-0.146518717508966,9.11058135677975E-5,
-2.30158449541571));
#42329=CARTESIAN_POINT('Ctrl Pts',(-0.146485691396121,0.00010691274947015,
-2.30871550458428));
#42330=CARTESIAN_POINT('Ctrl Pts',(-0.146142087373619,-0.0417652911665238,
-2.30643256817748));
#42331=CARTESIAN_POINT('Ctrl Pts',(-0.127259609035765,-0.0839080844543,
-2.30414963177068));
#42332=CARTESIAN_POINT('Ctrl Pts',(-0.0955696282125509,-0.111154774481476,
-2.30186669536387));
#42333=CARTESIAN_POINT('Ctrl Pts',(-0.0587968840696793,-0.142771567394633,
-2.29921759826122));
#42334=CARTESIAN_POINT('Ctrl Pts',(-0.00477876756354516,-0.154330675541829,
-2.29656850115857));
#42335=CARTESIAN_POINT('Ctrl Pts',(0.0417124163263103,-0.140531178216557,
-2.29391940405592));
#42336=CARTESIAN_POINT('Ctrl Pts',(0.0882036002161671,-0.126731680891284,
-2.29127030695327));
#42337=CARTESIAN_POINT('Ctrl Pts',(0.127167851489746,-0.0875735780935426,
-2.28862120985062));
#42338=CARTESIAN_POINT('Ctrl Pts',(0.140736455384675,-0.0410144834475642,
-2.28597211274797));
#42339=CARTESIAN_POINT('Ctrl Pts',(0.154305059279604,0.005544611198413,
-2.28332301564532));
#42340=CARTESIAN_POINT('Ctrl Pts',(0.142478015795887,0.0595046976926254,
-2.28067391854267));
#42341=CARTESIAN_POINT('Ctrl Pts',(0.110679118785195,0.096120083185803,
-2.27802482144002));
#42342=CARTESIAN_POINT('Ctrl Pts',(0.0788802217745042,0.132735468678981,
-2.27537572433737));
#42343=CARTESIAN_POINT('Ctrl Pts',(0.0271094712368389,0.152006153171122,
-2.27272662723472));
#42344=CARTESIAN_POINT('Ctrl Pts',(-0.0208914531046072,0.145094744611551,
-2.27007753013207));
#42345=CARTESIAN_POINT('Ctrl Pts',(-0.0688923774460532,0.138183336051979,
-2.26742843302942));
#42346=CARTESIAN_POINT('Ctrl Pts',(-0.113123475591281,0.105089834440694,
-2.26477933592677));
#42347=CARTESIAN_POINT('Ctrl Pts',(-0.133300696120074,0.0609906725706206,
-2.26213023882412));
#42348=CARTESIAN_POINT('Ctrl Pts',(-0.141970297262714,0.0420424659237912,
-2.26099199407751));
#42349=CARTESIAN_POINT('Ctrl Pts',(-0.146199104167309,0.0210624092175888,
-2.25985374933089));
#42350=CARTESIAN_POINT('Ctrl Pts',(-0.146128142350211,5.51125628420172E-5,
-2.25871550458428));
#42351=CARTESIAN_POINT('Origin',(0.,0.,-1.487));
#42352=CARTESIAN_POINT('',(-0.146247143544926,-0.000124102100222137,-2.20158449541571));
#42353=CARTESIAN_POINT('',(-0.146283306677627,-0.000130979094668964,-2.20871550458428));
#42354=CARTESIAN_POINT('',(-0.14635,-1.79227059055215E-17,-1.487));
#42355=CARTESIAN_POINT('Ctrl Pts',(-0.146247143544926,-0.000124102100222137,
-2.20158449541571));
#42356=CARTESIAN_POINT('Ctrl Pts',(-0.145975220405292,0.0337524727000206,
-2.20342379727535));
#42357=CARTESIAN_POINT('Ctrl Pts',(-0.13426106438023,0.0677987052486075,
-2.205263099135));
#42358=CARTESIAN_POINT('Ctrl Pts',(-0.112739815984817,0.0936945672506367,
-2.20710240099464));
#42359=CARTESIAN_POINT('Ctrl Pts',(-0.081743339538734,0.130991682262237,
-2.20975149809729));
#42360=CARTESIAN_POINT('Ctrl Pts',(-0.0304031603579323,0.151381776383703,
-2.21240059519994));
#42361=CARTESIAN_POINT('Ctrl Pts',(0.0177364986444008,0.145514104664846,
-2.21504969230259));
#42362=CARTESIAN_POINT('Ctrl Pts',(0.0658761576467332,0.139646432945988,
-2.21769878940525));
#42363=CARTESIAN_POINT('Ctrl Pts',(0.110815296470595,0.107520995386807,
-2.2203478865079));
#42364=CARTESIAN_POINT('Ctrl Pts',(0.131945161526139,0.0638702778326173,
-2.22299698361055));
#42365=CARTESIAN_POINT('Ctrl Pts',(0.153075026581682,0.0202195602784276,
-2.2256460807132));
#42366=CARTESIAN_POINT('Ctrl Pts',(0.150395617868907,-0.0349564372707706,
-2.22829517781585));
#42367=CARTESIAN_POINT('Ctrl Pts',(0.125135692221462,-0.0763544142327749,
-2.2309442749185));
#42368=CARTESIAN_POINT('Ctrl Pts',(0.099875766574016,-0.11775239119478,
-2.23359337202115));
#42369=CARTESIAN_POINT('Ctrl Pts',(0.0520353239918985,-0.145372347569591,
-2.2362424691238));
#42370=CARTESIAN_POINT('Ctrl Pts',(0.00355363430999713,-0.146547977549216,
-2.23889156622645));
#42371=CARTESIAN_POINT('Ctrl Pts',(-0.0449280553719036,-0.14772360752884,
-2.2415406633291));
#42372=CARTESIAN_POINT('Ctrl Pts',(-0.094050992153589,-0.12245491111328,
-2.24418976043175));
#42373=CARTESIAN_POINT('Ctrl Pts',(-0.121287763934186,-0.0823299238455837,
-2.2468388575344));
#42374=CARTESIAN_POINT('Ctrl Pts',(-0.137551903616247,-0.0583697275741744,
-2.24842073682817));
#42375=CARTESIAN_POINT('Ctrl Pts',(-0.146011983357597,-0.0291121489472482,
-2.25000261612194));
#42376=CARTESIAN_POINT('Ctrl Pts',(-0.14614553911452,7.41235706846755E-5,
-2.25158449541571));
#42377=CARTESIAN_POINT('Ctrl Pts',(-0.146128142350211,5.51125628420172E-5,
-2.25871550458428));
#42378=CARTESIAN_POINT('Ctrl Pts',(-0.14603395098331,-0.0278289815560796,
-2.25720465222824));
#42379=CARTESIAN_POINT('Ctrl Pts',(-0.138364145592754,-0.0557610687996438,
-2.2556937998722));
#42380=CARTESIAN_POINT('Ctrl Pts',(-0.123448530857947,-0.0790531337502038,
-2.25418294751616));
#42381=CARTESIAN_POINT('Ctrl Pts',(-0.0972958021546651,-0.11989295607209,
-2.25153385041351));
#42382=CARTESIAN_POINT('Ctrl Pts',(-0.0488670018357426,-0.146467778586996,
-2.24888475331086));
#42383=CARTESIAN_POINT('Ctrl Pts',(-0.000371216202019402,-0.146590586073064,
-2.24623565620821));
#42384=CARTESIAN_POINT('Ctrl Pts',(0.0481245694317025,-0.146713393559132,
-2.24358655910556));
#42385=CARTESIAN_POINT('Ctrl Pts',(0.0966873403802246,-0.120384186016363,
-2.24093746200291));
#42386=CARTESIAN_POINT('Ctrl Pts',(0.123046572412074,-0.0796773414739313,
-2.23828836490026));
#42387=CARTESIAN_POINT('Ctrl Pts',(0.149405804443923,-0.0389704969314992,
-2.23563926779761));
#42388=CARTESIAN_POINT('Ctrl Pts',(0.153561497559099,0.0161139846105963,
-2.23299017069496));
#42389=CARTESIAN_POINT('Ctrl Pts',(0.133607881917611,0.0603147711278332,
-2.23034107359231));
#42390=CARTESIAN_POINT('Ctrl Pts',(0.113654266276122,0.10451555764507,-2.22769197648966));
#42391=CARTESIAN_POINT('Ctrl Pts',(0.0695913418779708,0.137832649137449,
-2.22504287938701));
#42392=CARTESIAN_POINT('Ctrl Pts',(0.0216260369183928,0.144987076161696,
-2.22239378228436));
#42393=CARTESIAN_POINT('Ctrl Pts',(-0.0263392680411845,0.152141503185943,
-2.21974468518171));
#42394=CARTESIAN_POINT('Ctrl Pts',(-0.0782069535621885,0.133133265742058,
-2.21709558807905));
#42395=CARTESIAN_POINT('Ctrl Pts',(-0.110190886261694,0.0966793996235781,
-2.2144464909764));
#42396=CARTESIAN_POINT('Ctrl Pts',(-0.133255283421017,0.0703916240067169,
-2.21253616217903));
#42397=CARTESIAN_POINT('Ctrl Pts',(-0.145979720895302,0.0350317633164389,
-2.21062583338166));
#42398=CARTESIAN_POINT('Ctrl Pts',(-0.146283306677627,-0.000130979094668964,
-2.20871550458428));
#42399=CARTESIAN_POINT('Origin',(0.,0.,-1.487));
#42400=CARTESIAN_POINT('',(-0.146589640615231,-1.29382981380044E-5,-2.15158449541571));
#42401=CARTESIAN_POINT('',(-0.146589947336248,1.14350527840421E-5,-2.15871550458428));
#42402=CARTESIAN_POINT('',(-0.14635,-1.79227059055215E-17,-1.487));
#42403=CARTESIAN_POINT('Ctrl Pts',(-0.146589640615231,-1.29382981380044E-5,
-2.15158449541571));
#42404=CARTESIAN_POINT('Ctrl Pts',(-0.146529298073255,0.0477938860680167,
-2.15419588132612));
#42405=CARTESIAN_POINT('Ctrl Pts',(-0.120930624581389,0.0956561308620035,
-2.15680726723653));
#42406=CARTESIAN_POINT('Ctrl Pts',(-0.0811096027371204,0.122107208568541,
-2.15941865314693));
#42407=CARTESIAN_POINT('Ctrl Pts',(-0.0407135229498382,0.148940267993073,
-2.16206775024958));
#42408=CARTESIAN_POINT('Ctrl Pts',(0.0143186428785755,0.153739295064571,
-2.16471684735223));
#42409=CARTESIAN_POINT('Ctrl Pts',(0.0587495543193546,0.134303491793221,
-2.16736594445488));
#42410=CARTESIAN_POINT('Ctrl Pts',(0.103180465760136,0.114867688521869,
-2.17001504155753));
#42411=CARTESIAN_POINT('Ctrl Pts',(0.137010122813282,0.0711970549076663,
-2.17266413866019));
#42412=CARTESIAN_POINT('Ctrl Pts',(0.144724497295698,0.0233186175208184,
-2.17531323576284));
#42413=CARTESIAN_POINT('Ctrl Pts',(0.152438871778113,-0.0245598198660281,
-2.17796233286549));
#42414=CARTESIAN_POINT('Ctrl Pts',(0.1340379636898,-0.0766460610255191,
-2.18061142996814));
#42415=CARTESIAN_POINT('Ctrl Pts',(0.0979602921155994,-0.109053744590459,
-2.18326052707079));
#42416=CARTESIAN_POINT('Ctrl Pts',(0.0618826205413989,-0.141461428155398,
-2.18590962417344));
#42417=CARTESIAN_POINT('Ctrl Pts',(0.00812818548131124,-0.154190554125787,
-2.18855872127609));
#42418=CARTESIAN_POINT('Ctrl Pts',(-0.0386516304278741,-0.141403640355691,
-2.19120781837874));
#42419=CARTESIAN_POINT('Ctrl Pts',(-0.0854314463370593,-0.128616726585596,
-2.19385691548139));
#42420=CARTESIAN_POINT('Ctrl Pts',(-0.125236643095342,-0.0903137730750164,
-2.19650601258404));
#42421=CARTESIAN_POINT('Ctrl Pts',(-0.139812854618803,-0.0440602283688595,
-2.19915510968669));
#42422=CARTESIAN_POINT('Ctrl Pts',(-0.144268616825835,-0.0299211088787746,
-2.1999649049297));
#42423=CARTESIAN_POINT('Ctrl Pts',(-0.146366864005047,-0.0150390487571437,
-2.2007747001727));
#42424=CARTESIAN_POINT('Ctrl Pts',(-0.146247143544926,-0.000124102100222137,
-2.20158449541571));
#42425=CARTESIAN_POINT('Ctrl Pts',(-0.146283306677627,-0.000130979094668964,
-2.20871550458428));
#42426=CARTESIAN_POINT('Ctrl Pts',(-0.146400710317368,-0.013729224410152,
-2.20797673627901));
#42427=CARTESIAN_POINT('Ctrl Pts',(-0.14466051635752,-0.0272979897470232,
-2.20723796797373));
#42428=CARTESIAN_POINT('Ctrl Pts',(-0.140942373732611,-0.040301178808194,
-2.20649919966845));
#42429=CARTESIAN_POINT('Ctrl Pts',(-0.127609748626014,-0.0869283963284094,
-2.2038501025658));
#42430=CARTESIAN_POINT('Ctrl Pts',(-0.088844318534813,-0.126283336575766,
-2.20120100546315));
#42431=CARTESIAN_POINT('Ctrl Pts',(-0.0424236203113571,-0.140318117741049,
-2.1985519083605));
#42432=CARTESIAN_POINT('Ctrl Pts',(0.00399707791210018,-0.154352898906332,
-2.19590281125785));
#42433=CARTESIAN_POINT('Ctrl Pts',(0.0580730442678115,-0.14306752098954,
-2.1932537141552));
#42434=CARTESIAN_POINT('Ctrl Pts',(0.0950054442670761,-0.111637374056938,
-2.19060461705255));
#42435=CARTESIAN_POINT('Ctrl Pts',(0.13193784426634,-0.0802072271243357,
-2.1879555199499));
#42436=CARTESIAN_POINT('Ctrl Pts',(0.151726677909156,-0.0286323111759234,
-2.18530642284725));
#42437=CARTESIAN_POINT('Ctrl Pts',(0.145296933812379,0.0194355023458139,
-2.1826573257446));
#42438=CARTESIAN_POINT('Ctrl Pts',(0.138867189715603,0.0675033158675512,
-2.18000822864195));
#42439=CARTESIAN_POINT('Ctrl Pts',(0.106218867879233,0.112064026962615,
-2.1773591315393));
#42440=CARTESIAN_POINT('Ctrl Pts',(0.0623242449747267,0.132682426172585,
-2.17471003443665));
#42441=CARTESIAN_POINT('Ctrl Pts',(0.0184296220702193,0.153300825382555,
-2.172060937334));
#42442=CARTESIAN_POINT('Ctrl Pts',(-0.0367113019024245,0.149976912707432,
-2.16941184023135));
#42443=CARTESIAN_POINT('Ctrl Pts',(-0.0778113108413852,0.124235009686716,
-2.1667627431287));
#42444=CARTESIAN_POINT('Ctrl Pts',(-0.118911319780345,0.0984931066660002,
-2.16411364602605));
#42445=CARTESIAN_POINT('Ctrl Pts',(-0.145970413685621,0.0503332132996906,
-2.16146454892339));
#42446=CARTESIAN_POINT('Ctrl Pts',(-0.14657949409086,0.00184109716757596,
-2.15881545182074));
#42447=CARTESIAN_POINT('Ctrl Pts',(-0.146587154047055,0.00123124749556039,
-2.15878213607526));
#42448=CARTESIAN_POINT('Ctrl Pts',(-0.146590630604965,0.000621345278386432,
-2.15874882032977));
#42449=CARTESIAN_POINT('Ctrl Pts',(-0.146589947336248,1.14350527840421E-5,
-2.15871550458428));
#42450=CARTESIAN_POINT('Origin',(0.,0.,-1.487));
#42451=CARTESIAN_POINT('',(-0.146285624387341,0.00013129064497696,-2.10158449541571));
#42452=CARTESIAN_POINT('',(-0.146249303190328,0.000124626032094787,-2.10871550458428));
#42453=CARTESIAN_POINT('',(-0.14635,-1.79227059055215E-17,-1.487));
#42454=CARTESIAN_POINT('Ctrl Pts',(-0.146285624387341,0.00013129064497696,
-2.10158449541571));
#42455=CARTESIAN_POINT('Ctrl Pts',(-0.146402750591997,0.0136480875377478,
-2.10231886827423));
#42456=CARTESIAN_POINT('Ctrl Pts',(-0.144683559179741,0.0271356452517675,
-2.10305324113275));
#42457=CARTESIAN_POINT('Ctrl Pts',(-0.141008962074582,0.0400675761086641,
-2.10378761399127));
#42458=CARTESIAN_POINT('Ctrl Pts',(-0.12775361850934,0.0867168226966701,
-2.10643671109392));
#42459=CARTESIAN_POINT('Ctrl Pts',(-0.0890534542095754,0.126135945210629,
-2.10908580819657));
#42460=CARTESIAN_POINT('Ctrl Pts',(-0.0426560756228998,0.140247628332988,
-2.11173490529922));
#42461=CARTESIAN_POINT('Ctrl Pts',(0.0037413029637753,0.154359311455347,
-2.11438400240188));
#42462=CARTESIAN_POINT('Ctrl Pts',(0.0578358958373609,0.143163555186107,
-2.11703309950452));
#42463=CARTESIAN_POINT('Ctrl Pts',(0.0948203265271063,0.111794649772999,
-2.11968219660717));
#42464=CARTESIAN_POINT('Ctrl Pts',(0.131804757216852,0.0804257443598906,
-2.12233129370982));
#42465=CARTESIAN_POINT('Ctrl Pts',(0.151679025722757,0.0288836898029136,
-2.12498039081248));
#42466=CARTESIAN_POINT('Ctrl Pts',(0.145328940871243,-0.0191947124442461,
-2.12762948791513));
#42467=CARTESIAN_POINT('Ctrl Pts',(0.138978856019729,-0.0672731146914066,
-2.13027858501778));
#42468=CARTESIAN_POINT('Ctrl Pts',(0.106404417810795,-0.11188786462875,
-2.13292768212043));
#42469=CARTESIAN_POINT('Ctrl Pts',(0.0625440204359034,-0.132578970988192,
-2.13557677922308));
#42470=CARTESIAN_POINT('Ctrl Pts',(0.0186836230610119,-0.153270077347634,
-2.13822587632573));
#42471=CARTESIAN_POINT('Ctrl Pts',(-0.0364627334798375,-0.150037540129176,
-2.14087497342838));
#42472=CARTESIAN_POINT('Ctrl Pts',(-0.0776053417495988,-0.124363776770017,
-2.14352407053103));
#42473=CARTESIAN_POINT('Ctrl Pts',(-0.118747950019361,-0.0986900134108574,
-2.14617316763368));
#42474=CARTESIAN_POINT('Ctrl Pts',(-0.145886810018034,-0.0505750239109964,
-2.14882226473633));
#42475=CARTESIAN_POINT('Ctrl Pts',(-0.146576243144295,-0.00208398327228049,
-2.15147136183898));
#42476=CARTESIAN_POINT('Ctrl Pts',(-0.14658605756187,-0.00139368960439911,
-2.15150907303122));
#42477=CARTESIAN_POINT('Ctrl Pts',(-0.146590512025769,-0.000703319730076893,
-2.15154678422347));
#42478=CARTESIAN_POINT('Ctrl Pts',(-0.146589640615231,-1.29382981380044E-5,
-2.15158449541571));
#42479=CARTESIAN_POINT('Ctrl Pts',(-0.146589947336248,1.14350527840421E-5,
-2.15871550458428));
#42480=CARTESIAN_POINT('Ctrl Pts',(-0.146536300583162,-0.0478755857641898,
-2.15609972322712));
#42481=CARTESIAN_POINT('Ctrl Pts',(-0.12083905113848,-0.0958119752148835,
-2.15348394186996));
#42482=CARTESIAN_POINT('Ctrl Pts',(-0.0809071538188127,-0.12224144218575,
-2.15086816051279));
#42483=CARTESIAN_POINT('Ctrl Pts',(-0.0404666662363262,-0.149007526509037,
-2.14821906341014));
#42484=CARTESIAN_POINT('Ctrl Pts',(0.0145733758338476,-0.153715356257692,
-2.14556996630749));
#42485=CARTESIAN_POINT('Ctrl Pts',(0.0589720199772672,-0.13420595585336,
-2.14292086920484));
#42486=CARTESIAN_POINT('Ctrl Pts',(0.103370664120688,-0.114696555449027,
-2.14027177210219));
#42487=CARTESIAN_POINT('Ctrl Pts',(0.137127910337354,-0.070969924891706,
-2.13762267499954));
#42488=CARTESIAN_POINT('Ctrl Pts',(0.144762937513227,-0.0230787705316953,
-2.13497357789689));
#42489=CARTESIAN_POINT('Ctrl Pts',(0.152397964689099,0.0248123838283127,
-2.13232448079424));
#42490=CARTESIAN_POINT('Ctrl Pts',(0.133910772824182,0.0768680619910102,
-2.12967538369159));
#42491=CARTESIAN_POINT('Ctrl Pts',(0.0977794500991502,0.109215918551376,
-2.12702628658894));
#42492=CARTESIAN_POINT('Ctrl Pts',(0.0616481273741167,0.141563775111744,
-2.12437718948629));
#42493=CARTESIAN_POINT('Ctrl Pts',(0.00787267378896704,0.154203810069778,
-2.12172809238364));
#42494=CARTESIAN_POINT('Ctrl Pts',(-0.0388858890808203,0.14133939775274,
-2.11907899528099));
#42495=CARTESIAN_POINT('Ctrl Pts',(-0.0856444519506078,0.128474985435702,
-2.11642989817834));
#42496=CARTESIAN_POINT('Ctrl Pts',(-0.125386124105033,0.0901061258435907,
-2.11378080107569));
#42497=CARTESIAN_POINT('Ctrl Pts',(-0.139885671369288,0.0438284915583091,
-2.11113170397303));
#42498=CARTESIAN_POINT('Ctrl Pts',(-0.144293940285014,0.0297587931742726,
-2.11032630417678));
#42499=CARTESIAN_POINT('Ctrl Pts',(-0.146369002652299,0.0149580626372562,
-2.10952090438053));
#42500=CARTESIAN_POINT('Ctrl Pts',(-0.146249303190328,0.000124626032094787,
-2.10871550458428));
#42501=CARTESIAN_POINT('Origin',(0.,0.,-1.487));
#42502=CARTESIAN_POINT('',(-0.146127240320273,-5.3885368266407E-5,-2.05158449541571));
#42503=CARTESIAN_POINT('',(-0.146144311576588,-7.2996660745207E-5,-2.05871550458428));
#42504=CARTESIAN_POINT('',(-0.14635,-1.79227059055215E-17,-1.487));
#42505=CARTESIAN_POINT('Ctrl Pts',(-0.146127240320273,-5.3885368266407E-5,
-2.05158449541571));
#42506=CARTESIAN_POINT('Ctrl Pts',(-0.14603544661587,0.0277495163116801,
-2.05309095232499));
#42507=CARTESIAN_POINT('Ctrl Pts',(-0.138413074264927,0.0555995514695339,
-2.05459740923428));
#42508=CARTESIAN_POINT('Ctrl Pts',(-0.123579356770016,0.078848466192334,
-2.05610386614356));
#42509=CARTESIAN_POINT('Ctrl Pts',(-0.0974943371487333,0.119731568956415,
-2.05875296324621));
#42510=CARTESIAN_POINT('Ctrl Pts',(-0.0491096386046498,0.146386603816594,
-2.06140206034886));
#42511=CARTESIAN_POINT('Ctrl Pts',(-0.000614122693888632,0.146589770768261,
-2.06405115745151));
#42512=CARTESIAN_POINT('Ctrl Pts',(0.0478813932168725,0.146792937719929,
-2.06670025455416));
#42513=CARTESIAN_POINT('Ctrl Pts',(0.0964877264943104,0.120544236763086,
-2.06934935165682));
#42514=CARTESIAN_POINT('Ctrl Pts',(0.12291437554811,0.0798811262075896,
-2.07199844875947));
#42515=CARTESIAN_POINT('Ctrl Pts',(0.149341024601909,0.0392180156520937,
-2.07464754586212));
#42516=CARTESIAN_POINT('Ctrl Pts',(0.153587989432068,-0.0158595045020563,
-2.07729664296477));
#42517=CARTESIAN_POINT('Ctrl Pts',(0.133707643671456,-0.0600932946708818,
-2.07994574006742));
#42518=CARTESIAN_POINT('Ctrl Pts',(0.113827297910845,-0.104327084839708,
-2.08259483717007));
#42519=CARTESIAN_POINT('Ctrl Pts',(0.0698196415594624,-0.13771714502321,
-2.08524393427272));
#42520=CARTESIAN_POINT('Ctrl Pts',(0.0218662572988801,-0.144951042881084,
-2.08789303137537));
#42521=CARTESIAN_POINT('Ctrl Pts',(-0.0260871269617016,-0.152184940738957,
-2.09054212847802));
#42522=CARTESIAN_POINT('Ctrl Pts',(-0.0779862391314823,-0.133262676271201,
-2.09319122558067));
#42523=CARTESIAN_POINT('Ctrl Pts',(-0.110030533801013,-0.0968618587062973,
-2.09584032268332));
#42524=CARTESIAN_POINT('Ctrl Pts',(-0.133191628133265,-0.0705519405730871,
-2.09775504692745));
#42525=CARTESIAN_POINT('Ctrl Pts',(-0.145980242208416,-0.0351109414354531,
-2.09966977117158));
#42526=CARTESIAN_POINT('Ctrl Pts',(-0.146285624387341,0.00013129064497696,
-2.10158449541571));
#42527=CARTESIAN_POINT('Ctrl Pts',(-0.146249303190328,0.000124626032094787,
-2.10871550458428));
#42528=CARTESIAN_POINT('Ctrl Pts',(-0.145975290735094,-0.0338316367344376,
-2.10687180727788));
#42529=CARTESIAN_POINT('Ctrl Pts',(-0.134200066247532,-0.067959289133989,
-2.10502810997148));
#42530=CARTESIAN_POINT('Ctrl Pts',(-0.112584404396465,-0.0938812527260169,
-2.10318441266508));
#42531=CARTESIAN_POINT('Ctrl Pts',(-0.0815261677853019,-0.131126953746614,
-2.10053531556243));
#42532=CARTESIAN_POINT('Ctrl Pts',(-0.0301522721888892,-0.151431946809354,
-2.09788621845978));
#42533=CARTESIAN_POINT('Ctrl Pts',(0.0179775973830789,-0.145484513674291,
-2.09523712135713));
#42534=CARTESIAN_POINT('Ctrl Pts',(0.0661074669550455,-0.139537080539229,
-2.09258802425448));
#42535=CARTESIAN_POINT('Ctrl Pts',(0.110993310502568,-0.107337221206366,
-2.08993892715183));
#42536=CARTESIAN_POINT('Ctrl Pts',(0.132050815251673,-0.0636515507908622,
-2.08728983004918));
#42537=CARTESIAN_POINT('Ctrl Pts',(0.153108320000778,-0.0199658803753582,
-2.08464073294653));
#42538=CARTESIAN_POINT('Ctrl Pts',(0.150337485951465,0.0352056011227862,
-2.08199163584388));
#42539=CARTESIAN_POINT('Ctrl Pts',(0.12500899691422,0.076561664148669,-2.07934253874123));
#42540=CARTESIAN_POINT('Ctrl Pts',(0.0996805078769755,0.117917727174551,
-2.07669344163858));
#42541=CARTESIAN_POINT('Ctrl Pts',(0.0517943638517992,0.145458371728172,
-2.07404434453593));
#42542=CARTESIAN_POINT('Ctrl Pts',(0.00331079301419913,0.146553663810668,
-2.07139524743328));
#42543=CARTESIAN_POINT('Ctrl Pts',(-0.045172777823401,0.147648955893163,
-2.06874615033063));
#42544=CARTESIAN_POINT('Ctrl Pts',(-0.0942537754734231,0.122298895504535,
-2.06609705322797));
#42545=CARTESIAN_POINT('Ctrl Pts',(-0.1214240208077,0.0821288310984904,
-2.06344795612532));
#42546=CARTESIAN_POINT('Ctrl Pts',(-0.137603353415531,0.0582083686621983,
-2.06187047227831));
#42547=CARTESIAN_POINT('Ctrl Pts',(-0.146013216347422,0.0290327890053112,
-2.0602929884313));
#42548=CARTESIAN_POINT('Ctrl Pts',(-0.146144311576588,-7.2996660745207E-5,
-2.05871550458428));
#42549=CARTESIAN_POINT('Origin',(0.,0.,-1.487));
#42550=CARTESIAN_POINT('',(-0.146483524170368,-0.000107783910021919,-2.00158449541571));
#42551=CARTESIAN_POINT('',(-0.14651679492655,-9.2174979582009E-5,-2.00871550458428));
#42552=CARTESIAN_POINT('',(-0.14635,-1.79227059055215E-17,-1.487));
#42553=CARTESIAN_POINT('Ctrl Pts',(-0.146483524170368,-0.000107783910021919,
-2.00158449541571));
#42554=CARTESIAN_POINT('Ctrl Pts',(-0.146138605468356,0.0416854145126164,
-2.00386303637576));
#42555=CARTESIAN_POINT('Ctrl Pts',(-0.127337547382231,0.0837496555319783,
-2.0061415773358));
#42556=CARTESIAN_POINT('Ctrl Pts',(-0.0957536860156155,0.110996259644177,
-2.00842011829585));
#42557=CARTESIAN_POINT('Ctrl Pts',(-0.0590333824951295,0.142673943423525,
-2.0110692153985));
#42558=CARTESIAN_POINT('Ctrl Pts',(-0.00503449370253807,0.154322546162233,
-2.01371831250115));
#42559=CARTESIAN_POINT('Ctrl Pts',(0.0414794930685156,0.140600105602213,
-2.0163674096038));
#42560=CARTESIAN_POINT('Ctrl Pts',(0.0879934798395713,0.126877665042193,
-2.01901650670646));
#42561=CARTESIAN_POINT('Ctrl Pts',(0.127022564589087,0.0877841811834399,
-2.0216656038091));
#42562=CARTESIAN_POINT('Ctrl Pts',(0.140668300406616,0.041247633887154,
-2.02431470091175));
#42563=CARTESIAN_POINT('Ctrl Pts',(0.154314036224144,-0.00528891340913192,
-2.02696379801441));
#42564=CARTESIAN_POINT('Ctrl Pts',(0.142576423109686,-0.0592685241429521,
-2.02961289511706));
#42565=CARTESIAN_POINT('Ctrl Pts',(0.110838242815177,-0.0959365517944979,
-2.03226199221971));
#42566=CARTESIAN_POINT('Ctrl Pts',(0.0791000625206695,-0.132604579446043,
-2.03491108932236));
#42567=CARTESIAN_POINT('Ctrl Pts',(0.0273613150461139,-0.151961024015315,
-2.03756018642501));
#42568=CARTESIAN_POINT('Ctrl Pts',(-0.0206509962511345,-0.145129164520472,
-2.04020928352766));
#42569=CARTESIAN_POINT('Ctrl Pts',(-0.0686633075483823,-0.138297305025629,
-2.04285838063031));
#42570=CARTESIAN_POINT('Ctrl Pts',(-0.112949182668323,-0.105277141466672,
-2.04550747773296));
#42571=CARTESIAN_POINT('Ctrl Pts',(-0.133199449879051,-0.0612114743532014,
-2.04815657483561));
#42572=CARTESIAN_POINT('Ctrl Pts',(-0.141934036926929,-0.0422045446559245,
-2.04929921502898));
#42573=CARTESIAN_POINT('Ctrl Pts',(-0.146196865395841,-0.0211426294777117,
-2.05044185522234));
#42574=CARTESIAN_POINT('Ctrl Pts',(-0.146127240320273,-5.3885368266407E-5,
-2.05158449541571));
#42575=CARTESIAN_POINT('Ctrl Pts',(-0.146144311576588,-7.2996660745207E-5,
-2.05871550458428));
#42576=CARTESIAN_POINT('Ctrl Pts',(-0.146233366932427,-0.0198450823112631,
-2.05764389132865));
#42577=CARTESIAN_POINT('Ctrl Pts',(-0.142501994378041,-0.0395849599182529,
-2.05657227807301));
#42578=CARTESIAN_POINT('Ctrl Pts',(-0.134790535627584,-0.057623339298778,
-2.05550066481737));
#42579=CARTESIAN_POINT('Ctrl Pts',(-0.115727312094663,-0.102215376866536,
-2.05285156771472));
#42580=CARTESIAN_POINT('Ctrl Pts',(-0.0723413720102935,-0.136409383578594,
-2.05020247061207));
#42581=CARTESIAN_POINT('Ctrl Pts',(-0.0245291836171625,-0.144524243218183,
-2.04755337350942));
#42582=CARTESIAN_POINT('Ctrl Pts',(0.0232830047759706,-0.152639102857773,
-2.04490427640677));
#42583=CARTESIAN_POINT('Ctrl Pts',(0.0755214414778657,-0.134674815424893,
-2.04225517930412));
#42584=CARTESIAN_POINT('Ctrl Pts',(0.108229969381733,-0.0988696690312163,
-2.03960608220147));
#42585=CARTESIAN_POINT('Ctrl Pts',(0.140938497285599,-0.0630645226375404,
-2.03695698509882));
#42586=CARTESIAN_POINT('Ctrl Pts',(0.154117116391439,-0.00941851728306658,
-2.03430788799617));
#42587=CARTESIAN_POINT('Ctrl Pts',(0.141722210356908,0.0374666894489691,
-2.03165879089352));
#42588=CARTESIAN_POINT('Ctrl Pts',(0.129327304322376,0.0843518961810062,
-2.02900969379087));
#42589=CARTESIAN_POINT('Ctrl Pts',(0.0913588731474758,0.124476304290605,
-2.02636059668822));
#42590=CARTESIAN_POINT('Ctrl Pts',(0.0452289559312077,0.139439159751076,
-2.02371149958557));
#42591=CARTESIAN_POINT('Ctrl Pts',(-0.000900961285057872,0.154402015211546,
-2.02106240248292));
#42592=CARTESIAN_POINT('Ctrl Pts',(-0.0551923645426887,0.144203318022889,
-2.01841330538027));
#42593=CARTESIAN_POINT('Ctrl Pts',(-0.0927476215980198,0.113520114581618,
-2.01576420827762));
#42594=CARTESIAN_POINT('Ctrl Pts',(-0.126056565344061,0.0863062122544981,
-2.01341464037984));
#42595=CARTESIAN_POINT('Ctrl Pts',(-0.146200059172505,0.0429782214212413,
-2.01106507248206));
#42596=CARTESIAN_POINT('Ctrl Pts',(-0.14651679492655,-9.2174979582009E-5,
-2.00871550458428));
#42597=CARTESIAN_POINT('Origin',(0.,0.,-1.487));
#42598=CARTESIAN_POINT('',(-0.146467901202366,0.000113550927785495,-1.95158449541571));
#42599=CARTESIAN_POINT('',(-0.146430225588029,0.000124228536857034,-1.95871550458428));
#42600=CARTESIAN_POINT('',(-0.14635,-1.79227059055215E-17,-1.487));
#42601=CARTESIAN_POINT('Ctrl Pts',(-0.146467901202366,0.000113550927785495,
-1.95158449541571));
#42602=CARTESIAN_POINT('Ctrl Pts',(-0.146530905875648,0.00748045608225115,
-1.95198602332387));
#42603=CARTESIAN_POINT('Ctrl Pts',(-0.146023230868662,0.0148386496320622,
-1.95238755123203));
#42604=CARTESIAN_POINT('Ctrl Pts',(-0.144914795699676,0.0221052036384111,
-1.95278907914019));
#42605=CARTESIAN_POINT('Ctrl Pts',(-0.137601848492386,0.0700465964363302,
-1.95543817624284));
#42606=CARTESIAN_POINT('Ctrl Pts',(-0.104139279699996,0.11399914387574,
-1.95808727334549));
#42607=CARTESIAN_POINT('Ctrl Pts',(-0.0598727735695639,0.133806535810708,
-1.96073637044814));
#42608=CARTESIAN_POINT('Ctrl Pts',(-0.0156062674391309,0.153613927745677,
-1.96338546755079));
#42609=CARTESIAN_POINT('Ctrl Pts',(0.0394641760293445,0.149276164176203,
-1.96603456465344));
#42610=CARTESIAN_POINT('Ctrl Pts',(0.0800836625671089,0.122782511093445,
-1.96868366175609));
#42611=CARTESIAN_POINT('Ctrl Pts',(0.120703149104873,0.0962888580106879,
-1.97133275885874));
#42612=CARTESIAN_POINT('Ctrl Pts',(0.146871678711927,0.0476393154146473,
-1.9739818559614));
#42613=CARTESIAN_POINT('Ctrl Pts',(0.146588559060938,-0.000855799633410346,
-1.97663095306405));
#42614=CARTESIAN_POINT('Ctrl Pts',(0.146305439409949,-0.049350914681468,
-1.9792800501667));
#42615=CARTESIAN_POINT('Ctrl Pts',(0.119570670500917,-0.0976916021815428,
-1.98192914726935));
#42616=CARTESIAN_POINT('Ctrl Pts',(0.0786446177780337,-0.123709183713747,
-1.984578244372));
#42617=CARTESIAN_POINT('Ctrl Pts',(0.0377185650551491,-0.149726765245952,
-1.98722734147465));
#42618=CARTESIAN_POINT('Ctrl Pts',(-0.0173987714815884,-0.153421240810284,
-1.9898764385773));
#42619=CARTESIAN_POINT('Ctrl Pts',(-0.0614309927523799,-0.13309835149254,
-1.99252553567995));
#42620=CARTESIAN_POINT('Ctrl Pts',(-0.10546321402317,-0.112775462174795,
-1.9951746327826));
#42621=CARTESIAN_POINT('Ctrl Pts',(-0.138410320028015,-0.0684352079749748,
-1.99782372988525));
#42622=CARTESIAN_POINT('Ctrl Pts',(-0.145163013906248,-0.0204116984650692,
-2.0004728269879));
#42623=CARTESIAN_POINT('Ctrl Pts',(-0.146107581847224,-0.0136941619804954,
-2.0008433831305));
#42624=CARTESIAN_POINT('Ctrl Pts',(-0.146539617848722,-0.00690455722508045,
-2.00121393927311));
#42625=CARTESIAN_POINT('Ctrl Pts',(-0.146483524170368,-0.000107783910021919,
-2.00158449541571));
#42626=CARTESIAN_POINT('Ctrl Pts',(-0.14651679492655,-9.2174979582009E-5,
-2.00871550458428));
#42627=CARTESIAN_POINT('Ctrl Pts',(-0.146557173248306,-0.00558290440251719,
-2.00841597537941));
#42628=CARTESIAN_POINT('Ctrl Pts',(-0.14627533041133,-0.0110694474437864,
-2.00811644617454));
#42629=CARTESIAN_POINT('Ctrl Pts',(-0.145657465336476,-0.0165178848060591,
-2.00781691696966));
#42630=CARTESIAN_POINT('Ctrl Pts',(-0.140192941166569,-0.0647049710585717,
-2.00516781986701));
#42631=CARTESIAN_POINT('Ctrl Pts',(-0.108444781973725,-0.109911433869707,
-2.00251872276436));
#42632=CARTESIAN_POINT('Ctrl Pts',(-0.0649724565608736,-0.131405926864653,
-1.99986962566171));
#42633=CARTESIAN_POINT('Ctrl Pts',(-0.0215001311480229,-0.152900419859598,
-1.99722052855906));
#42634=CARTESIAN_POINT('Ctrl Pts',(0.0336963604848347,-0.150682943038354,
-1.99457143145641));
#42635=CARTESIAN_POINT('Ctrl Pts',(0.0753043193217198,-0.125770414717475,
-1.99192233435376));
#42636=CARTESIAN_POINT('Ctrl Pts',(0.116912278158607,-0.100857886396594,
-1.98927323725111));
#42637=CARTESIAN_POINT('Ctrl Pts',(0.144931704199522,-0.053250306576076,
-1.98662414014846));
#42638=CARTESIAN_POINT('Ctrl Pts',(0.146513097829673,-0.00478015596668234,
-1.98397504304581));
#42639=CARTESIAN_POINT('Ctrl Pts',(0.148094491459823,0.0436899946427065,
-1.98132594594316));
#42640=CARTESIAN_POINT('Ctrl Pts',(0.123237852679217,0.093022716040971,
-1.97867684884051));
#42641=CARTESIAN_POINT('Ctrl Pts',(0.0833422504755588,0.12059439046814,
-1.97602775173786));
#42642=CARTESIAN_POINT('Ctrl Pts',(0.0434466482718983,0.148166064895312,
-1.97337865463521));
#42643=CARTESIAN_POINT('Ctrl Pts',(-0.0114879173548165,0.153976692351384,
-1.97072955753256));
#42644=CARTESIAN_POINT('Ctrl Pts',(-0.0562688646997204,0.135361562461866,
-1.96808046042991));
#42645=CARTESIAN_POINT('Ctrl Pts',(-0.101049812044625,0.116746432572348,
-1.96543136332725));
#42646=CARTESIAN_POINT('Ctrl Pts',(-0.135677141107718,0.0737055453372412,
-1.9627822662246));
#42647=CARTESIAN_POINT('Ctrl Pts',(-0.14427101727684,0.0259771303384112,
-1.96013316912195));
#42648=CARTESIAN_POINT('Ctrl Pts',(-0.145804021795487,0.017463175235828,
-1.95966061427606));
#42649=CARTESIAN_POINT('Ctrl Pts',(-0.146508625607797,0.00880006007651845,
-1.95918805943017));
#42650=CARTESIAN_POINT('Ctrl Pts',(-0.146430225588029,0.000124228536857034,
-1.95871550458428));
#42651=CARTESIAN_POINT('Origin',(0.,0.,-1.487));
#42652=CARTESIAN_POINT('',(-0.146121465979963,4.50978529691337E-5,-1.90158449541571));
#42653=CARTESIAN_POINT('',(-0.146112202146807,2.42034320618872E-5,-1.90871550458428));
#42654=CARTESIAN_POINT('',(-0.14635,-1.79227059055215E-17,-1.487));
#42655=CARTESIAN_POINT('Ctrl Pts',(-0.146121465979963,4.50978529691337E-5,
-1.90158449541571));
#42656=CARTESIAN_POINT('Ctrl Pts',(-0.146181182134258,0.0217075988651919,
-1.90275810737463));
#42657=CARTESIAN_POINT('Ctrl Pts',(-0.141674343543634,0.04334647161387,
-1.90393171933356));
#42658=CARTESIAN_POINT('Ctrl Pts',(-0.132475676519681,0.0627625140607628,
-1.90510533129248));
#42659=CARTESIAN_POINT('Ctrl Pts',(-0.111712287073873,0.106588739074822,
-1.90775442839513));
#42660=CARTESIAN_POINT('Ctrl Pts',(-0.0670438933564559,0.139089578130225,
-1.91040352549778));
#42661=CARTESIAN_POINT('Ctrl Pts',(-0.0189550872725999,0.145360389057895,
-1.91305262260043));
#42662=CARTESIAN_POINT('Ctrl Pts',(0.029133718811256,0.151631199985565,
-1.91570171970308));
#42663=CARTESIAN_POINT('Ctrl Pts',(0.0806429372615497,0.131671982785502,
-1.91835081680573));
#42664=CARTESIAN_POINT('Ctrl Pts',(0.111950825017996,0.0946358854682761,
-1.92099991390838));
#42665=CARTESIAN_POINT('Ctrl Pts',(0.14325871277444,0.0575997881510518,
-1.92364901101104));
#42666=CARTESIAN_POINT('Ctrl Pts',(0.154365269837039,0.00348681071666326,
-1.92629810811369));
#42667=CARTESIAN_POINT('Ctrl Pts',(0.140177112048345,-0.0428872393417926,
-1.92894720521634));
#42668=CARTESIAN_POINT('Ctrl Pts',(0.125988954259651,-0.0892612894002504,
-1.93159630231899));
#42669=CARTESIAN_POINT('Ctrl Pts',(0.0865060816196672,-0.127896412082776,
-1.93424539942164));
#42670=CARTESIAN_POINT('Ctrl Pts',(0.0398350447778369,-0.141074828541885,
-1.93689449652429));
#42671=CARTESIAN_POINT('Ctrl Pts',(-0.00683599206399215,-0.154253245000994,
-1.93954359362694));
#42672=CARTESIAN_POINT('Ctrl Pts',(-0.0606951931076668,-0.141974955236685,
-1.94219269072959));
#42673=CARTESIAN_POINT('Ctrl Pts',(-0.0970431308184098,-0.109870691276316,
-1.94484178783224));
#42674=CARTESIAN_POINT('Ctrl Pts',(-0.127881753155114,-0.082632522234911,
-1.94708935702673));
#42675=CARTESIAN_POINT('Ctrl Pts',(-0.146115229918752,-0.0411230075962279,
-1.94933692622122));
#42676=CARTESIAN_POINT('Ctrl Pts',(-0.146467901202366,0.000113550927785495,
-1.95158449541571));
#42677=CARTESIAN_POINT('Ctrl Pts',(-0.146430225588029,0.000124228536857034,
-1.95871550458428));
#42678=CARTESIAN_POINT('Ctrl Pts',(-0.146069122623071,-0.0398358186890666,
-1.95653896232752));
#42679=CARTESIAN_POINT('Ctrl Pts',(-0.129097100987133,-0.0800656356800447,
-1.95436242007076));
#42680=CARTESIAN_POINT('Ctrl Pts',(-0.0999499468002784,-0.10723313788813,
-1.952185877814));
#42681=CARTESIAN_POINT('Ctrl Pts',(-0.0644745768794416,-0.140299048353297,
-1.94953678071135));
#42682=CARTESIAN_POINT('Ctrl Pts',(-0.0109634137626148,-0.154014926521079,
-1.9468876836087));
#42683=CARTESIAN_POINT('Ctrl Pts',(0.0360437226105418,-0.142090773054014,
-1.94423858650605));
#42684=CARTESIAN_POINT('Ctrl Pts',(0.0830508589836977,-0.13016661958695,
-1.9415894894034));
#42685=CARTESIAN_POINT('Ctrl Pts',(0.123553968613184,-0.0926024344850394,
-1.93894039230075));
#42686=CARTESIAN_POINT('Ctrl Pts',(0.138978627782331,-0.0466248726159469,
-1.9362912951981));
#42687=CARTESIAN_POINT('Ctrl Pts',(0.154403286951479,-0.000647310746854889,
-1.93364219809545));
#42688=CARTESIAN_POINT('Ctrl Pts',(0.144749495660286,0.0537436278894195,
-1.9309931009928));
#42689=CARTESIAN_POINT('Ctrl Pts',(0.114444410528462,0.0916046648676035,
-1.92834400389015));
#42690=CARTESIAN_POINT('Ctrl Pts',(0.0841393253966373,0.129465701845788,
-1.9256949067875));
#42691=CARTESIAN_POINT('Ctrl Pts',(0.033182946424181,0.150796837165882,
-1.92304580968485));
#42692=CARTESIAN_POINT('Ctrl Pts',(-0.0150565113861619,0.145815771408965,
-1.9203967125822));
#42693=CARTESIAN_POINT('Ctrl Pts',(-0.0632959691965042,0.140834705652047,
-1.91774761547955));
#42694=CARTESIAN_POINT('Ctrl Pts',(-0.108818505844733,0.109541438818118,
-1.91509851837689));
#42695=CARTESIAN_POINT('Ctrl Pts',(-0.130747825853863,0.0662868294701219,
-1.91244942127424));
#42696=CARTESIAN_POINT('Ctrl Pts',(-0.141050990895727,0.0459642942183122,
-1.91120478237759));
#42697=CARTESIAN_POINT('Ctrl Pts',(-0.146146070039581,0.0230013517587152,
-1.90996014348094));
#42698=CARTESIAN_POINT('Ctrl Pts',(-0.146112202146807,2.42034320618872E-5,
-1.90871550458428));
#42699=CARTESIAN_POINT('Origin',(0.,0.,-1.487));
#42700=CARTESIAN_POINT('',(-0.146302162622722,-0.00013309729056632,-1.85158449541571));
#42701=CARTESIAN_POINT('',(-0.146341186202789,-0.000134609574743057,-1.85871550458428));
#42702=CARTESIAN_POINT('',(-0.14635,-1.79227059055215E-17,-1.487));
#42703=CARTESIAN_POINT('Ctrl Pts',(-0.146302162622722,-0.00013309729056632,
-1.85158449541571));
#42704=CARTESIAN_POINT('Ctrl Pts',(-0.145984741937988,0.0356689174518258,
-1.8535301914254));
#42705=CARTESIAN_POINT('Ctrl Pts',(-0.132738385200244,0.071681077496235,
-1.85547588743509));
#42706=CARTESIAN_POINT('Ctrl Pts',(-0.108892092441933,0.0981399523343686,
-1.85742158344477));
#42707=CARTESIAN_POINT('Ctrl Pts',(-0.0764249728402753,0.134164145386161,
-1.86007068054742));
#42708=CARTESIAN_POINT('Ctrl Pts',(-0.0243084654917135,0.15247915557962,
-1.86271977765007));
#42709=CARTESIAN_POINT('Ctrl Pts',(0.0235571883881887,0.144685855963249,
-1.86536887475272));
#42710=CARTESIAN_POINT('Ctrl Pts',(0.0714228422680896,0.136892556346878,
-1.86801797185537));
#42711=CARTESIAN_POINT('Ctrl Pts',(0.115037642679331,0.102990946920679,
-1.87066706895803));
#42712=CARTESIAN_POINT('Ctrl Pts',(0.134400167741787,0.0585280526888954,
-1.87331616606068));
#42713=CARTESIAN_POINT('Ctrl Pts',(0.153762692804244,0.0140651584571082,
-1.87596526316333));
#42714=CARTESIAN_POINT('Ctrl Pts',(0.148872942517911,-0.0409590205802653,
-1.87861436026598));
#42715=CARTESIAN_POINT('Ctrl Pts',(0.121973319861668,-0.0813108066772044,
-1.88126345736863));
#42716=CARTESIAN_POINT('Ctrl Pts',(0.0950736972054269,-0.121662592774141,
-1.88391255447128));
#42717=CARTESIAN_POINT('Ctrl Pts',(0.0461642021792778,-0.147341985930645,
-1.88656165157393));
#42718=CARTESIAN_POINT('Ctrl Pts',(-0.00232563591163342,-0.146572608144159,
-1.88921074867658));
#42719=CARTESIAN_POINT('Ctrl Pts',(-0.0508154740025447,-0.145803230357672,
-1.89185984577923));
#42720=CARTESIAN_POINT('Ctrl Pts',(-0.0988856551582181,-0.118585081628195,
-1.89450894288188));
#42721=CARTESIAN_POINT('Ctrl Pts',(-0.124491553148954,-0.0774002017770997,
-1.89715803998453));
#42722=CARTESIAN_POINT('Ctrl Pts',(-0.138753439600492,-0.0544611867045152,
-1.89863352512826));
#42723=CARTESIAN_POINT('Ctrl Pts',(-0.146046389803521,-0.0271893710670532,
-1.90010901027198));
#42724=CARTESIAN_POINT('Ctrl Pts',(-0.146121465979963,4.50978529691337E-5,
-1.90158449541571));
#42725=CARTESIAN_POINT('Ctrl Pts',(-0.146112202146807,2.42034320618872E-5,
-1.90871550458428));
#42726=CARTESIAN_POINT('Ctrl Pts',(-0.146073985407756,-0.0259033524273363,
-1.90731104637829));
#42727=CARTESIAN_POINT('Ctrl Pts',(-0.139505077963029,-0.0518489966240254,
-1.90590658817229));
#42728=CARTESIAN_POINT('Ctrl Pts',(-0.12651918653732,-0.0740394027842464,
-1.90450212996629));
#42729=CARTESIAN_POINT('Ctrl Pts',(-0.102025123841615,-0.115895073828558,
-1.90185303286364));
#42730=CARTESIAN_POINT('Ctrl Pts',(-0.0547008950801745,-0.144390464055115,
-1.89920393576099));
#42731=CARTESIAN_POINT('Ctrl Pts',(-0.00624903828330516,-0.14645780022671,
-1.89655483865834));
#42732=CARTESIAN_POINT('Ctrl Pts',(0.0422028185135615,-0.148525136398304,
-1.89390574155569));
#42733=CARTESIAN_POINT('Ctrl Pts',(0.0917823033458551,-0.124164418514939,
-1.89125664445304));
#42734=CARTESIAN_POINT('Ctrl Pts',(0.11975263458487,-0.0845472899429408,
-1.88860754735039));
#42735=CARTESIAN_POINT('Ctrl Pts',(0.147722965823886,-0.0449301613709413,
-1.88595845024774));
#42736=CARTESIAN_POINT('Ctrl Pts',(0.15408414346962,0.00994337788969538,
-1.88330935314509));
#42737=CARTESIAN_POINT('Ctrl Pts',(0.13591897894051,0.0549087323700171,
-1.88066025604244));
#42738=CARTESIAN_POINT('Ctrl Pts',(0.117753814411401,0.0998740868503387,
-1.87801115893979));
#42739=CARTESIAN_POINT('Ctrl Pts',(0.0750623077074499,0.134931256550348,
-1.87536206183714));
#42740=CARTESIAN_POINT('Ctrl Pts',(0.0274224651070917,0.144003285150594,
-1.87271296473449));
#42741=CARTESIAN_POINT('Ctrl Pts',(-0.0202173774932664,0.153075313750841,
-1.87006386763184));
#42742=CARTESIAN_POINT('Ctrl Pts',(-0.0728055559900301,0.136162201251325,
-1.86741477052919));
#42743=CARTESIAN_POINT('Ctrl Pts',(-0.106225524300139,0.101020174786394,
-1.86476567342654));
#42744=CARTESIAN_POINT('Ctrl Pts',(-0.131667708705355,0.0742670100497515,
-1.86274895047912));
#42745=CARTESIAN_POINT('Ctrl Pts',(-0.146000808165931,0.0369491367817265,
-1.8607322275317));
#42746=CARTESIAN_POINT('Ctrl Pts',(-0.146341186202789,-0.000134609574743057,
-1.85871550458428));
#42747=CARTESIAN_POINT('Origin',(0.,0.,-1.487));
#42748=CARTESIAN_POINT('',(-0.146586453393407,2.34618399145015E-5,-1.80158449541571));
#42749=CARTESIAN_POINT('',(-0.146572905486282,4.68275666195741E-5,-1.80871550458428));
#42750=CARTESIAN_POINT('',(-0.14635,-1.79227059055215E-17,-1.487));
#42751=CARTESIAN_POINT('Ctrl Pts',(-0.146586453393407,2.34618399145015E-5,
-1.80158449541571));
#42752=CARTESIAN_POINT('Ctrl Pts',(-0.146589249888724,0.00128091906965625,
-1.80165317837351));
#42753=CARTESIAN_POINT('Ctrl Pts',(-0.146574472401979,0.00253830888863432,
-1.80172186133131));
#42754=CARTESIAN_POINT('Ctrl Pts',(-0.14654191962176,0.00379523835145167,
-1.80179054428911));
#42755=CARTESIAN_POINT('Ctrl Pts',(-0.145286361059294,0.0522749239213617,
-1.80443964139176));
#42756=CARTESIAN_POINT('Ctrl Pts',(-0.117587569244064,0.100069765364511,
-1.80708873849441));
#42757=CARTESIAN_POINT('Ctrl Pts',(-0.0761480033285232,0.125261405187926,
-1.80973783559706));
#42758=CARTESIAN_POINT('Ctrl Pts',(-0.0347084374129826,0.150453045011341,
-1.81238693269971));
#42759=CARTESIAN_POINT('Ctrl Pts',(0.0204719026028683,0.153041483215024,
-1.81503602980236));
#42760=CARTESIAN_POINT('Ctrl Pts',(0.0640877247140375,0.131839681361691,
-1.81768512690501));
#42761=CARTESIAN_POINT('Ctrl Pts',(0.107703546825207,0.110637879508359,
-1.82033422400766));
#42762=CARTESIAN_POINT('Ctrl Pts',(0.139754851031694,0.0656458375980124,
-1.82298332111031));
#42763=CARTESIAN_POINT('Ctrl Pts',(0.145543148490318,0.0174965701810349,
-1.82563241821297));
#42764=CARTESIAN_POINT('Ctrl Pts',(0.151331445948941,-0.0306526972359428,
-1.82828151531562));
#42765=CARTESIAN_POINT('Ctrl Pts',(0.130856736659701,-0.0819591901595512,
-1.83093061241827));
#42766=CARTESIAN_POINT('Ctrl Pts',(0.0935085694570671,-0.112894133942679,
-1.83357970952092));
#42767=CARTESIAN_POINT('Ctrl Pts',(0.0561604022544324,-0.143829077725807,
-1.83622880662357));
#42768=CARTESIAN_POINT('Ctrl Pts',(0.00193877713840383,-0.154392472368453,
-1.83887790372622));
#42769=CARTESIAN_POINT('Ctrl Pts',(-0.0442906733821896,-0.139740023944204,
-1.84152700082887));
#42770=CARTESIAN_POINT('Ctrl Pts',(-0.0905201239027831,-0.125087575519956,
-1.84417609793152));
#42771=CARTESIAN_POINT('Ctrl Pts',(-0.128757399827941,-0.0852192840288131,
-1.84682519503417));
#42772=CARTESIAN_POINT('Ctrl Pts',(-0.141467171863142,-0.0384184503281782,
-1.84947429213682));
#42773=CARTESIAN_POINT('Ctrl Pts',(-0.144841932090664,-0.0259916662953639,
-1.85017769322978));
#42774=CARTESIAN_POINT('Ctrl Pts',(-0.146416915418359,-0.0130761141722773,
-1.85088109432275));
#42775=CARTESIAN_POINT('Ctrl Pts',(-0.146302162622722,-0.00013309729056632,
-1.85158449541571));
#42776=CARTESIAN_POINT('Ctrl Pts',(-0.146341186202789,-0.000134609574743057,
-1.85871550458428));
#42777=CARTESIAN_POINT('Ctrl Pts',(-0.146447916913517,-0.0117627823017354,
-1.85808313042905));
#42778=CARTESIAN_POINT('Ctrl Pts',(-0.145178839300704,-0.0233679349353573,
-1.85745075627382));
#42779=CARTESIAN_POINT('Ctrl Pts',(-0.14244504878576,-0.0346171316422315,
-1.85681838211858));
#42780=CARTESIAN_POINT('Ctrl Pts',(-0.130992846837817,-0.0817414711755775,
-1.85416928501593));
#42781=CARTESIAN_POINT('Ctrl Pts',(-0.0938366848184793,-0.122619209811925,
-1.85152018791328));
#42782=CARTESIAN_POINT('Ctrl Pts',(-0.0480161012556727,-0.138504121768697,
-1.84887109081063));
#42783=CARTESIAN_POINT('Ctrl Pts',(-0.00219551769286602,-0.154389033725469,
-1.84622199370798));
#42784=CARTESIAN_POINT('Ctrl Pts',(0.0522894874134106,-0.145281119002665,
-1.84357289660533));
#42785=CARTESIAN_POINT('Ctrl Pts',(0.0904524974569562,-0.115357199300748,
-1.84092379950268));
#42786=CARTESIAN_POINT('Ctrl Pts',(0.128615507500503,-0.08543327959883,
-1.83827470240003));
#42787=CARTESIAN_POINT('Ctrl Pts',(0.150456522481318,-0.0346933549178013,
-1.83562560529738));
#42788=CARTESIAN_POINT('Ctrl Pts',(0.145959415974372,0.0135936240617936,
-1.83297650819473));
#42789=CARTESIAN_POINT('Ctrl Pts',(0.141462309467426,0.0618806030413885,
-1.83032741109208));
#42790=CARTESIAN_POINT('Ctrl Pts',(0.110627081472717,0.107714636319548,
-1.82767831398943));
#42791=CARTESIAN_POINT('Ctrl Pts',(0.0675945373608278,0.13007657839015,
-1.82502921688678));
#42792=CARTESIAN_POINT('Ctrl Pts',(0.0245619932489395,0.152438520460751,
-1.82238011978413));
#42793=CARTESIAN_POINT('Ctrl Pts',(-0.0306678669801303,0.151328371323796,
-1.81973102268148));
#42794=CARTESIAN_POINT('Ctrl Pts',(-0.072767041721279,0.127255237086128,
-1.81708192557883));
#42795=CARTESIAN_POINT('Ctrl Pts',(-0.114866216462428,0.103182102848461,
-1.81443282847617));
#42796=CARTESIAN_POINT('Ctrl Pts',(-0.143834705715656,0.0561459835100795,
-1.81178373137352));
#42797=CARTESIAN_POINT('Ctrl Pts',(-0.146387776561852,0.0077172922706412,
-1.80913463427087));
#42798=CARTESIAN_POINT('Ctrl Pts',(-0.146522422158967,0.00516322681681316,
-1.80899492437534));
#42799=CARTESIAN_POINT('Ctrl Pts',(-0.146583596735172,0.00260528810693123,
-1.80885521447981));
#42800=CARTESIAN_POINT('Ctrl Pts',(-0.146572905486282,4.68275666195741E-5,
-1.80871550458428));
#42801=CARTESIAN_POINT('Origin',(0.,0.,-1.487));
#42802=CARTESIAN_POINT('',(-0.146232247576531,0.000120056641797081,-1.75158449541571));
#42803=CARTESIAN_POINT('',(-0.146200518682322,0.000108553130818545,-1.75871550458428));
#42804=CARTESIAN_POINT('',(-0.14635,-1.79227059055215E-17,-1.487));
#42805=CARTESIAN_POINT('Ctrl Pts',(-0.146232247576531,0.000120056641797081,
-1.75158449541571));
#42806=CARTESIAN_POINT('Ctrl Pts',(-0.146351639518327,0.0156094297883246,
-1.75242526242427));
#42807=CARTESIAN_POINT('Ctrl Pts',(-0.144086148722195,0.031064779006721,
-1.75326602943284));
#42808=CARTESIAN_POINT('Ctrl Pts',(-0.139288885238194,0.0456896540770004,
-1.7541067964414));
#42809=CARTESIAN_POINT('Ctrl Pts',(-0.124173619455077,0.091769856773679,
-1.75675589354405));
#42810=CARTESIAN_POINT('Ctrl Pts',(-0.0839239177960128,0.129605441253845,
-1.7594049906467));
#42811=CARTESIAN_POINT('Ctrl Pts',(-0.036997992974151,0.141845290920986,
-1.76205408774935));
#42812=CARTESIAN_POINT('Ctrl Pts',(0.00992793184771074,0.154085140588127,
-1.764703184852));
#42813=CARTESIAN_POINT('Ctrl Pts',(0.0635300798323712,0.140729255442244,
-1.76735228195465));
#42814=CARTESIAN_POINT('Ctrl Pts',(0.0992269060589921,0.107902544708336,
-1.7700013790573));
#42815=CARTESIAN_POINT('Ctrl Pts',(0.134923732285611,0.0750758339744305,
-1.77265047615995));
#42816=CARTESIAN_POINT('Ctrl Pts',(0.152715236754193,0.0227782976525062,
-1.77529957326261));
#42817=CARTESIAN_POINT('Ctrl Pts',(0.144442368330655,-0.0250068045060932,
-1.77794867036526));
#42818=CARTESIAN_POINT('Ctrl Pts',(0.136169499907116,-0.0727919066646952,
-1.78059776746791));
#42819=CARTESIAN_POINT('Ctrl Pts',(0.101832258591451,-0.11606457465997,
-1.78324686457056));
#42820=CARTESIAN_POINT('Ctrl Pts',(0.057177446920383,-0.1349802859837,-1.78589596167321));
#42821=CARTESIAN_POINT('Ctrl Pts',(0.0125226352493163,-0.153895997307429,
-1.78854505877586));
#42822=CARTESIAN_POINT('Ctrl Pts',(-0.0424497467771537,-0.148454751959616,
-1.79119415587851));
#42823=CARTESIAN_POINT('Ctrl Pts',(-0.0825297751355384,-0.121151864437375,
-1.79384325298116));
#42824=CARTESIAN_POINT('Ctrl Pts',(-0.121570651364079,-0.0945568569961039,
-1.79642366712601));
#42825=CARTESIAN_POINT('Ctrl Pts',(-0.146481389250798,-0.0472191224353378,
-1.79900408127086));
#42826=CARTESIAN_POINT('Ctrl Pts',(-0.146586453393407,2.34618399145015E-5,
-1.80158449541571));
#42827=CARTESIAN_POINT('Ctrl Pts',(-0.146572905486282,4.68275666195741E-5,
-1.80871550458428));
#42828=CARTESIAN_POINT('Ctrl Pts',(-0.146380875543874,-0.0459067401848022,
-1.80620611737716));
#42829=CARTESIAN_POINT('Ctrl Pts',(-0.123004041028004,-0.0920286568909353,
-1.80369673017004));
#42830=CARTESIAN_POINT('Ctrl Pts',(-0.0857438283361303,-0.118898837794897,
-1.80118734296292));
#42831=CARTESIAN_POINT('Ctrl Pts',(-0.0464091568250557,-0.147265013480497,
-1.79853824586027));
#42832=CARTESIAN_POINT('Ctrl Pts',(0.00839783863625381,-0.154176101711202,
-1.79588914875762));
#42833=CARTESIAN_POINT('Ctrl Pts',(0.053543079068469,-0.136462729016317,
-1.79324005165497));
#42834=CARTESIAN_POINT('Ctrl Pts',(0.0986883195006868,-0.118749356321431,
-1.79059095455232));
#42835=CARTESIAN_POINT('Ctrl Pts',(0.134171804903809,-0.0764115227009509,
-1.78794185744967));
#42836=CARTESIAN_POINT('Ctrl Pts',(0.143721073759422,-0.0288650425974362,
-1.78529276034702));
#42837=CARTESIAN_POINT('Ctrl Pts',(0.153270342615035,0.0186814375060771,
-1.78264366324437));
#42838=CARTESIAN_POINT('Ctrl Pts',(0.13688539492314,0.0714365640926248,
-1.77999456614172));
#42839=CARTESIAN_POINT('Ctrl Pts',(0.102080245380109,0.105207229931454,
-1.77734546903907));
#42840=CARTESIAN_POINT('Ctrl Pts',(0.0672750958370787,0.138977895770283,
-1.77469637193642));
#42841=CARTESIAN_POINT('Ctrl Pts',(0.0140497444429127,0.153764100861393,
-1.77204727483377));
#42842=CARTESIAN_POINT('Ctrl Pts',(-0.0331870599851328,0.142785001930372,
-1.76939817773112));
#42843=CARTESIAN_POINT('Ctrl Pts',(-0.0804238644131796,0.131805902999351,
-1.76674908062846));
#42844=CARTESIAN_POINT('Ctrl Pts',(-0.121672121875106,0.0950615000461977,
-1.76409998352581));
#42845=CARTESIAN_POINT('Ctrl Pts',(-0.138015689420879,0.0494025019649056,
-1.76145088642316));
#42846=CARTESIAN_POINT('Ctrl Pts',(-0.143640989427498,0.0336871104820155,
-1.76053909247687));
#42847=CARTESIAN_POINT('Ctrl Pts',(-0.146315903748105,0.0169156330188866,
-1.75962729853058));
#42848=CARTESIAN_POINT('Ctrl Pts',(-0.146200518682322,0.000108553130818545,
-1.75871550458428));
#42849=CARTESIAN_POINT('Origin',(0.,0.,-1.487));
#42850=CARTESIAN_POINT('',(-0.146154722497813,-8.18537555021537E-5,-1.70158449541571));
#42851=CARTESIAN_POINT('',(-0.146179203325735,-9.80254664548016E-5,-1.70871550458428));
#42852=CARTESIAN_POINT('',(-0.14635,-1.79227059055215E-17,-1.487));
#42853=CARTESIAN_POINT('Ctrl Pts',(-0.146154722497813,-8.18537555021537E-5,
-1.70158449541571));
#42854=CARTESIAN_POINT('Ctrl Pts',(-0.146003790237749,0.029671180203538,
-1.70319734647504));
#42855=CARTESIAN_POINT('Ctrl Pts',(-0.137184906065914,0.0595064104567512,
-1.70481019753436));
#42856=CARTESIAN_POINT('Ctrl Pts',(-0.120318227416389,0.0837404453770858,
-1.70642304859369));
#42857=CARTESIAN_POINT('Ctrl Pts',(-0.092614820283167,0.123544686023934,
-1.70907214569634));
#42858=CARTESIAN_POINT('Ctrl Pts',(-0.0432001993188249,0.14823810967376,
-1.71172124279899));
#42859=CARTESIAN_POINT('Ctrl Pts',(0.00526445918704815,0.146496496579415,
-1.71437033990164));
#42860=CARTESIAN_POINT('Ctrl Pts',(0.0537291176929198,0.14475488348507,
-1.71701943700429));
#42861=CARTESIAN_POINT('Ctrl Pts',(0.101243813740321,0.116578233646556,
-1.71966853410694));
#42862=CARTESIAN_POINT('Ctrl Pts',(0.126018662423459,0.0748881483385505,
-1.72231763120959));
#42863=CARTESIAN_POINT('Ctrl Pts',(0.150793511106598,0.0331980630305453,
-1.72496672831224));
#42864=CARTESIAN_POINT('Ctrl Pts',(0.152828512425473,-0.0220054577469498,
-1.7276158254149));
#42865=CARTESIAN_POINT('Ctrl Pts',(0.131190429966719,-0.0654064914647002,
-1.73026492251755));
#42866=CARTESIAN_POINT('Ctrl Pts',(0.109552347507966,-0.108807525182449,
-1.7329140196202));
#42867=CARTESIAN_POINT('Ctrl Pts',(0.0642411812715823,-0.140406071840456,
-1.73556311672285));
#42868=CARTESIAN_POINT('Ctrl Pts',(0.0160362938415837,-0.145711273827391,
-1.7382122138255));
#42869=CARTESIAN_POINT('Ctrl Pts',(-0.0321685935884163,-0.151016475814326,
-1.74086131092815));
#42870=CARTESIAN_POINT('Ctrl Pts',(-0.083267202212033,-0.130028333130192,
-1.7435104080308));
#42871=CARTESIAN_POINT('Ctrl Pts',(-0.113826091570257,-0.0923718513315293,
-1.74615950513345));
#42872=CARTESIAN_POINT('Ctrl Pts',(-0.134686240189591,-0.0666667349710097,
-1.74796783522754));
#42873=CARTESIAN_POINT('Ctrl Pts',(-0.145975458193573,-0.0331946420964979,
-1.74977616532162));
#42874=CARTESIAN_POINT('Ctrl Pts',(-0.146232247576531,0.000120056641797081,
-1.75158449541571));
#42875=CARTESIAN_POINT('Ctrl Pts',(-0.146200518682322,0.000108553130818545,
-1.75871550458428));
#42876=CARTESIAN_POINT('Ctrl Pts',(-0.145980667651508,-0.0319151217985716,
-1.75697820142793));
#42877=CARTESIAN_POINT('Ctrl Pts',(-0.135630836057442,-0.0640680487624917,
-1.75524089827157));
#42878=CARTESIAN_POINT('Ctrl Pts',(-0.116258389119244,-0.0892912352143908,
-1.75350359511521));
#42879=CARTESIAN_POINT('Ctrl Pts',(-0.0867186436422094,-0.127752381102974,
-1.75085449801256));
#42880=CARTESIAN_POINT('Ctrl Pts',(-0.0362002750585158,-0.150101079670706,
-1.74820540090991));
#42881=CARTESIAN_POINT('Ctrl Pts',(0.0121293699235867,-0.146088384589501,
-1.74555630380726));
#42882=CARTESIAN_POINT('Ctrl Pts',(0.0604590149056865,-0.142075689508295,
-1.74290720670461));
#42883=CARTESIAN_POINT('Ctrl Pts',(0.106599936286197,-0.111701600778155,
-1.74025810960196));
#42884=CARTESIAN_POINT('Ctrl Pts',(0.129392251966206,-0.068895448745377,
-1.73760901249931));
#42885=CARTESIAN_POINT('Ctrl Pts',(0.152184567646216,-0.0260892967125986,
-1.73495991539666));
#42886=CARTESIAN_POINT('Ctrl Pts',(0.151628277625726,0.0291489186228149,
-1.73231081829401));
#42887=CARTESIAN_POINT('Ctrl Pts',(0.127978492355377,0.0714873640663704,
-1.72966172119136));
#42888=CARTESIAN_POINT('Ctrl Pts',(0.104328707085028,0.113825809509926,
-1.72701262408871));
#42889=CARTESIAN_POINT('Ctrl Pts',(0.0575854265648198,0.143264485061621,
-1.72436352698606));
#42890=CARTESIAN_POINT('Ctrl Pts',(0.00918477029846232,0.146303033875848,
-1.72171442988341));
#42891=CARTESIAN_POINT('Ctrl Pts',(-0.0392158859678952,0.149341582690075,
-1.71906533278076));
#42892=CARTESIAN_POINT('Ctrl Pts',(-0.089273917980403,0.125980004766836,
-1.7164162356781));
#42893=CARTESIAN_POINT('Ctrl Pts',(-0.118033085945904,0.086931745345414,
-1.71376713857545));
#42894=CARTESIAN_POINT('Ctrl Pts',(-0.136313627683054,0.062111022542423,
-1.7120832605784));
#42895=CARTESIAN_POINT('Ctrl Pts',(-0.145988554068708,0.030952236506723,
-1.71039938258134));
#42896=CARTESIAN_POINT('Ctrl Pts',(-0.146179203325735,-9.80254664548015E-5,
-1.70871550458428));
#42897=CARTESIAN_POINT('Origin',(0.,0.,-1.487));
#42898=CARTESIAN_POINT('',(-0.14653173368382,-8.32536397529643E-5,-1.65158449541571));
#42899=CARTESIAN_POINT('',(-0.146557652869009,-6.33180884534729E-5,-1.65871550458428));
#42900=CARTESIAN_POINT('',(-0.14635,-1.79227059055215E-17,-1.487));
#42901=CARTESIAN_POINT('Ctrl Pts',(-0.14653173368382,-8.32536397529643E-5,
-1.65158449541571));
#42902=CARTESIAN_POINT('Ctrl Pts',(-0.146234877222684,0.0436237564073687,
-1.6539694305258));
#42903=CARTESIAN_POINT('Ctrl Pts',(-0.125401469120029,0.0875762997777429,
-1.65635436563589));
#42904=CARTESIAN_POINT('Ctrl Pts',(-0.0912258453865786,0.114746604194105,
-1.65873930074598));
#42905=CARTESIAN_POINT('Ctrl Pts',(-0.0532648352817327,0.144926366487419,
-1.66138839784863));
#42906=CARTESIAN_POINT('Ctrl Pts',(0.00115771916799673,0.154400304621344,
-1.66403749495128));
#42907=CARTESIAN_POINT('Ctrl Pts',(0.0470840407613024,0.138823741291476,
-1.66668659205393));
#42908=CARTESIAN_POINT('Ctrl Pts',(0.0930103623546093,0.123247177961607,
-1.66933568915658));
#42909=CARTESIAN_POINT('Ctrl Pts',(0.130440451091492,0.0826201131679442,
-1.67198478625923));
#42910=CARTESIAN_POINT('Ctrl Pts',(0.142209147696246,0.0355738155401125,
-1.67463388336189));
#42911=CARTESIAN_POINT('Ctrl Pts',(0.153977844300999,-0.0114724820877164,
-1.67728298046454));
#42912=CARTESIAN_POINT('Ctrl Pts',(0.140085148773626,-0.0649380125497132,
-1.67993207756719));
#42913=CARTESIAN_POINT('Ctrl Pts',(0.106902147572739,-0.100303882701074,
-1.68258117466984));
#42914=CARTESIAN_POINT('Ctrl Pts',(0.0737191463718505,-0.135669752852438,
-1.68523027177249));
#42915=CARTESIAN_POINT('Ctrl Pts',(0.0212458394974457,-0.152935962693163,
-1.68787936887514));
#42916=CARTESIAN_POINT('Ctrl Pts',(-0.0264539062358995,-0.144184357284127,
-1.69052846597779));
#42917=CARTESIAN_POINT('Ctrl Pts',(-0.0741536519692447,-0.135432751875091,
-1.69317756308044));
#42918=CARTESIAN_POINT('Ctrl Pts',(-0.11707983656153,-0.100663331216293,
-1.69582666018309));
#42919=CARTESIAN_POINT('Ctrl Pts',(-0.135546832206621,-0.055821092064959,
-1.69847575728574));
#42920=CARTESIAN_POINT('Ctrl Pts',(-0.142770558037638,-0.0382801748793176,
-1.69951200332906));
#42921=CARTESIAN_POINT('Ctrl Pts',(-0.146251695467758,-0.0191979795369924,
-1.70054824937239));
#42922=CARTESIAN_POINT('Ctrl Pts',(-0.146154722497813,-8.18537555021537E-5,
-1.70158449541571));
#42923=CARTESIAN_POINT('Ctrl Pts',(-0.146179203325735,-9.80254664548015E-5,
-1.70871550458428));
#42924=CARTESIAN_POINT('Ctrl Pts',(-0.146288485771181,-0.0178964088069292,
-1.70775028547869));
#42925=CARTESIAN_POINT('Ctrl Pts',(-0.143281500139797,-0.0356591341771629,
-1.7067850663731));
#42926=CARTESIAN_POINT('Ctrl Pts',(-0.136992758016216,-0.052172042109003,
-1.7058198472675));
#42927=CARTESIAN_POINT('Ctrl Pts',(-0.119732958202532,-0.0974926292223889,
-1.70317075016485));
#42928=CARTESIAN_POINT('Ctrl Pts',(-0.0777530546566726,-0.133398862529558,
-1.7005216530622));
#42929=CARTESIAN_POINT('Ctrl Pts',(-0.0303047177609532,-0.143424411479155,
-1.69787255595955));
#42930=CARTESIAN_POINT('Ctrl Pts',(0.0171436191347676,-0.153449960428753,
-1.6952234588569));
#42931=CARTESIAN_POINT('Ctrl Pts',(0.0700603893803513,-0.137594825020773,
-1.69257436175425));
#42932=CARTESIAN_POINT('Ctrl Pts',(0.104178357169689,-0.103130051993285,
-1.6899252646516));
#42933=CARTESIAN_POINT('Ctrl Pts',(0.138296324959027,-0.0686652789657974,
-1.68727616754895));
#42934=CARTESIAN_POINT('Ctrl Pts',(0.153615490292124,-0.0155908683188006,
-1.6846270704463));
#42935=CARTESIAN_POINT('Ctrl Pts',(0.143110598306188,0.0317536514303153,
-1.68197797334365));
#42936=CARTESIAN_POINT('Ctrl Pts',(0.132605706320252,0.079098171179434,
-1.679328876241));
#42937=CARTESIAN_POINT('Ctrl Pts',(0.0962767570152818,0.120712800030669,
-1.67667977913835));
#42938=CARTESIAN_POINT('Ctrl Pts',(0.0507839353436132,0.137513379849849,
-1.67403068203569));
#42939=CARTESIAN_POINT('Ctrl Pts',(0.00529111367194721,0.154313959669027,
-1.67138158493304));
#42940=CARTESIAN_POINT('Ctrl Pts',(-0.0493655803664143,0.146300490456153,
-1.6687324878304));
#42941=CARTESIAN_POINT('Ctrl Pts',(-0.0881209949026922,0.117147889370969,
-1.66608339072774));
#42942=CARTESIAN_POINT('Ctrl Pts',(-0.124050907457956,0.0901206876165238,
-1.66362742867992));
#42943=CARTESIAN_POINT('Ctrl Pts',(-0.146313617841786,0.0449243323049988,
-1.6611714666321));
#42944=CARTESIAN_POINT('Ctrl Pts',(-0.146557652869009,-6.33180884534729E-5,
-1.65871550458428));
#42945=CARTESIAN_POINT('Origin',(0.,0.,-1.487));
#42946=CARTESIAN_POINT('',(-0.146410789716796,0.000128174727319227,-1.60158449541571));
#42947=CARTESIAN_POINT('',(-0.14637109517831,0.000133274683421165,-1.60871550458428));
#42948=CARTESIAN_POINT('',(-0.14635,-1.79227059055215E-17,-1.487));
#42949=CARTESIAN_POINT('Ctrl Pts',(-0.146410789716796,0.000128174727319227,
-1.60158449541571));
#42950=CARTESIAN_POINT('Ctrl Pts',(-0.146496395207264,0.00945652267731366,
-1.60209241747391));
#42951=CARTESIAN_POINT('Ctrl Pts',(-0.145681450775993,0.0187699689983965,
-1.60260033953212));
#42952=CARTESIAN_POINT('Ctrl Pts',(-0.143911848766203,0.0278983480741794,
-1.60310826159032));
#42953=CARTESIAN_POINT('Ctrl Pts',(-0.134682386329468,0.0755079412607435,
-1.60575735869297));
#42954=CARTESIAN_POINT('Ctrl Pts',(-0.0994842823287073,0.118083326301294,
-1.60840645579562));
#42955=CARTESIAN_POINT('Ctrl Pts',(-0.0544591245016121,0.13609974944537,
-1.61105555289827));
#42956=CARTESIAN_POINT('Ctrl Pts',(-0.00943396667451821,0.154116172589446,
-1.61370465000092));
#42957=CARTESIAN_POINT('Ctrl Pts',(0.0454182449789114,0.147573633837048,
-1.61635374710357));
#42958=CARTESIAN_POINT('Ctrl Pts',(0.0849426956711816,0.119472492619379,
-1.61900284420622));
#42959=CARTESIAN_POINT('Ctrl Pts',(0.124467146363453,0.0913713514017089,
-1.62165194130887));
#42960=CARTESIAN_POINT('Ctrl Pts',(0.148663836094565,0.0417116077187646,
-1.62430103841153));
#42961=CARTESIAN_POINT('Ctrl Pts',(0.146436343584327,-0.00673315069097555,
-1.62695013551418));
#42962=CARTESIAN_POINT('Ctrl Pts',(0.14420885107409,-0.0551779091007144,
-1.62959923261683));
#42963=CARTESIAN_POINT('Ctrl Pts',(0.115557176322507,-0.102407682237246,
-1.63224832971948));
#42964=CARTESIAN_POINT('Ctrl Pts',(0.0736207634832826,-0.126763248714733,
-1.63489742682213));
#42965=CARTESIAN_POINT('Ctrl Pts',(0.0316843506440586,-0.151118815192219,
-1.63754652392478));
#42966=CARTESIAN_POINT('Ctrl Pts',(-0.0235368002828062,-0.152600175010656,
-1.64019562102743));
#42967=CARTESIAN_POINT('Ctrl Pts',(-0.0667186817131846,-0.130527987615796,
-1.64284471813008));
#42968=CARTESIAN_POINT('Ctrl Pts',(-0.109900563143564,-0.108455800220934,
-1.64549381523273));
#42969=CARTESIAN_POINT('Ctrl Pts',(-0.141043175077458,-0.0628300656127732,
-1.64814291233538));
#42970=CARTESIAN_POINT('Ctrl Pts',(-0.145864748164422,-0.0145744050823413,
-1.65079200943803));
#42971=CARTESIAN_POINT('Ctrl Pts',(-0.146345544565827,-0.00976245937251802,
-1.65105617143059));
#42972=CARTESIAN_POINT('Ctrl Pts',(-0.146564614324448,-0.0049243626552666,
-1.65132033342315));
#42973=CARTESIAN_POINT('Ctrl Pts',(-0.14653173368382,-8.32536397529643E-5,
-1.65158449541571));
#42974=CARTESIAN_POINT('Ctrl Pts',(-0.146557652869009,-6.33180884534729E-5,
-1.65871550458428));
#42975=CARTESIAN_POINT('Ctrl Pts',(-0.146576843604633,-0.00360111393230097,
-1.65852236952945));
#42976=CARTESIAN_POINT('Ctrl Pts',(-0.14645986789498,-0.00713761911690831,
-1.65832923447462));
#42977=CARTESIAN_POINT('Ctrl Pts',(-0.146202664286797,-0.0106638961995758,
-1.65813609941979));
#42978=CARTESIAN_POINT('Ctrl Pts',(-0.142674784100431,-0.0590313477274492,
-1.65548700231714));
#42979=CARTESIAN_POINT('Ctrl Pts',(-0.112764888693505,-0.105474517825706,
-1.65283790521449));
#42980=CARTESIAN_POINT('Ctrl Pts',(-0.0701894328195342,-0.12869491538979,
-1.65018880811184));
#42981=CARTESIAN_POINT('Ctrl Pts',(-0.0276139769455624,-0.151915312953875,
-1.64753971100919));
#42982=CARTESIAN_POINT('Ctrl Pts',(0.0276270393954554,-0.151912937983787,
-1.64489061390654));
#42983=CARTESIAN_POINT('Ctrl Pts',(0.0702004984887575,-0.128688879623078,
-1.64224151680389));
#42984=CARTESIAN_POINT('Ctrl Pts',(0.112773957582058,-0.10546482126237,
-1.63959241970124));
#42985=CARTESIAN_POINT('Ctrl Pts',(0.142679859427646,-0.0590190795110429,
-1.63694332259859));
#42986=CARTESIAN_POINT('Ctrl Pts',(0.146203580689421,-0.0106513248145528,
-1.63429422549594));
#42987=CARTESIAN_POINT('Ctrl Pts',(0.149727301951196,0.0377164298819386,
-1.63164512839329));
#42988=CARTESIAN_POINT('Ctrl Pts',(0.126868842629159,0.0880061975235912,
-1.62899603129064));
#42989=CARTESIAN_POINT('Ctrl Pts',(0.0881109215279091,0.117155466087655,
-1.62634693418799));
#42990=CARTESIAN_POINT('Ctrl Pts',(0.0493530004266599,0.146304734651718,
-1.62369783708534));
#42991=CARTESIAN_POINT('Ctrl Pts',(-0.00530438245380212,0.154313504138191,
-1.62104873998269));
#42992=CARTESIAN_POINT('Ctrl Pts',(-0.0507957593468502,0.137509012646772,
-1.61839964288004));
#42993=CARTESIAN_POINT('Ctrl Pts',(-0.0962871362398984,0.120704521155352,
-1.61575054577738));
#42994=CARTESIAN_POINT('Ctrl Pts',(-0.132612507145534,0.079086768686041,
-1.61310144867473));
#42995=CARTESIAN_POINT('Ctrl Pts',(-0.143113328138643,0.0317413458409419,
-1.61045235157208));
#42996=CARTESIAN_POINT('Ctrl Pts',(-0.145408238266455,0.0213942034161637,
-1.60987340257615));
#42997=CARTESIAN_POINT('Ctrl Pts',(-0.146469709565528,0.0107734945182561,
-1.60929445358022));
#42998=CARTESIAN_POINT('Ctrl Pts',(-0.14637109517831,0.000133274683421165,
-1.60871550458428));
#42999=CARTESIAN_POINT('Origin',(0.,0.,-1.487));
#43000=CARTESIAN_POINT('',(-0.146109700211217,1.35404246933285E-5,-1.55158449541571));
#43001=CARTESIAN_POINT('',(-0.146108968460049,-8.05953396676445E-6,-1.55871550458429));
#43002=CARTESIAN_POINT('',(-0.14635,-1.79227059055215E-17,-1.487));
#43003=CARTESIAN_POINT('Ctrl Pts',(-0.146109700211217,1.35404246933285E-5,
-1.55158449541571));
#43004=CARTESIAN_POINT('Ctrl Pts',(-0.146129167206823,0.023644608817299,
-1.55286450152468));
#43005=CARTESIAN_POINT('Ctrl Pts',(-0.14072606949062,0.0472672806948128,
-1.55414450763364));
#43006=CARTESIAN_POINT('Ctrl Pts',(-0.129852420916273,0.0680241635211907,
-1.55542451374261));
#43007=CARTESIAN_POINT('Ctrl Pts',(-0.107348347903067,0.110982550805601,
-1.55807361084526));
#43008=CARTESIAN_POINT('Ctrl Pts',(-0.0614126325066573,0.141666096683144,
-1.56072270794791));
#43009=CARTESIAN_POINT('Ctrl Pts',(-0.0131110508935279,0.14600355606985,
-1.56337180505056));
#43010=CARTESIAN_POINT('Ctrl Pts',(0.0351905307196015,0.150341015456556,
-1.56602090215321));
#43011=CARTESIAN_POINT('Ctrl Pts',(0.085857978549451,0.128332388352425,
-1.56866999925586));
#43012=CARTESIAN_POINT('Ctrl Pts',(0.115655579258376,0.0900706668510009,
-1.57131909635851));
#43013=CARTESIAN_POINT('Ctrl Pts',(0.145453179967302,0.0518089453495764,
-1.57396819346116));
#43014=CARTESIAN_POINT('Ctrl Pts',(0.154380933555303,-0.0027058705491417,
-1.57661729056382));
#43015=CARTESIAN_POINT('Ctrl Pts',(0.138344638873419,-0.0484736932320802,
-1.57926638766647));
#43016=CARTESIAN_POINT('Ctrl Pts',(0.122308344191535,-0.0942415159150187,
-1.58191548476912));
#43017=CARTESIAN_POINT('Ctrl Pts',(0.081308001239765,-0.131262345382178,
-1.58456458187177));
#43018=CARTESIAN_POINT('Ctrl Pts',(0.034146061224487,-0.14255870560379,
-1.58721367897442));
#43019=CARTESIAN_POINT('Ctrl Pts',(-0.0130158787907924,-0.153855065825403,
-1.58986277607707));
#43020=CARTESIAN_POINT('Ctrl Pts',(-0.0663394158695805,-0.139426956801469,
-1.59251187317972));
#43021=CARTESIAN_POINT('Ctrl Pts',(-0.101370773972617,-0.105891001623212,
-1.59516097028237));
#43022=CARTESIAN_POINT('Ctrl Pts',(-0.129685428678273,-0.0787850302160007,
-1.59730214532682));
#43023=CARTESIAN_POINT('Ctrl Pts',(-0.146049914781562,-0.0391960198294007,
-1.59944332037126));
#43024=CARTESIAN_POINT('Ctrl Pts',(-0.146410789716796,0.000128174727319227,
-1.60158449541571));
#43025=CARTESIAN_POINT('Ctrl Pts',(-0.14637109517831,0.000133274683421165,
-1.60871550458428));
#43026=CARTESIAN_POINT('Ctrl Pts',(-0.146018479682941,-0.0379129627241524,
-1.60664535647757));
#43027=CARTESIAN_POINT('Ctrl Pts',(-0.130833434658462,-0.0762086598056477,
-1.60457520837085));
#43028=CARTESIAN_POINT('Ctrl Pts',(-0.104169489069799,-0.103139009466109,
-1.60250506026413));
#43029=CARTESIAN_POINT('Ctrl Pts',(-0.0700485579272628,-0.137600848707174,
-1.59985596316148));
#43030=CARTESIAN_POINT('Ctrl Pts',(-0.017130424561609,-0.153451433968415,
-1.59720686605883));
#43031=CARTESIAN_POINT('Ctrl Pts',(0.0303170501043716,-0.143421805175092,
-1.59455776895618));
#43032=CARTESIAN_POINT('Ctrl Pts',(0.0777645247703496,-0.13339217638177,
-1.59190867185353));
#43033=CARTESIAN_POINT('Ctrl Pts',(0.119741340736654,-0.0974823335338879,
-1.58925957475088));
#43034=CARTESIAN_POINT('Ctrl Pts',(0.136997243561903,-0.052160262491227,
-1.58661047764823));
#43035=CARTESIAN_POINT('Ctrl Pts',(0.154253146387154,-0.00683819144856339,
-1.58396138054558));
#43036=CARTESIAN_POINT('Ctrl Pts',(0.146788136071344,0.0478961077888828,
-1.58131228344293));
#43037=CARTESIAN_POINT('Ctrl Pts',(0.118025610618323,0.0869418941873539,
-1.57866318634028));
#43038=CARTESIAN_POINT('Ctrl Pts',(0.0892630851653034,0.125987680585823,
-1.57601408923763));
#43039=CARTESIAN_POINT('Ctrl Pts',(0.0392030445750755,0.149344954145322,
-1.57336499213497));
#43040=CARTESIAN_POINT('Ctrl Pts',(-0.00919735024045918,0.146302243575645,
-1.57071589503232));
#43041=CARTESIAN_POINT('Ctrl Pts',(-0.0575977450559952,0.143259533005969,
-1.56806679792967));
#43042=CARTESIAN_POINT('Ctrl Pts',(-0.104338494096836,0.113816838307116,
-1.56541770082703));
#43043=CARTESIAN_POINT('Ctrl Pts',(-0.127984638776814,0.0714763594755748,
-1.56276860372438));
#43044=CARTESIAN_POINT('Ctrl Pts',(-0.14004411476116,0.0498828187717894,
-1.56141757067768));
#43045=CARTESIAN_POINT('Ctrl Pts',(-0.146096741734407,0.0249345965739106,
-1.56006653763098));
#43046=CARTESIAN_POINT('Ctrl Pts',(-0.146108968460049,-8.05953396676445E-6,
-1.55871550458429));
#43047=CARTESIAN_POINT('Origin',(0.,0.,-1.487));
#43048=CARTESIAN_POINT('',(-0.146360964522871,-0.000133965814129389,-1.50158449541571));
#43049=CARTESIAN_POINT('',(-0.146400754326123,-0.000129830579301018,-1.50871550458428));
#43050=CARTESIAN_POINT('',(-0.14635,-1.79227059055215E-17,-1.487));
#43051=CARTESIAN_POINT('Ctrl Pts',(-0.146360964522871,-0.000133965814129389,
-1.50158449541571));
#43052=CARTESIAN_POINT('Ctrl Pts',(-0.146011950827357,0.0375870817956262,
-1.50363658557544));
#43053=CARTESIAN_POINT('Ctrl Pts',(-0.131118218928743,0.0755527203925127,
-1.50568867573517));
#43054=CARTESIAN_POINT('Ctrl Pts',(-0.104869208528632,0.102427472599654,
-1.5077407658949));
#43055=CARTESIAN_POINT('Ctrl Pts',(-0.0709836713514958,0.137120796315871,
-1.51038986299755));
#43056=CARTESIAN_POINT('Ctrl Pts',(-0.0181746687979467,0.153331261636109,
-1.5130389601002));
#43057=CARTESIAN_POINT('Ctrl Pts',(0.0293399847849844,0.143624870177109,
-1.51568805720285));
#43058=CARTESIAN_POINT('Ctrl Pts',(0.0768546383679142,0.13391847871811,
-1.5183371543055));
#43059=CARTESIAN_POINT('Ctrl Pts',(0.119074942980225,0.0982952304798761,
-1.52098625140815));
#43060=CARTESIAN_POINT('Ctrl Pts',(0.136638982105141,0.0530916811736593,
-1.52363534851081));
#43061=CARTESIAN_POINT('Ctrl Pts',(0.154203021230057,0.00788813186744377,
-1.52628444561345));
#43062=CARTESIAN_POINT('Ctrl Pts',(0.147110794867578,-0.0468957185067564,
-1.5289335427161));
#43063=CARTESIAN_POINT('Ctrl Pts',(0.118614745083421,-0.0861364051337745,
-1.53158263981876));
#43064=CARTESIAN_POINT('Ctrl Pts',(0.0901186952992629,-0.125377091760793,
-1.53423173692141));
#43065=CARTESIAN_POINT('Ctrl Pts',(0.0402188220934277,-0.149074614640631,
-1.53688083402406));
#43066=CARTESIAN_POINT('Ctrl Pts',(-0.00820116518900179,-0.146361466684771,
-1.53952993112671));
#43067=CARTESIAN_POINT('Ctrl Pts',(-0.056621152471434,-0.14364831872891,
-1.54217902822936));
#43068=CARTESIAN_POINT('Ctrl Pts',(-0.103561253830459,-0.114524499937346,
-1.54482812533201));
#43069=CARTESIAN_POINT('Ctrl Pts',(-0.12749508919497,-0.0723459761959237,
-1.54747722243466));
#43070=CARTESIAN_POINT('Ctrl Pts',(-0.139864435116293,-0.0505475162891599,
-1.54884631342834));
#43071=CARTESIAN_POINT('Ctrl Pts',(-0.146088878366562,-0.0252621849650469,
-1.55021540442203));
#43072=CARTESIAN_POINT('Ctrl Pts',(-0.146109700211217,1.35404246933285E-5,
-1.55158449541571));
#43073=CARTESIAN_POINT('Ctrl Pts',(-0.146108968460049,-8.05953396676445E-6,
-1.55871550458429));
#43074=CARTESIAN_POINT('Ctrl Pts',(-0.146120715821164,-0.0239728066826975,
-1.55741744052833));
#43075=CARTESIAN_POINT('Ctrl Pts',(-0.140556421379631,-0.0479324156370611,
-1.55611937647238));
#43076=CARTESIAN_POINT('Ctrl Pts',(-0.129386327461104,-0.0689065743803954,
-1.55482131241642));
#43077=CARTESIAN_POINT('Ctrl Pts',(-0.106590331146305,-0.111710766440592,
-1.55217221531377));
#43078=CARTESIAN_POINT('Ctrl Pts',(-0.0604467981975962,-0.142080887596758,
-1.54952311821112));
#43079=CARTESIAN_POINT('Ctrl Pts',(-0.0121168083595676,-0.146089427002404,
-1.54687402110847));
#43080=CARTESIAN_POINT('Ctrl Pts',(0.0362131814784611,-0.150097966408049,
-1.54422492400582));
#43081=CARTESIAN_POINT('Ctrl Pts',(0.0867296282058091,-0.127744924063173,
-1.54157582690317));
#43082=CARTESIAN_POINT('Ctrl Pts',(0.116266066463203,-0.0892812383196336,
-1.53892672980052));
#43083=CARTESIAN_POINT('Ctrl Pts',(0.145802504720596,-0.0508175525760944,
-1.53627763269787));
#43084=CARTESIAN_POINT('Ctrl Pts',(0.154358934508036,0.00375677656610807,
-1.53362853559522));
#43085=CARTESIAN_POINT('Ctrl Pts',(0.13801144099953,0.0494143691647103,
-1.53097943849257));
#43086=CARTESIAN_POINT('Ctrl Pts',(0.121663947491025,0.0950719617633139,
-1.52833034138992));
#43087=CARTESIAN_POINT('Ctrl Pts',(0.080412530686573,0.131812817818317,
-1.52568124428727));
#43088=CARTESIAN_POINT('Ctrl Pts',(0.0331747823871046,0.142787855016739,
-1.52303214718461));
#43089=CARTESIAN_POINT('Ctrl Pts',(-0.0140629659123612,0.153762892215161,
-1.52038305008196));
#43090=CARTESIAN_POINT('Ctrl Pts',(-0.0672870457068432,0.138972110557006,
-1.51773395297932));
#43091=CARTESIAN_POINT('Ctrl Pts',(-0.102089291325209,0.105198452096168,
-1.51508485587667));
#43092=CARTESIAN_POINT('Ctrl Pts',(-0.129981527751131,0.0781305761582737,
-1.51296173877921));
#43093=CARTESIAN_POINT('Ctrl Pts',(-0.146041032707425,0.0388695992739819,
-1.51083862168174));
#43094=CARTESIAN_POINT('Ctrl Pts',(-0.146400754326123,-0.000129830579301018,
-1.50871550458428));
#43095=CARTESIAN_POINT('Origin',(0.,0.,-1.487));
#43096=CARTESIAN_POINT('',(-0.146563252594768,5.78712481600838E-5,-1.45158449541571));
#43097=CARTESIAN_POINT('',(-0.146538870035492,7.8428438803138E-5,-1.45871550458428));
#43098=CARTESIAN_POINT('',(-0.14635,-1.79227059055215E-17,-1.487));
#43099=CARTESIAN_POINT('Ctrl Pts',(-0.146563252594768,5.78712481600838E-5,
-1.45158449541571));
#43100=CARTESIAN_POINT('Ctrl Pts',(-0.146579365056784,0.00326456151995294,
-1.45175957252355));
#43101=CARTESIAN_POINT('Ctrl Pts',(-0.146483262220459,0.00647026841391055,
-1.4519346496314));
#43102=CARTESIAN_POINT('Ctrl Pts',(-0.146271873409478,0.00966835507499523,
-1.45210972673924));
#43103=CARTESIAN_POINT('Ctrl Pts',(-0.143073342810017,0.0580587026896339,
-1.45475882384189));
#43104=CARTESIAN_POINT('Ctrl Pts',(-0.113480308324777,0.104704412530463,
-1.45740792094454));
#43105=CARTESIAN_POINT('Ctrl Pts',(-0.0710639146539858,0.128214110278961,
-1.46005701804719));
#43106=CARTESIAN_POINT('Ctrl Pts',(-0.0286475209831971,0.151723808027457,
-1.46270611514984));
#43107=CARTESIAN_POINT('Ctrl Pts',(0.0265922318731414,0.152097493683626,
-1.46535521225249));
#43108=CARTESIAN_POINT('Ctrl Pts',(0.0693228056249136,0.129163797795145,
-1.46800430935514));
#43109=CARTESIAN_POINT('Ctrl Pts',(0.112053379376688,0.106230101906662,
-1.47065340645779));
#43110=CARTESIAN_POINT('Ctrl Pts',(0.142274774023895,0.0599890244735269,
-1.47330250356044));
#43111=CARTESIAN_POINT('Ctrl Pts',(0.146127683586795,0.0116463784127105,
-1.4759516006631));
#43112=CARTESIAN_POINT('Ctrl Pts',(0.149980593149695,-0.0366962676481046,
-1.47860069776575));
#43113=CARTESIAN_POINT('Ctrl Pts',(0.12746501762829,-0.0871404823366008,
-1.4812497948684));
#43114=CARTESIAN_POINT('Ctrl Pts',(0.0889064318758686,-0.116552925367303,
-1.48389889197105));
#43115=CARTESIAN_POINT('Ctrl Pts',(0.0503478461234483,-0.145965368398004,
-1.4865479890737));
#43116=CARTESIAN_POINT('Ctrl Pts',(-0.00425374985998689,-0.154346039770913,
-1.48919708617635));
#43117=CARTESIAN_POINT('Ctrl Pts',(-0.0498584717623352,-0.13785162615689,
-1.491846183279));
#43118=CARTESIAN_POINT('Ctrl Pts',(-0.0954631936646862,-0.121357212542867,
-1.49449528038165));
#43119=CARTESIAN_POINT('Ctrl Pts',(-0.132071041485949,-0.0799877139419083,
-1.4971443774843));
#43120=CARTESIAN_POINT('Ctrl Pts',(-0.142893929496219,-0.0327148735853313,
-1.49979347458695));
#43121=CARTESIAN_POINT('Ctrl Pts',(-0.145333001766583,-0.022061351720772,
-1.50039048152987));
#43122=CARTESIAN_POINT('Ctrl Pts',(-0.146462501776685,-0.0111080096252457,
-1.50098748847279));
#43123=CARTESIAN_POINT('Ctrl Pts',(-0.146360964522871,-0.000133965814129389,
-1.50158449541571));
#43124=CARTESIAN_POINT('Ctrl Pts',(-0.146400754326123,-0.000129830579301018,
-1.50871550458428));
#43125=CARTESIAN_POINT('Ctrl Pts',(-0.146489871586351,-0.00979153051154047,
-1.50818952457909));
#43126=CARTESIAN_POINT('Ctrl Pts',(-0.145615416708744,-0.0194371780291451,
-1.5076635445739));
#43127=CARTESIAN_POINT('Ctrl Pts',(-0.143718591245809,-0.0288774004549093,
-1.50713756456871));
#43128=CARTESIAN_POINT('Ctrl Pts',(-0.134165234105791,-0.0764230592816198,
-1.50448846746606));
#43129=CARTESIAN_POINT('Ctrl Pts',(-0.0986781083835066,-0.118757841671515,
-1.50183937036341));
#43130=CARTESIAN_POINT('Ctrl Pts',(-0.0535313450205615,-0.136467332453605,
-1.49919027326076));
#43131=CARTESIAN_POINT('Ctrl Pts',(-0.00838458165761895,-0.154176823235693,
-1.49654117615811));
#43132=CARTESIAN_POINT('Ctrl Pts',(0.0464218193459839,-0.147261022409979,
-1.49389207905546));
#43133=CARTESIAN_POINT('Ctrl Pts',(0.0857540516247829,-0.11889146460805,
-1.49124298195281));
#43134=CARTESIAN_POINT('Ctrl Pts',(0.125086283903585,-0.0905219068061183,
-1.48859388485016));
#43135=CARTESIAN_POINT('Ctrl Pts',(0.148944347457581,-0.0406985920279711,
-1.48594478774751));
#43136=CARTESIAN_POINT('Ctrl Pts',(0.146387112443533,0.00772987950473067,
-1.48329569064486));
#43137=CARTESIAN_POINT('Ctrl Pts',(0.143829877429484,0.0561583510374297,
-1.48064659354221));
#43138=CARTESIAN_POINT('Ctrl Pts',(0.114857343847392,0.103191979324682,
-1.47799749643956));
#43139=CARTESIAN_POINT('Ctrl Pts',(0.0727560993153952,0.127261493544282,
-1.47534839933691));
#43140=CARTESIAN_POINT('Ctrl Pts',(0.0306548547833984,0.151331007763883,
-1.47269930223425));
#43141=CARTESIAN_POINT('Ctrl Pts',(-0.0245751006985043,0.152436407915832,
-1.4700502051316));
#43142=CARTESIAN_POINT('Ctrl Pts',(-0.067605721842972,0.13007076574236,
-1.46740110802895));
#43143=CARTESIAN_POINT('Ctrl Pts',(-0.11063634298744,0.107705123568887,
-1.4647520109263));
#43144=CARTESIAN_POINT('Ctrl Pts',(-0.141467629794474,0.0618684390699918,
-1.46210291382365));
#43145=CARTESIAN_POINT('Ctrl Pts',(-0.14596058429274,0.0135810735818327,
-1.459453816721));
#43146=CARTESIAN_POINT('Ctrl Pts',(-0.146377984726076,0.00909512401630342,
-1.45920771267543));
#43147=CARTESIAN_POINT('Ctrl Pts',(-0.146568069149991,0.00458802356634012,
-1.45896160862986));
#43148=CARTESIAN_POINT('Ctrl Pts',(-0.146538870035492,7.8428438803138E-5,
-1.45871550458428));
#43149=CARTESIAN_POINT('Origin',(0.,0.,-1.487));
#43150=CARTESIAN_POINT('',(-0.146186144827487,0.00010175201331792,-1.40158449541571));
#43151=CARTESIAN_POINT('',(-0.14616050398721,8.61805021221069E-5,-1.40871550458428));
#43152=CARTESIAN_POINT('',(-0.14635,-1.79227059055215E-17,-1.487));
#43153=CARTESIAN_POINT('Ctrl Pts',(-0.146186144827487,0.00010175201331792,
-1.40158449541571));
#43154=CARTESIAN_POINT('Ctrl Pts',(-0.146297791485825,0.0175650700753052,
-1.40253165657432));
#43155=CARTESIAN_POINT('Ctrl Pts',(-0.143405387297582,0.0349926282668302,
-1.40347881773292));
#43156=CARTESIAN_POINT('Ctrl Pts',(-0.137344752713405,0.0512382371151499,
-1.40442597889153));
#43157=CARTESIAN_POINT('Ctrl Pts',(-0.12039387865013,0.0966752727661706,
-1.40707507599418));
#43158=CARTESIAN_POINT('Ctrl Pts',(-0.078659384026827,0.132866458089903,
-1.40972417309683));
#43159=CARTESIAN_POINT('Ctrl Pts',(-0.0312803965259292,0.143214785667386,
-1.41237327019948));
#43160=CARTESIAN_POINT('Ctrl Pts',(0.0160985909749686,0.153563113244869,
-1.41502236730213));
#43161=CARTESIAN_POINT('Ctrl Pts',(0.0691220713534613,0.138068583076103,
-1.41767146440478));
#43162=CARTESIAN_POINT('Ctrl Pts',(0.103473872333095,0.103836871028401,
-1.42032056150743));
#43163=CARTESIAN_POINT('Ctrl Pts',(0.137825673312729,0.0696051589807,-1.42296965861008));
#43164=CARTESIAN_POINT('Ctrl Pts',(0.153505794893504,0.0166362650540631,
-1.42561875571273));
#43165=CARTESIAN_POINT('Ctrl Pts',(0.143323450372017,-0.0307786714143838,
-1.42826785281539));
#43166=CARTESIAN_POINT('Ctrl Pts',(0.133141105850529,-0.078193607882832,
-1.43091694991804));
#43167=CARTESIAN_POINT('Ctrl Pts',(0.0970962952267766,-0.12005458689309,
-1.43356604702069));
#43168=CARTESIAN_POINT('Ctrl Pts',(0.0517188995750107,-0.137164475967083,
-1.43621514412334));
#43169=CARTESIAN_POINT('Ctrl Pts',(0.00634150392324483,-0.154274365041076,
-1.43886424122599));
#43170=CARTESIAN_POINT('Ctrl Pts',(-0.0483684767565346,-0.146633164178805,
-1.44151333832864));
#43171=CARTESIAN_POINT('Ctrl Pts',(-0.0873214537395813,-0.117745071053445,
-1.44416243543129));
#43172=CARTESIAN_POINT('Ctrl Pts',(-0.12370005376028,-0.0907661732499322,
-1.4466364554261));
#43173=CARTESIAN_POINT('Ctrl Pts',(-0.146335566898538,-0.0452559675928817,
-1.4491104754209));
#43174=CARTESIAN_POINT('Ctrl Pts',(-0.146563252594768,5.78712481600838E-5,
-1.45158449541571));
#43175=CARTESIAN_POINT('Ctrl Pts',(-0.146538870035492,7.8428438803138E-5,
-1.45871550458428));
#43176=CARTESIAN_POINT('Ctrl Pts',(-0.146253765947706,-0.0439538659368936,
-1.45631251152721));
#43177=CARTESIAN_POINT('Ctrl Pts',(-0.125062536189296,-0.0882239986986389,
-1.45390951847013));
#43178=CARTESIAN_POINT('Ctrl Pts',(-0.0904425780473909,-0.11536497650004,
-1.45150652541305));
#43179=CARTESIAN_POINT('Ctrl Pts',(-0.0522769951142755,-0.145285614616334,
-1.4488574283104));
#43180=CARTESIAN_POINT('Ctrl Pts',(0.00220879294145686,-0.154388844371495,
-1.44620833120775));
#43181=CARTESIAN_POINT('Ctrl Pts',(0.0480280104588239,-0.138499992556246,
-1.4435592341051));
#43182=CARTESIAN_POINT('Ctrl Pts',(0.0938472279761883,-0.122611140740998,
-1.44091013700245));
#43183=CARTESIAN_POINT('Ctrl Pts',(0.130999874955191,-0.081730207355346,
-1.4382610398998));
#43184=CARTESIAN_POINT('Ctrl Pts',(0.142448024839166,-0.0346048832700464,
-1.43561194279715));
#43185=CARTESIAN_POINT('Ctrl Pts',(0.153896174723141,0.0125204408152545,
-1.4329628456945));
#43186=CARTESIAN_POINT('Ctrl Pts',(0.139639827512083,0.0658901556002054,
-1.43031374859185));
#43187=CARTESIAN_POINT('Ctrl Pts',(0.106216837612053,0.101029308294217,
-1.4276646514892));
#43188=CARTESIAN_POINT('Ctrl Pts',(0.0727938477120221,0.136168460988228,
-1.42501555438655));
#43189=CARTESIAN_POINT('Ctrl Pts',(0.0202042151230188,0.153077051591303,
-1.4223664572839));
#43190=CARTESIAN_POINT('Ctrl Pts',(-0.0274348472360513,0.144000926677045,
-1.41971736018125));
#43191=CARTESIAN_POINT('Ctrl Pts',(-0.0750739095951214,0.134924801762786,
-1.41706826307859));
#43192=CARTESIAN_POINT('Ctrl Pts',(-0.117762401724257,0.0998639613311952,
-1.41441916597594));
#43193=CARTESIAN_POINT('Ctrl Pts',(-0.135923699806529,0.0548970450718224,
-1.41177006887329));
#43194=CARTESIAN_POINT('Ctrl Pts',(-0.142904046998363,0.0376138813786416,
-1.41075188077696));
#43195=CARTESIAN_POINT('Ctrl Pts',(-0.146261062082397,0.0188673214836565,
-1.40973369268062));
#43196=CARTESIAN_POINT('Ctrl Pts',(-0.14616050398721,8.61805021221068E-5,
-1.40871550458428));
#43197=CARTESIAN_POINT('Origin',(0.,0.,-1.487));
#43198=CARTESIAN_POINT('',(-0.146193053794332,-0.000105164914211059,-1.35158449541571));
#43199=CARTESIAN_POINT('',(-0.146223843614078,-0.00011741876304885,-1.35871550458429));
#43200=CARTESIAN_POINT('',(-0.14635,-1.79227059055215E-17,-1.487));
#43201=CARTESIAN_POINT('Ctrl Pts',(-0.146193053794332,-0.000105164914211059,
-1.35158449541571));
#43202=CARTESIAN_POINT('Ctrl Pts',(-0.145982970582079,0.0315897173710793,
-1.35330374062508));
#43203=CARTESIAN_POINT('Ctrl Pts',(-0.135864273539381,0.0634067802567858,
-1.35502298583445));
#43204=CARTESIAN_POINT('Ctrl Pts',(-0.11686355797358,0.0884977223341386,
-1.35674223104382));
#43205=CARTESIAN_POINT('Ctrl Pts',(-0.0875863261515443,0.127159073023167,
-1.35939132814647));
#43206=CARTESIAN_POINT('Ctrl Pts',(-0.0372212695608701,0.149851164403594,
-1.36204042524912));
#43207=CARTESIAN_POINT('Ctrl Pts',(0.0111345728257042,0.146167572766889,
-1.36468952235177));
#43208=CARTESIAN_POINT('Ctrl Pts',(0.0594904152122772,0.142483981130183,
-1.36733861945442));
#43209=CARTESIAN_POINT('Ctrl Pts',(0.105837043394752,0.112424706476348,
-1.36998771655707));
#43210=CARTESIAN_POINT('Ctrl Pts',(0.128920239670456,0.0697747077664019,
-1.37263681365972));
#43211=CARTESIAN_POINT('Ctrl Pts',(0.152003435946159,0.0271247090564568,
-1.37528591076238));
#43212=CARTESIAN_POINT('Ctrl Pts',(0.151823200315095,-0.0281160137095958,
-1.37793500786503));
#43213=CARTESIAN_POINT('Ctrl Pts',(0.128462187492193,-0.0706144774482909,
-1.38058410496768));
#43214=CARTESIAN_POINT('Ctrl Pts',(0.10510117466929,-0.113112941186989,
-1.38323320207033));
#43215=CARTESIAN_POINT('Ctrl Pts',(0.0585593846545423,-0.142869145898326,
-1.38588229917298));
#43216=CARTESIAN_POINT('Ctrl Pts',(0.0101805349100076,-0.146237118234464,
-1.38853139627563));
#43217=CARTESIAN_POINT('Ctrl Pts',(-0.0381983148345271,-0.149605090570603,
-1.39118049337828));
#43218=CARTESIAN_POINT('Ctrl Pts',(-0.0884142243088482,-0.126584830531547,
-1.39382959048093));
#43219=CARTESIAN_POINT('Ctrl Pts',(-0.117438552294387,-0.0877332575228631,
-1.39647868758358));
#43220=CARTESIAN_POINT('Ctrl Pts',(-0.136085489396421,-0.06277271963999,
-1.39818062352762));
#43221=CARTESIAN_POINT('Ctrl Pts',(-0.145985529062017,-0.0312777534086356,
-1.39988255947167));
#43222=CARTESIAN_POINT('Ctrl Pts',(-0.146186144827487,0.00010175201331792,
-1.40158449541571));
#43223=CARTESIAN_POINT('Ctrl Pts',(-0.14616050398721,8.61805021221068E-5,
-1.40871550458428));
#43224=CARTESIAN_POINT('Ctrl Pts',(-0.145999432468413,-0.029996995765469,
-1.40708459557797));
#43225=CARTESIAN_POINT('Ctrl Pts',(-0.136967315343511,-0.0601688962277433,
-1.40545368657166));
#43226=CARTESIAN_POINT('Ctrl Pts',(-0.119745364280119,-0.0845575866503699,
-1.40382277756534));
#43227=CARTESIAN_POINT('Ctrl Pts',(-0.0917716266360291,-0.124172310026032,
-1.40117368046269));
#43228=CARTESIAN_POINT('Ctrl Pts',(-0.0421900473124433,-0.148528764690202,
-1.39852458336004));
#43229=CARTESIAN_POINT('Ctrl Pts',(0.00626163154385964,-0.146457262357051,
-1.39587548625739));
#43230=CARTESIAN_POINT('Ctrl Pts',(0.0547133104001626,-0.1443857600239,
-1.39322638915474));
#43231=CARTESIAN_POINT('Ctrl Pts',(0.102035088789183,-0.115886300693427,
-1.39057729205209));
#43232=CARTESIAN_POINT('Ctrl Pts',(0.126525552403112,-0.0740285236635203,
-1.38792819494944));
#43233=CARTESIAN_POINT('Ctrl Pts',(0.151016016017042,-0.032170746633614,
-1.38527909784679));
#43234=CARTESIAN_POINT('Ctrl Pts',(0.152675164855881,0.0230453480957256,
-1.38263000074414));
#43235=CARTESIAN_POINT('Ctrl Pts',(0.130742125647836,0.0662980716748126,
-1.37998090364149));
#43236=CARTESIAN_POINT('Ctrl Pts',(0.10880908643979,0.109550795253901,-1.37733180653884));
#43237=CARTESIAN_POINT('Ctrl Pts',(0.0632838591848581,0.140840147682736,
-1.37468270943619));
#43238=CARTESIAN_POINT('Ctrl Pts',(0.0150439732521744,0.145817065515326,
-1.37203361233353));
#43239=CARTESIAN_POINT('Ctrl Pts',(-0.0331959126805066,0.150793983347916,
-1.36938451523088));
#43240=CARTESIAN_POINT('Ctrl Pts',(-0.0841504572909391,0.129458466584265,
-1.36673541812823));
#43241=CARTESIAN_POINT('Ctrl Pts',(-0.114452286801109,0.0915948239406019,
-1.36408632102558));
#43242=CARTESIAN_POINT('Ctrl Pts',(-0.134930404165678,0.0660063980784996,
-1.36229604887848));
#43243=CARTESIAN_POINT('Ctrl Pts',(-0.145976180189185,0.0328693799721589,
-1.36050577673138));
#43244=CARTESIAN_POINT('Ctrl Pts',(-0.146223843614078,-0.00011741876304885,
-1.35871550458429));
#43245=CARTESIAN_POINT('Origin',(0.,0.,-1.487));
#43246=CARTESIAN_POINT('',(-0.146568201272772,-5.25249794677829E-5,-1.30158449541571));
#43247=CARTESIAN_POINT('',(-0.146583801498189,-2.95221421093228E-5,-1.30871550458428));
#43248=CARTESIAN_POINT('',(-0.14635,-1.79227059055215E-17,-1.487));
#43249=CARTESIAN_POINT('Ctrl Pts',(-0.146568201272772,-5.25249794677829E-5,
-1.30158449541571));
#43250=CARTESIAN_POINT('Ctrl Pts',(-0.146357355089256,0.0455742536737809,
-1.30407582467584));
#43251=CARTESIAN_POINT('Ctrl Pts',(-0.123360881151597,0.0913843415984147,
-1.30656715393598));
#43252=CARTESIAN_POINT('Ctrl Pts',(-0.0865512617525035,0.118312370991474,
-1.30905848319611));
#43253=CARTESIAN_POINT('Ctrl Pts',(-0.0474106079416224,0.146945665589161,
-1.31170758029876));
#43254=CARTESIAN_POINT('Ctrl Pts',(0.00734806976815248,0.154229699641535,
-1.31435667740141));
#43255=CARTESIAN_POINT('Ctrl Pts',(0.0526128505576494,0.136824069508157,
-1.31700577450406));
#43256=CARTESIAN_POINT('Ctrl Pts',(0.0978776313471463,0.119418439374779,
-1.31965487160671));
#43257=CARTESIAN_POINT('Ctrl Pts',(0.133648515216364,0.0773231450556503,
-1.32230396870936));
#43258=CARTESIAN_POINT('Ctrl Pts',(0.143521241855794,0.0298427742803053,
-1.32495306581201));
#43259=CARTESIAN_POINT('Ctrl Pts',(0.153393968495224,-0.0176375964950385,
-1.32760216291466));
#43260=CARTESIAN_POINT('Ctrl Pts',(0.137368537904866,-0.0705030437266001,
-1.33025126001732));
#43261=CARTESIAN_POINT('Ctrl Pts',(0.102794092922157,-0.104509867959372,
-1.33290035711997));
#43262=CARTESIAN_POINT('Ctrl Pts',(0.0682196479394476,-0.138516692192145,
-1.33554945422262));
#43263=CARTESIAN_POINT('Ctrl Pts',(0.0150961885643901,-0.15366489342613,
-1.33819855132527));
#43264=CARTESIAN_POINT('Ctrl Pts',(-0.0322142633050966,-0.14300761965813,
-1.34084764842792));
#43265=CARTESIAN_POINT('Ctrl Pts',(-0.0795247151745847,-0.13235034589013,
-1.34349674553057));
#43266=CARTESIAN_POINT('Ctrl Pts',(-0.1210221595385,-0.095887597120137,
-1.34614584263322));
#43267=CARTESIAN_POINT('Ctrl Pts',(-0.137676178193757,-0.0503409177363263,
-1.34879493973587));
#43268=CARTESIAN_POINT('Ctrl Pts',(-0.143521856995724,-0.0343537098626333,
-1.34972479162915));
#43269=CARTESIAN_POINT('Ctrl Pts',(-0.146306677070172,-0.0172473073728051,
-1.35065464352243));
#43270=CARTESIAN_POINT('Ctrl Pts',(-0.146193053794332,-0.000105164914211059,
-1.35158449541571));
#43271=CARTESIAN_POINT('Ctrl Pts',(-0.146223843614078,-0.00011741876304885,
-1.35871550458429));
#43272=CARTESIAN_POINT('Ctrl Pts',(-0.146342652103738,-0.0159417648008479,
-1.35785667962873));
#43273=CARTESIAN_POINT('Ctrl Pts',(-0.143976502592481,-0.0317315410168582,
-1.35699785467318));
#43274=CARTESIAN_POINT('Ctrl Pts',(-0.138974618193963,-0.0466368226249961,
-1.35613902971763));
#43275=CARTESIAN_POINT('Ctrl Pts',(-0.123546005666741,-0.0926130580232472,
-1.35348993261498));
#43276=CARTESIAN_POINT('Ctrl Pts',(-0.0830396662023916,-0.130173760296071,
-1.35084083551233));
#43277=CARTESIAN_POINT('Ctrl Pts',(-0.0360315046957431,-0.142093871775224,
-1.34819173840968));
#43278=CARTESIAN_POINT('Ctrl Pts',(0.0109766568109053,-0.154013983254376,
-1.34554264130703));
#43279=CARTESIAN_POINT('Ctrl Pts',(0.0644866403598532,-0.140293503939857,
-1.34289354420438));
#43280=CARTESIAN_POINT('Ctrl Pts',(0.0999591669524664,-0.107224543220673,
-1.34024444710173));
#43281=CARTESIAN_POINT('Ctrl Pts',(0.135431693545081,-0.0741555825014888,
-1.33759534999908));
#43282=CARTESIAN_POINT('Ctrl Pts',(0.152866763181359,-0.021738140377639,
-1.33494625289643));
#43283=CARTESIAN_POINT('Ctrl Pts',(0.144268783080492,0.0259895354938695,
-1.33229715579378));
#43284=CARTESIAN_POINT('Ctrl Pts',(0.135670802979624,0.0737172113653767,
-1.32964805869113));
#43285=CARTESIAN_POINT('Ctrl Pts',(0.101039773141612,0.116755120984543,
-1.32699896158848));
#43286=CARTESIAN_POINT('Ctrl Pts',(0.0562572253263671,0.135366400281944,
-1.32434986448583));
#43287=CARTESIAN_POINT('Ctrl Pts',(0.0114746775111209,0.153977679579345,
-1.32170076738318));
#43288=CARTESIAN_POINT('Ctrl Pts',(-0.0434593882813584,0.14816232855498,
-1.31905167028053));
#43289=CARTESIAN_POINT('Ctrl Pts',(-0.0833526195664562,0.120587223776496,
-1.31640257317787));
#43290=CARTESIAN_POINT('Ctrl Pts',(-0.121939603914395,0.0939150264587117,
-1.31384021698001));
#43291=CARTESIAN_POINT('Ctrl Pts',(-0.146454609180979,0.046884730027936,
-1.31127786078215));
#43292=CARTESIAN_POINT('Ctrl Pts',(-0.146583801498189,-2.95221421093228E-5,
-1.30871550458428));
#43293=CARTESIAN_POINT('Origin',(0.,0.,-1.487));
#43294=CARTESIAN_POINT('',(-0.146351269115874,0.000134398057797393,-1.25158449541571));
#43295=CARTESIAN_POINT('',(-0.146311958104459,0.000133832465902105,-1.25871550458429));
#43296=CARTESIAN_POINT('',(-0.14635,-1.79227059055215E-17,-1.487));
#43297=CARTESIAN_POINT('Ctrl Pts',(-0.146351269115874,0.000134398057797393,
-1.25158449541571));
#43298=CARTESIAN_POINT('Ctrl Pts',(-0.146455439504307,0.0114285307963374,
-1.25219881162396));
#43299=CARTESIAN_POINT('Ctrl Pts',(-0.145258679634911,0.0227008231077745,
-1.2528131278322));
#43300=CARTESIAN_POINT('Ctrl Pts',(-0.142677409791644,0.0336466161110121,
-1.25342744404045));
#43301=CARTESIAN_POINT('Ctrl Pts',(-0.131546278346365,0.0808478264027943,
-1.2560765411431));
#43302=CARTESIAN_POINT('Ctrl Pts',(-0.0946692576923265,0.121977563628807,
-1.25872563824575));
#43303=CARTESIAN_POINT('Ctrl Pts',(-0.0489578742111441,0.138174037334444,
-1.2613747353484));
#43304=CARTESIAN_POINT('Ctrl Pts',(-0.00324649072996173,0.154370511040082,
-1.26402383245105));
#43305=CARTESIAN_POINT('Ctrl Pts',(0.0512992555783647,0.145633721225344,
-1.2666729295537));
#43306=CARTESIAN_POINT('Ctrl Pts',(0.0896650926458139,0.115970294478337,
-1.26932202665635));
#43307=CARTESIAN_POINT('Ctrl Pts',(0.128030929713264,0.0863068677313288,
-1.271971123759));
#43308=CARTESIAN_POINT('Ctrl Pts',(0.150216857539836,0.0357168040520492,
-1.27462022086165));
#43309=CARTESIAN_POINT('Ctrl Pts',(0.14604857524424,-0.0125996710156281,
-1.27726931796431));
#43310=CARTESIAN_POINT('Ctrl Pts',(0.141880292948645,-0.060916146083304,
-1.27991841506696));
#43311=CARTESIAN_POINT('Ctrl Pts',(0.111357800530883,-0.106959032539378,
-1.28256751216961));
#43312=CARTESIAN_POINT('Ctrl Pts',(0.0684784851605484,-0.129613406369446,
-1.28521660927226));
#43313=CARTESIAN_POINT('Ctrl Pts',(0.0255991697902121,-0.152267780199515,
-1.28786570637491));
#43314=CARTESIAN_POINT('Ctrl Pts',(-0.0296369685326984,-0.151533641403577,
-1.29051480347756));
#43315=CARTESIAN_POINT('Ctrl Pts',(-0.071899049116112,-0.127747660553035,
-1.29316390058021));
#43316=CARTESIAN_POINT('Ctrl Pts',(-0.114161129699523,-0.103961679702495,
-1.29581299768286));
#43317=CARTESIAN_POINT('Ctrl Pts',(-0.143449152543439,-0.0571238567973552,
-1.29846209478551));
#43318=CARTESIAN_POINT('Ctrl Pts',(-0.146331849009405,-0.00871366777328614,
-1.30111119188816));
#43319=CARTESIAN_POINT('Ctrl Pts',(-0.146503528938243,-0.00583058316663799,
-1.30126895973068));
#43320=CARTESIAN_POINT('Ctrl Pts',(-0.146581553481172,-0.00294192163382165,
-1.30142672757319));
#43321=CARTESIAN_POINT('Ctrl Pts',(-0.146568201272772,-5.25249794677829E-5,
-1.30158449541571));
#43322=CARTESIAN_POINT('Ctrl Pts',(-0.146583801498189,-2.95221421093228E-5,
-1.30871550458428));
#43323=CARTESIAN_POINT('Ctrl Pts',(-0.146588174917659,-0.00161766382360389,
-1.3086287636795));
#43324=CARTESIAN_POINT('Ctrl Pts',(-0.146564603207359,-0.0032056725231908,
-1.30854202277471));
#43325=CARTESIAN_POINT('Ctrl Pts',(-0.146512686262755,-0.00479275398747684,
-1.30845528186992));
#43326=CARTESIAN_POINT('Ctrl Pts',(-0.144927124896243,-0.0532627684403694,
-1.30580618476727));
#43327=CARTESIAN_POINT('Ctrl Pts',(-0.116903605385501,-0.100867938813553,
-1.30315708766462));
#43328=CARTESIAN_POINT('Ctrl Pts',(-0.0752935045800234,-0.125776889350831,
-1.30050799056197));
#43329=CARTESIAN_POINT('Ctrl Pts',(-0.0336834037745442,-0.150685839888109,
-1.29785889345932));
#43330=CARTESIAN_POINT('Ctrl Pts',(0.0215132783256708,-0.152898570589479,
-1.29520979635667));
#43331=CARTESIAN_POINT('Ctrl Pts',(0.0649837553577353,-0.13140033967353,
-1.29256069925402));
#43332=CARTESIAN_POINT('Ctrl Pts',(0.108454232389799,-0.109902108757581,
-1.28991160215137));
#43333=CARTESIAN_POINT('Ctrl Pts',(0.140198504353711,-0.0646929162243153,
-1.28726250504872));
#43334=CARTESIAN_POINT('Ctrl Pts',(0.145658885100711,-0.0165053602787354,
-1.28461340794607));
#43335=CARTESIAN_POINT('Ctrl Pts',(0.151119265847712,0.0316821956668444,
-1.28196431084342));
#43336=CARTESIAN_POINT('Ctrl Pts',(0.130295755377799,0.0828481150247396,
-1.27931521374077));
#43337=CARTESIAN_POINT('Ctrl Pts',(0.092737860143069,0.113528089135675,
-1.27666611663812));
#43338=CARTESIAN_POINT('Ctrl Pts',(0.05517996490834,0.144208063246609,-1.27401701953547));
#43339=CARTESIAN_POINT('Ctrl Pts',(0.00088768490879558,0.154402092110587,
-1.27136792243281));
#43340=CARTESIAN_POINT('Ctrl Pts',(-0.0452409455446037,0.139435270189946,
-1.26871882533016));
#43341=CARTESIAN_POINT('Ctrl Pts',(-0.0913695759980056,0.124468448269304,
-1.26606972822751));
#43342=CARTESIAN_POINT('Ctrl Pts',(-0.12933455690526,0.0843407755640405,
-1.26342063112486));
#43343=CARTESIAN_POINT('Ctrl Pts',(-0.14172543143435,0.0374545032200476,
-1.26077153402221));
#43344=CARTESIAN_POINT('Ctrl Pts',(-0.144931052293872,0.0253246400454748,
-1.26008619087624));
#43345=CARTESIAN_POINT('Ctrl Pts',(-0.146424999918828,0.0127424242477569,
-1.25940084773026));
#43346=CARTESIAN_POINT('Ctrl Pts',(-0.146311958104459,0.000133832465902105,
-1.25871550458429));
#43347=CARTESIAN_POINT('Origin',(0.,0.,-1.487));
#43348=CARTESIAN_POINT('',(-0.146110748319233,-1.87736639323394E-5,-1.20158449541571));
#43349=CARTESIAN_POINT('',(-0.146118579951279,-3.98722473775574E-5,-1.20871550458429));
#43350=CARTESIAN_POINT('',(-0.14635,-1.79227059055215E-17,-1.487));
#43351=CARTESIAN_POINT('Ctrl Pts',(-0.146110748319233,-1.87736639323394E-5,
-1.20158449541571));
#43352=CARTESIAN_POINT('Ctrl Pts',(-0.146081502410529,0.0255760520854927,
-1.20297089567472));
#43353=CARTESIAN_POINT('Ctrl Pts',(-0.139689794215594,0.0511845413353593,
-1.20435729593373));
#43354=CARTESIAN_POINT('Ctrl Pts',(-0.127020288822047,0.0731763914670449,
-1.20574369619274));
#43355=CARTESIAN_POINT('Ctrl Pts',(-0.102811731580409,0.115197839520859,
-1.20839279329539));
#43356=CARTESIAN_POINT('Ctrl Pts',(-0.0556825852416403,0.144014735640639,
-1.21104189039804));
#43357=CARTESIAN_POINT('Ctrl Pts',(-0.00724592449332075,0.146411866386614,
-1.21369098750069));
#43358=CARTESIAN_POINT('Ctrl Pts',(0.0411907362549988,0.148808997132589,
-1.21634008460334));
#43359=CARTESIAN_POINT('Ctrl Pts',(0.090934911412867,0.124786362504761,
-1.21898918170599));
#43360=CARTESIAN_POINT('Ctrl Pts',(0.119174293597701,0.0853605634122892,
-1.22163827880864));
#43361=CARTESIAN_POINT('Ctrl Pts',(0.147413675782537,0.0459347643198159,
-1.22428737591129));
#43362=CARTESIAN_POINT('Ctrl Pts',(0.154148264994333,-0.00889419923730254,
-1.22693647301394));
#43363=CARTESIAN_POINT('Ctrl Pts',(0.136289628894883,-0.0539821738749891,
-1.2295855701166));
#43364=CARTESIAN_POINT('Ctrl Pts',(0.118430992795435,-0.0990701485126745,
-1.23223466721925));
#43365=CARTESIAN_POINT('Ctrl Pts',(0.0759791313847414,-0.13441713423093,
-1.2348837643219));
#43366=CARTESIAN_POINT('Ctrl Pts',(0.0284021513987267,-0.143813267247839,
-1.23753286142455));
#43367=CARTESIAN_POINT('Ctrl Pts',(-0.0191748285872881,-0.153209400264748,
-1.2401819585272));
#43368=CARTESIAN_POINT('Ctrl Pts',(-0.0718769271486259,-0.136654680580311,
-1.24283105562985));
#43369=CARTESIAN_POINT('Ctrl Pts',(-0.105535355311034,-0.101740979059317,
-1.2454801527325));
#43370=CARTESIAN_POINT('Ctrl Pts',(-0.131388513540689,-0.0749236409040759,
-1.2475149336269));
#43371=CARTESIAN_POINT('Ctrl Pts',(-0.146006228706228,-0.0372748143425158,
-1.24954971452131));
#43372=CARTESIAN_POINT('Ctrl Pts',(-0.146351269115874,0.000134398057797393,
-1.25158449541571));
#43373=CARTESIAN_POINT('Ctrl Pts',(-0.146311958104459,0.000133832465902105,
-1.25871550458429));
#43374=CARTESIAN_POINT('Ctrl Pts',(-0.1459880527564,-0.0359943058909224,
-1.25675175062761));
#43375=CARTESIAN_POINT('Ctrl Pts',(-0.132470313237583,-0.0723389984778341,
-1.25478799667094));
#43376=CARTESIAN_POINT('Ctrl Pts',(-0.108221467599082,-0.0988789749007037,
-1.25282424271426));
#43377=CARTESIAN_POINT('Ctrl Pts',(-0.0755098610837993,-0.134681308694744,
-1.25017514561161));
#43378=CARTESIAN_POINT('Ctrl Pts',(-0.023269879902309,-0.152641104300106,
-1.24752604850896));
#43379=CARTESIAN_POINT('Ctrl Pts',(0.0245416105517876,-0.144522133523684,
-1.24487695140631));
#43380=CARTESIAN_POINT('Ctrl Pts',(0.0723531010058841,-0.136403162747262,
-1.24222785430366));
#43381=CARTESIAN_POINT('Ctrl Pts',(0.115736100732587,-0.102205425589056,
-1.23957875720101));
#43382=CARTESIAN_POINT('Ctrl Pts',(0.134795489915285,-0.0576117490205896,
-1.23692966009836));
#43383=CARTESIAN_POINT('Ctrl Pts',(0.153854879097983,-0.0130180724521228,
-1.23428056299571));
#43384=CARTESIAN_POINT('Ctrl Pts',(0.148590657736676,0.0419715435266052,
-1.23163146589306));
#43385=CARTESIAN_POINT('Ctrl Pts',(0.121416958449766,0.0821392715302546,
-1.22898236879041));
#43386=CARTESIAN_POINT('Ctrl Pts',(0.0942432591628547,0.122306999533906,
-1.22633327168776));
#43387=CARTESIAN_POINT('Ctrl Pts',(0.0451600819503379,0.147652839562477,
-1.2236841745851));
#43388=CARTESIAN_POINT('Ctrl Pts',(-0.00332339452852188,0.146553378587874,
-1.22103507748245));
#43389=CARTESIAN_POINT('Ctrl Pts',(-0.0518068710073776,0.145453917613272,
-1.2183859803798));
#43390=CARTESIAN_POINT('Ctrl Pts',(-0.0996906467525764,0.1179091556355,
-1.21573688327715));
#43391=CARTESIAN_POINT('Ctrl Pts',(-0.12501557966413,0.0765509148734009,
-1.2130877861745));
#43392=CARTESIAN_POINT('Ctrl Pts',(-0.138948344130923,0.0537972661544986,
-1.21163035897776));
#43393=CARTESIAN_POINT('Ctrl Pts',(-0.146053088318131,0.0268626089518478,
-1.21017293178102));
#43394=CARTESIAN_POINT('Ctrl Pts',(-0.146118579951279,-3.98722473775574E-5,
-1.20871550458429));
#43395=CARTESIAN_POINT('Origin',(0.,0.,-1.487));
#43396=CARTESIAN_POINT('',(-0.146420343877387,-0.000126359191821662,-1.15158449541571));
#43397=CARTESIAN_POINT('',(-0.146458539542634,-0.000116607055467748,-1.15871550458429));
#43398=CARTESIAN_POINT('',(-0.14635,-1.79227059055215E-17,-1.487));
#43399=CARTESIAN_POINT('Ctrl Pts',(-0.146420343877387,-0.000126359191821662,
-1.15158449541571));
#43400=CARTESIAN_POINT('Ctrl Pts',(-0.146059012458362,0.0395090623243778,
-1.15374297972548));
#43401=CARTESIAN_POINT('Ctrl Pts',(-0.129398885067076,0.0794119747695151,
-1.15590146403526));
#43402=CARTESIAN_POINT('Ctrl Pts',(-0.100677635328534,0.106550231277221,
-1.15805994834503));
#43403=CARTESIAN_POINT('Ctrl Pts',(-0.0654281877775973,0.139856879076344,
-1.16070904544768));
#43404=CARTESIAN_POINT('Ctrl Pts',(-0.0120116369076935,0.153936723882358,
-1.16335814255033));
#43405=CARTESIAN_POINT('Ctrl Pts',(0.0350755858116793,0.142332853974555,
-1.16600723965298));
#43406=CARTESIAN_POINT('Ctrl Pts',(0.0821628085310534,0.130728984066752,
-1.16865633675563));
#43407=CARTESIAN_POINT('Ctrl Pts',(0.122920703099893,0.0934413994451258,
-1.17130543385828));
#43408=CARTESIAN_POINT('Ctrl Pts',(0.13865800333033,0.047569908061934,-1.17395453096093));
#43409=CARTESIAN_POINT('Ctrl Pts',(0.154395303560766,0.00169841667874217,
-1.17660362806358));
#43410=CARTESIAN_POINT('Ctrl Pts',(0.145112009452802,-0.0527569814660171,
-1.17925272516623));
#43411=CARTESIAN_POINT('Ctrl Pts',(0.115065370383711,-0.0908234472976769,
-1.18190182226889));
#43412=CARTESIAN_POINT('Ctrl Pts',(0.0850187313146192,-0.128889913129339,
-1.18455091937154));
#43413=CARTESIAN_POINT('Ctrl Pts',(0.0342087472843984,-0.1505674466479,
-1.18720001647419));
#43414=CARTESIAN_POINT('Ctrl Pts',(-0.0140635023318603,-0.145914892806514,
-1.18984911357684));
#43415=CARTESIAN_POINT('Ctrl Pts',(-0.062335751948115,-0.141262338965128,
-1.19249821067949));
#43416=CARTESIAN_POINT('Ctrl Pts',(-0.108070267150408,-0.1102796977638,
-1.19514730778214));
#43417=CARTESIAN_POINT('Ctrl Pts',(-0.130293540679301,-0.0671753771692121,
-1.19779640488479));
#43418=CARTESIAN_POINT('Ctrl Pts',(-0.140886303516203,-0.0466296261253513,
-1.19905910172843));
#43419=CARTESIAN_POINT('Ctrl Pts',(-0.146137384722659,-0.0233298668906606,
-1.20032179857207));
#43420=CARTESIAN_POINT('Ctrl Pts',(-0.146110748319233,-1.87736639323394E-5,
-1.20158449541571));
#43421=CARTESIAN_POINT('Ctrl Pts',(-0.146118579951279,-3.98722473775574E-5,
-1.20871550458429));
#43422=CARTESIAN_POINT('Ctrl Pts',(-0.146172129389966,-0.0220367701447063,
-1.20752383467837));
#43423=CARTESIAN_POINT('Ctrl Pts',(-0.141519539811635,-0.0440121565613824,
-1.20633216477246));
#43424=CARTESIAN_POINT('Ctrl Pts',(-0.132045341637239,-0.0636629050438161,
-1.20514049486655));
#43425=CARTESIAN_POINT('Ctrl Pts',(-0.110984080620887,-0.107346764652504,
-1.2024913977639));
#43426=CARTESIAN_POINT('Ctrl Pts',(-0.0660954685102728,-0.139542764323454,
-1.19984230066125));
#43427=CARTESIAN_POINT('Ctrl Pts',(-0.0179650877217393,-0.145486058953644,
-1.1971932035586));
#43428=CARTESIAN_POINT('Ctrl Pts',(0.0301652930667956,-0.151429353583835,
-1.19454410645595));
#43429=CARTESIAN_POINT('Ctrl Pts',(0.0815374425332507,-0.131119943173266,
-1.1918950093533));
#43430=CARTESIAN_POINT('Ctrl Pts',(0.112592476430099,-0.0938715717246213,
-1.18924591225065));
#43431=CARTESIAN_POINT('Ctrl Pts',(0.143647510326947,-0.0566232002759764,
-1.186596815148));
#43432=CARTESIAN_POINT('Ctrl Pts',(0.154385428654186,-0.00243586778925729,
-1.18394771804535));
#43433=CARTESIAN_POINT('Ctrl Pts',(0.139881902226487,0.0438405195705144,
-1.1812986209427));
#43434=CARTESIAN_POINT('Ctrl Pts',(0.125378375798787,0.090116906930286,
-1.17864952384005));
#43435=CARTESIAN_POINT('Ctrl Pts',(0.0856334046161455,0.12848234916311,
-1.1760004267374));
#43436=CARTESIAN_POINT('Ctrl Pts',(0.0388737357630849,0.141342740862539,
-1.17335132963475));
#43437=CARTESIAN_POINT('Ctrl Pts',(-0.00788593308997566,0.154203132561969,
-1.17070223253209));
#43438=CARTESIAN_POINT('Ctrl Pts',(-0.061660299613454,0.141558473728007,
-1.16805313542944));
#43439=CARTESIAN_POINT('Ctrl Pts',(-0.0977888407502427,0.109207510508375,
-1.16540403832679));
#43440=CARTESIAN_POINT('Ctrl Pts',(-0.128195045467967,0.0819805597508731,
-1.16317452707929));
#43441=CARTESIAN_POINT('Ctrl Pts',(-0.146102529657357,0.0407954298906481,
-1.16094501583179));
#43442=CARTESIAN_POINT('Ctrl Pts',(-0.146458539542634,-0.000116607055467748,
-1.15871550458429));
#43443=CARTESIAN_POINT('Origin',(0.,0.,-1.487));
#43444=CARTESIAN_POINT('',(-0.146524574873171,8.77098538252519E-5,-1.10158449541571));
#43445=CARTESIAN_POINT('',(-0.1464923466868,0.000104122940576147,-1.10871550458429));
#43446=CARTESIAN_POINT('',(-0.14635,-1.79227059055215E-17,-1.487));
#43447=CARTESIAN_POINT('Ctrl Pts',(-0.146524574873171,8.77098538252519E-5,
-1.10158449541571));
#43448=CARTESIAN_POINT('Ctrl Pts',(-0.146561083382481,0.00524669631098321,
-1.1018659666736));
#43449=CARTESIAN_POINT('Ctrl Pts',(-0.146312285983159,0.0104021223371573,
-1.10214743793148));
#43450=CARTESIAN_POINT('Ctrl Pts',(-0.145766538895233,0.0155259195888394,
-1.10242890918937));
#43451=CARTESIAN_POINT('Ctrl Pts',(-0.140630181313775,0.063749090067944,
-1.10507800629202));
#43452=CARTESIAN_POINT('Ctrl Pts',(-0.10919050657635,0.109170635495247,
-1.10772710339467));
#43453=CARTESIAN_POINT('Ctrl Pts',(-0.0658655148174998,0.13096057421377,
-1.11037620049732));
#43454=CARTESIAN_POINT('Ctrl Pts',(-0.0225405230586548,0.15275051293229,
-1.11302529759997));
#43455=CARTESIAN_POINT('Ctrl Pts',(0.0326697857216125,0.150908844942036,
-1.11567439470262));
#43456=CARTESIAN_POINT('Ctrl Pts',(0.0744463760666706,0.126280145435118,
-1.11832349180527));
#43457=CARTESIAN_POINT('Ctrl Pts',(0.116222966411732,0.101651445928197,
-1.12097258890792));
#43458=CARTESIAN_POINT('Ctrl Pts',(0.144565838321582,0.0542357149046093,
-1.12362168601057));
#43459=CARTESIAN_POINT('Ctrl Pts',(0.146477162320489,0.0057774526490098,
-1.12627078311322));
#43460=CARTESIAN_POINT('Ctrl Pts',(0.148388486319397,-0.0426808096065883,
-1.12891988021587));
#43461=CARTESIAN_POINT('Ctrl Pts',(0.123868262407364,-0.0921816030941977,
-1.13156897731853));
#43462=CARTESIAN_POINT('Ctrl Pts',(0.0841612822247374,-0.120024233448344,
-1.13421807442118));
#43463=CARTESIAN_POINT('Ctrl Pts',(0.0444543020421122,-0.14786686380249,
-1.13686717152383));
#43464=CARTESIAN_POINT('Ctrl Pts',(-0.010439434411105,-0.154051331023175,
-1.13951626862648));
#43465=CARTESIAN_POINT('Ctrl Pts',(-0.0553460693842255,-0.135741484610605,
-1.14216536572913));
#43466=CARTESIAN_POINT('Ctrl Pts',(-0.10025270435735,-0.117431638198033,
-1.14481446283178));
#43467=CARTESIAN_POINT('Ctrl Pts',(-0.135172237850375,-0.0746274781522026,
-1.14746355993443));
#43468=CARTESIAN_POINT('Ctrl Pts',(-0.144090832480906,-0.0269586727331693,
-1.15011265703708));
#43469=CARTESIAN_POINT('Ctrl Pts',(-0.14574255623835,-0.0181304097992216,
-1.15060326982996));
#43470=CARTESIAN_POINT('Ctrl Pts',(-0.146502472719297,-0.00913529419259381,
-1.15109388262283));
#43471=CARTESIAN_POINT('Ctrl Pts',(-0.146420343877387,-0.000126359191821662,
-1.15158449541571));
#43472=CARTESIAN_POINT('Ctrl Pts',(-0.146458539542634,-0.000116607055467748,
-1.15871550458429));
#43473=CARTESIAN_POINT('Ctrl Pts',(-0.146525539299788,-0.00781610264093099,
-1.15829591872914));
#43474=CARTESIAN_POINT('Ctrl Pts',(-0.14597090336011,-0.0155059258592174,
-1.15787633287399));
#43475=CARTESIAN_POINT('Ctrl Pts',(-0.1447609525327,-0.0230912179959941,
-1.15745674701884));
#43476=CARTESIAN_POINT('Ctrl Pts',(-0.137121807428272,-0.0709817156754305,
-1.15480764991619));
#43477=CARTESIAN_POINT('Ctrl Pts',(-0.10336080146932,-0.114705443429,-1.15215855281354));
#43478=CARTESIAN_POINT('Ctrl Pts',(-0.0589604799596247,-0.134211026110539,
-1.14950945571089));
#43479=CARTESIAN_POINT('Ctrl Pts',(-0.0145601584499285,-0.153716608792078,
-1.14686035860824));
#43480=CARTESIAN_POINT('Ctrl Pts',(0.0404794786105083,-0.149004046401583,
-1.14421126150559));
#43481=CARTESIAN_POINT('Ctrl Pts',(0.0809176645416876,-0.122234484871627,
-1.14156216440294));
#43482=CARTESIAN_POINT('Ctrl Pts',(0.121355850472866,-0.0954649233416712,
-1.13891306730029));
#43483=CARTESIAN_POINT('Ctrl Pts',(0.147192585274786,-0.0466383626722524,
-1.13626397019764));
#43484=CARTESIAN_POINT('Ctrl Pts',(0.14657933524087,0.00185370090836365,
-1.13361487309499));
#43485=CARTESIAN_POINT('Ctrl Pts',(0.145966085206954,0.0503457644889783,
-1.13096577599234));
#43486=CARTESIAN_POINT('Ctrl Pts',(0.118902850337209,0.0985033309807881,
-1.12831667888969));
#43487=CARTESIAN_POINT('Ctrl Pts',(0.077800628113376,0.124241699891289,
-1.12566758178703));
#43488=CARTESIAN_POINT('Ctrl Pts',(0.0366984058895428,0.149980068801791,
-1.12301848468438));
#43489=CARTESIAN_POINT('Ctrl Pts',(-0.0184428036883855,0.153299240130978,
-1.12036938758173));
#43490=CARTESIAN_POINT('Ctrl Pts',(-0.0623356535421235,0.132677066685202,
-1.11772029047908));
#43491=CARTESIAN_POINT('Ctrl Pts',(-0.106228503395864,0.112054893239424,
-1.11507119337643));
#43492=CARTESIAN_POINT('Ctrl Pts',(-0.13887299352542,0.0674913750186834,
-1.11242209627378));
#43493=CARTESIAN_POINT('Ctrl Pts',(-0.145298604451477,0.0194230088082777,
-1.10977299917113));
#43494=CARTESIAN_POINT('Ctrl Pts',(-0.146153618884468,0.0130268626125056,
-1.10942050097552));
#43495=CARTESIAN_POINT('Ctrl Pts',(-0.146544404427699,0.00656865992383821,
-1.1090680027799));
#43496=CARTESIAN_POINT('Ctrl Pts',(-0.1464923466868,0.000104122940576147,
-1.10871550458429));
#43497=CARTESIAN_POINT('Origin',(0.,0.,-1.487));
#43498=CARTESIAN_POINT('',(-0.146149474112214,7.75799253666179E-5,-1.05158449541571));
#43499=CARTESIAN_POINT('',(-0.146131080621407,5.8892630247073E-5,-1.05871550458429));
#43500=CARTESIAN_POINT('',(-0.14635,-1.79227059055215E-17,-1.487));
#43501=CARTESIAN_POINT('Ctrl Pts',(-0.146149474112214,7.75799253666179E-5,
-1.05158449541571));
#43502=CARTESIAN_POINT('Ctrl Pts',(-0.146242719876307,0.0195147651561755,
-1.05263805072436));
#43503=CARTESIAN_POINT('Ctrl Pts',(-0.142640298356387,0.0389187871975207,
-1.05369160603301));
#43504=CARTESIAN_POINT('Ctrl Pts',(-0.135179691770213,0.0567043999481941,
-1.05474516134166));
#43505=CARTESIAN_POINT('Ctrl Pts',(-0.11642047606583,0.101425179977368,
-1.05739425844431));
#43506=CARTESIAN_POINT('Ctrl Pts',(-0.0732683212642689,0.135913750150424,
-1.06004335554696));
#43507=CARTESIAN_POINT('Ctrl Pts',(-0.0255124834227526,0.144353909646322,
-1.06269245264961));
#43508=CARTESIAN_POINT('Ctrl Pts',(0.022243354418761,0.152794069142219,
-1.06534154975226));
#43509=CARTESIAN_POINT('Ctrl Pts',(0.0746028753002338,0.135185817960959,
-1.06799064685491));
#43510=CARTESIAN_POINT('Ctrl Pts',(0.107554393814019,0.0996041686470673,
-1.07063974395756));
#43511=CARTESIAN_POINT('Ctrl Pts',(0.140505912327805,0.0640225193331759,
-1.07328884106021));
#43512=CARTESIAN_POINT('Ctrl Pts',(0.154049428473909,0.0104674718866523,
-1.07593793816287));
#43513=CARTESIAN_POINT('Ctrl Pts',(0.141973986851311,-0.0365010287268484,
-1.07858703526552));
#43514=CARTESIAN_POINT('Ctrl Pts',(0.129898545228714,-0.083469529340349,
-1.08123613236817));
#43515=CARTESIAN_POINT('Ctrl Pts',(0.0922041458374203,-0.123851483120823,
-1.08388522947082));
#43516=CARTESIAN_POINT('Ctrl Pts',(0.0461771588461381,-0.139128027519523,
-1.08653432657347));
#43517=CARTESIAN_POINT('Ctrl Pts',(0.00015017185485576,-0.154404571918223,
-1.08918342367612));
#43518=CARTESIAN_POINT('Ctrl Pts',(-0.0542094027364084,-0.144575706935147,
-1.09183252077877));
#43519=CARTESIAN_POINT('Ctrl Pts',(-0.0919726698192958,-0.114148876678158,
-1.09448161788142));
#43520=CARTESIAN_POINT('Ctrl Pts',(-0.125723522907594,-0.0869549510124533,
-1.09684924372618));
#43521=CARTESIAN_POINT('Ctrl Pts',(-0.146217479609366,-0.0433076611709086,
-1.09921686957095));
#43522=CARTESIAN_POINT('Ctrl Pts',(-0.146524574873171,8.77098538252519E-5,
-1.10158449541571));
#43523=CARTESIAN_POINT('Ctrl Pts',(-0.1464923466868,0.000104122940576147,
-1.10871550458429));
#43524=CARTESIAN_POINT('Ctrl Pts',(-0.146153179700024,-0.0420136772493715,
-1.10641890567725));
#43525=CARTESIAN_POINT('Ctrl Pts',(-0.127016232218379,-0.0844003551295632,
-1.10412230677021));
#43526=CARTESIAN_POINT('Ctrl Pts',(-0.0949958446926328,-0.111645542758528,
-1.10182570786318));
#43527=CARTESIAN_POINT('Ctrl Pts',(-0.0580607422851733,-0.143072513914862,
-1.09917661076053));
#43528=CARTESIAN_POINT('Ctrl Pts',(-0.00398380574769549,-0.154353242027462,
-1.09652751365788));
#43529=CARTESIAN_POINT('Ctrl Pts',(0.0424356855129829,-0.140314469395556,
-1.09387841655523));
#43530=CARTESIAN_POINT('Ctrl Pts',(0.0888551767736612,-0.126275696763649,
-1.09122931945258));
#43531=CARTESIAN_POINT('Ctrl Pts',(0.12761722275754,-0.086917423387236,
-1.08858022234993));
#43532=CARTESIAN_POINT('Ctrl Pts',(0.140945838538626,-0.0402890596236343,
-1.08593112524728));
#43533=CARTESIAN_POINT('Ctrl Pts',(0.154274454319711,0.00633930413996739,
-1.08328202814463));
#43534=CARTESIAN_POINT('Ctrl Pts',(0.142169639898003,0.0602377582907576,
-1.08063293104198));
#43535=CARTESIAN_POINT('Ctrl Pts',(0.110182572803752,0.096688874112066,
-1.07798383393933));
#43536=CARTESIAN_POINT('Ctrl Pts',(0.0781955057095002,0.133139989933375,
-1.07533473683668));
#43537=CARTESIAN_POINT('Ctrl Pts',(0.0263261859427038,0.152143767425202,
-1.07268563973402));
#43538=CARTESIAN_POINT('Ctrl Pts',(-0.0216385036607916,0.144985216094728,
-1.07003654263137));
#43539=CARTESIAN_POINT('Ctrl Pts',(-0.0696031932642857,0.137826664764254,
-1.06738744552872));
#43540=CARTESIAN_POINT('Ctrl Pts',(-0.113663252704479,0.104505784611482,
-1.06473834842607));
#43541=CARTESIAN_POINT('Ctrl Pts',(-0.133613067634466,0.0603032825310584,
-1.06208925132342));
#43542=CARTESIAN_POINT('Ctrl Pts',(-0.142082069267649,0.0415386441810969,
-1.06096466907704));
#43543=CARTESIAN_POINT('Ctrl Pts',(-0.146206085659769,0.0208129935048418,
-1.05984008683066));
#43544=CARTESIAN_POINT('Ctrl Pts',(-0.146131080621407,5.8892630247073E-5,
-1.05871550458429));
#43545=CARTESIAN_POINT('Origin',(0.,0.,-1.487));
#43546=CARTESIAN_POINT('',(-0.14624049998758,-0.000122393304379964,-1.00158449541571));
#43547=CARTESIAN_POINT('',(-0.146276158903947,-0.000129924306316357,-1.00871550458429));
#43548=CARTESIAN_POINT('',(-0.14635,-1.79227059055215E-17,-1.487));
#43549=CARTESIAN_POINT('Ctrl Pts',(-0.14624049998758,-0.000122393304379964,
-1.00158449541571));
#43550=CARTESIAN_POINT('Ctrl Pts',(-0.145975166651522,0.0335064020248649,
-1.00341013477512));
#43551=CARTESIAN_POINT('Ctrl Pts',(-0.134449619835993,0.0672994560490952,
-1.00523577413454));
#43552=CARTESIAN_POINT('Ctrl Pts',(-0.113220905513423,0.0931126446584736,
-1.00706141349395));
#43553=CARTESIAN_POINT('Ctrl Pts',(-0.0824169434302395,0.130568915965678,
-1.0097105105966));
#43554=CARTESIAN_POINT('Ctrl Pts',(-0.0311824668478037,0.151223173297353,
-1.01235960769925));
#43555=CARTESIAN_POINT('Ctrl Pts',(0.0169867757432259,0.145603528427109,
-1.0150087048019));
#43556=CARTESIAN_POINT('Ctrl Pts',(0.0651560183342582,0.139983883556864,
-1.01765780190455));
#43557=CARTESIAN_POINT('Ctrl Pts',(0.110260026933884,0.108090336484698,
-1.0203068990072));
#43558=CARTESIAN_POINT('Ctrl Pts',(0.131614439903856,0.0645490298096645,
-1.02295599610985));
#43559=CARTESIAN_POINT('Ctrl Pts',(0.152968852873826,0.0210077231346337,
-1.0256050932125));
#43560=CARTESIAN_POINT('Ctrl Pts',(0.150573670214146,-0.0341813431432621,
-1.02825419031516));
#43561=CARTESIAN_POINT('Ctrl Pts',(0.125527304812286,-0.0757088752203993,
-1.03090328741781));
#43562=CARTESIAN_POINT('Ctrl Pts',(0.100480939410427,-0.117236407297537,
-1.03355238452046));
#43563=CARTESIAN_POINT('Ctrl Pts',(0.0527833912663882,-0.145102405173915,
-1.03620148162311));
#43564=CARTESIAN_POINT('Ctrl Pts',(0.00430839989247441,-0.146527730245647,
-1.03885057872576));
#43565=CARTESIAN_POINT('Ctrl Pts',(-0.044166591481438,-0.147953055317379,
-1.04149967582841));
#43566=CARTESIAN_POINT('Ctrl Pts',(-0.0934190260852259,-0.122937707584465,
-1.04414877293106));
#43567=CARTESIAN_POINT('Ctrl Pts',(-0.120862105083515,-0.0829535387753645,
-1.04679787003371));
#43568=CARTESIAN_POINT('Ctrl Pts',(-0.137390974279754,-0.0588712156436504,
-1.04839341182771));
#43569=CARTESIAN_POINT('Ctrl Pts',(-0.146008259396191,-0.0293587877137046,
-1.04998895362171));
#43570=CARTESIAN_POINT('Ctrl Pts',(-0.146149474112214,7.75799253666179E-5,
-1.05158449541571));
#43571=CARTESIAN_POINT('Ctrl Pts',(-0.146131080621407,5.8892630247073E-5,
-1.05871550458429));
#43572=CARTESIAN_POINT('Ctrl Pts',(-0.146029401712954,-0.0280759416282176,
-1.05719098972801));
#43573=CARTESIAN_POINT('Ctrl Pts',(-0.138211069888345,-0.0562630595698258,
-1.05566647487174));
#43574=CARTESIAN_POINT('Ctrl Pts',(-0.123039720841311,-0.0796879214310764,
-1.05414196001547));
#43575=CARTESIAN_POINT('Ctrl Pts',(-0.0966769886983866,-0.120392499304715,
-1.05149286291282));
#43576=CARTESIAN_POINT('Ctrl Pts',(-0.0481119539927562,-0.146717531043917,
-1.04884376581017));
#43577=CARTESIAN_POINT('Ctrl Pts',(0.00038382090199534,-0.146590553611849,
-1.04619466870752));
#43578=CARTESIAN_POINT('Ctrl Pts',(0.0488795957967455,-0.14646357617978,
-1.04354557160487));
#43579=CARTESIAN_POINT('Ctrl Pts',(0.0973061108806183,-0.119884589576444,
-1.04089647450222));
#43580=CARTESIAN_POINT('Ctrl Pts',(0.123455327844505,-0.0790425186435681,
-1.03824737739957));
#43581=CARTESIAN_POINT('Ctrl Pts',(0.149604544808393,-0.0382004477106907,
-1.03559828029692));
#43582=CARTESIAN_POINT('Ctrl Pts',(0.153476463652296,0.0169047075517241,
-1.03294918319427));
#43583=CARTESIAN_POINT('Ctrl Pts',(0.133295451298627,0.0610021343053538,
-1.03030008609162));
#43584=CARTESIAN_POINT('Ctrl Pts',(0.113114438944959,0.105099561058982,
-1.02765098898896));
#43585=CARTESIAN_POINT('Ctrl Pts',(0.0688804953937197,0.138189259303824,
-1.02500189188631));
#43586=CARTESIAN_POINT('Ctrl Pts',(0.0208789769470806,0.145096540442412,
-1.02235279478366));
#43587=CARTESIAN_POINT('Ctrl Pts',(-0.0271225414995586,0.152003821581,-1.01970369768101));
#43588=CARTESIAN_POINT('Ctrl Pts',(-0.078891634841599,0.132728685613335,
-1.01705460057836));
#43589=CARTESIAN_POINT('Ctrl Pts',(-0.110687383333389,0.0961105660035381,
-1.01440550347571));
#43590=CARTESIAN_POINT('Ctrl Pts',(-0.133452092296473,0.0698931981089703,
-1.01250883717857));
#43591=CARTESIAN_POINT('Ctrl Pts',(-0.145978287949379,0.0347856633350198,
-1.01061217088143));
#43592=CARTESIAN_POINT('Ctrl Pts',(-0.146276158903947,-0.000129924306316357,
-1.00871550458429));
#43593=CARTESIAN_POINT('Origin',(0.,0.,-1.487));
#43594=CARTESIAN_POINT('',(-0.146588451745324,-1.75972019087617E-5,-0.951584495415713));
#43595=CARTESIAN_POINT('',(-0.146590666816024,6.75222312525112E-6,-0.958715504584286));
#43596=CARTESIAN_POINT('',(-0.14635,-1.79227059055215E-17,-1.487));
#43597=CARTESIAN_POINT('Ctrl Pts',(-0.146588451745324,-1.75972019087617E-5,
-0.951584495415713));
#43598=CARTESIAN_POINT('Ctrl Pts',(-0.146507854065706,0.0475401451251456,
-0.954182218825889));
#43599=CARTESIAN_POINT('Ctrl Pts',(-0.121214084826491,0.0951714550570576,
-0.956779942236065));
#43600=CARTESIAN_POINT('Ctrl Pts',(-0.0817374545005452,0.121687824256767,
-0.959377665646241));
#43601=CARTESIAN_POINT('Ctrl Pts',(-0.0414801173994512,0.148728592548183,
-0.962026762748892));
#43602=CARTESIAN_POINT('Ctrl Pts',(0.0135266004960519,0.153811005652573,
-0.964675859851542));
#43603=CARTESIAN_POINT('Ctrl Pts',(0.05805702898926,0.134604306860943,-0.967324956954193));
#43604=CARTESIAN_POINT('Ctrl Pts',(0.102587457482468,0.115397608069312,
-0.969974054056843));
#43605=CARTESIAN_POINT('Ctrl Pts',(0.13664159657338,0.071901797381661,-0.972623151159494));
#43606=CARTESIAN_POINT('Ctrl Pts',(0.144602472292162,0.0240637288791464,
-0.975272248262145));
#43607=CARTESIAN_POINT('Ctrl Pts',(0.152563348010944,-0.0237743396233668,
-0.977921345364795));
#43608=CARTESIAN_POINT('Ctrl Pts',(0.134430960357596,-0.0759546659407451,
-0.980570442467445));
#43609=CARTESIAN_POINT('Ctrl Pts',(0.0985206869500141,-0.108547741954736,
-0.983219539570096));
#43610=CARTESIAN_POINT('Ctrl Pts',(0.0626104135424317,-0.141140817968727,
-0.985868636672746));
#43611=CARTESIAN_POINT('Ctrl Pts',(0.00892225438061556,-0.154146643679333,
-0.988517733775397));
#43612=CARTESIAN_POINT('Ctrl Pts',(-0.0379228015308373,-0.141600844505346,
-0.991166830878048));
#43613=CARTESIAN_POINT('Ctrl Pts',(-0.0847678574422902,-0.12905504533136,
-0.993815927980698));
#43614=CARTESIAN_POINT('Ctrl Pts',(-0.124769810103378,-0.0909576212727806,
-0.996465025083348));
#43615=CARTESIAN_POINT('Ctrl Pts',(-0.139584062641958,-0.0447797666021233,
-0.999114122185999));
#43616=CARTESIAN_POINT('Ctrl Pts',(-0.144188994243358,-0.0304256261077581,
-0.999937579929236));
#43617=CARTESIAN_POINT('Ctrl Pts',(-0.146360179040833,-0.0152907187279361,
-1.00076103767247));
#43618=CARTESIAN_POINT('Ctrl Pts',(-0.14624049998758,-0.000122393304379964,
-1.00158449541571));
#43619=CARTESIAN_POINT('Ctrl Pts',(-0.146276158903947,-0.000129924306316357,
-1.00871550458429));
#43620=CARTESIAN_POINT('Ctrl Pts',(-0.146394327968595,-0.0139813665834068,
-1.00796307377878));
#43621=CARTESIAN_POINT('Ctrl Pts',(-0.144587995579233,-0.0278026000996961,
-1.00721064297327));
#43622=CARTESIAN_POINT('Ctrl Pts',(-0.140732928203323,-0.0410265846254768,
-1.00645821216776));
#43623=CARTESIAN_POINT('Ctrl Pts',(-0.127160320939926,-0.0875845123927666,
-1.00380911506511));
#43624=CARTESIAN_POINT('Ctrl Pts',(-0.0881927027715921,-0.126739264675417,
-1.00116001796246));
#43625=CARTESIAN_POINT('Ctrl Pts',(-0.0417003324934901,-0.140534764370406,
-0.99851092085981));
#43626=CARTESIAN_POINT('Ctrl Pts',(0.00479203778461458,-0.154330264065396,
-0.99586182375716));
#43627=CARTESIAN_POINT('Ctrl Pts',(0.0588091601724866,-0.142766511172721,
-0.993212726654508));
#43628=CARTESIAN_POINT('Ctrl Pts',(0.0955791855857983,-0.111146556444492,
-0.990563629551857));
#43629=CARTESIAN_POINT('Ctrl Pts',(0.132349210999107,-0.0795266017162653,
-0.987914532449207));
#43630=CARTESIAN_POINT('Ctrl Pts',(0.151872139437857,-0.027850445152484,
-0.985265435346556));
#43631=CARTESIAN_POINT('Ctrl Pts',(0.145194901660481,0.0201836136139252,
-0.982616338243906));
#43632=CARTESIAN_POINT('Ctrl Pts',(0.138517663883105,0.0682176723803358,
-0.979967241141256));
#43633=CARTESIAN_POINT('Ctrl Pts',(0.105640259889603,0.112609633349376,
-0.977318144038606));
#43634=CARTESIAN_POINT('Ctrl Pts',(0.0616400217185707,0.133001674610688,
-0.974669046935955));
#43635=CARTESIAN_POINT('Ctrl Pts',(0.0176397835475385,0.153393715871999,
-0.972019949833305));
#43636=CARTESIAN_POINT('Ctrl Pts',(-0.037483288801022,0.149785837425582,
-0.969370852730653));
#43637=CARTESIAN_POINT('Ctrl Pts',(-0.0784501658468312,0.12383258539382,
-0.966721755628003));
#43638=CARTESIAN_POINT('Ctrl Pts',(-0.11941704289264,0.0978793333620585,
-0.964072658525352));
#43639=CARTESIAN_POINT('Ctrl Pts',(-0.146227724635697,0.0495807077449533,
-0.961423561422702));
#43640=CARTESIAN_POINT('Ctrl Pts',(-0.146587032572823,0.00108609769685721,
-0.958774464320051));
#43641=CARTESIAN_POINT('Ctrl Pts',(-0.146589698223321,0.000726323619918058,
-0.958754811074796));
#43642=CARTESIAN_POINT('Ctrl Pts',(-0.146590908009088,0.000366538756135779,
-0.958735157829541));
#43643=CARTESIAN_POINT('Ctrl Pts',(-0.146590666816024,6.75222312525112E-6,
-0.958715504584286));
#43644=CARTESIAN_POINT('Origin',(0.,0.,-1.487));
#43645=CARTESIAN_POINT('',(-0.146292875288708,0.000132171896627023,-0.901584495415713));
#43646=CARTESIAN_POINT('',(-0.14625608928872,0.000126173321545744,-0.908715504584286));
#43647=CARTESIAN_POINT('',(-0.14635,-1.79227059055215E-17,-1.487));
#43648=CARTESIAN_POINT('Ctrl Pts',(-0.146292875288708,0.000132171896627023,
-0.901584495415713));
#43649=CARTESIAN_POINT('Ctrl Pts',(-0.146409043898152,0.013395829194403,
-0.902305205774001));
#43650=CARTESIAN_POINT('Ctrl Pts',(-0.144754282125947,0.0266310140695942,
-0.90302591613229));
#43651=CARTESIAN_POINT('Ctrl Pts',(-0.141213464455431,0.0393407612670267,
-0.903746626490579));
#43652=CARTESIAN_POINT('Ctrl Pts',(-0.128198569187039,0.086057662292393,
-0.90639572359323));
#43653=CARTESIAN_POINT('Ctrl Pts',(-0.0897019510869531,0.125675591711476,
-0.909044820695881));
#43654=CARTESIAN_POINT('Ctrl Pts',(-0.0433778718351044,0.140026062844143,
-0.911693917798532));
#43655=CARTESIAN_POINT('Ctrl Pts',(0.00294620741674562,0.15437653397681,
-0.914343014901182));
#43656=CARTESIAN_POINT('Ctrl Pts',(0.0570977478203569,0.143459546823063,
-0.916992112003832));
#43657=CARTESIAN_POINT('Ctrl Pts',(0.0942432571928315,0.112281550195303,
-0.919641209106482));
#43658=CARTESIAN_POINT('Ctrl Pts',(0.131388766565305,0.0811035535675439,
-0.922290306209133));
#43659=CARTESIAN_POINT('Ctrl Pts',(0.15152824490664,0.0296645474657715,
-0.924939403311784));
#43660=CARTESIAN_POINT('Ctrl Pts',(0.145425877792544,-0.0184459239086174,
-0.927588500414435));
#43661=CARTESIAN_POINT('Ctrl Pts',(0.139323510678449,-0.0665563952830063,
-0.930237597517086));
#43662=CARTESIAN_POINT('Ctrl Pts',(0.106979298108923,-0.111338331930014,
-0.932886694619735));
#43663=CARTESIAN_POINT('Ctrl Pts',(0.0632260545158511,-0.132255072004567,
-0.935535791722385));
#43664=CARTESIAN_POINT('Ctrl Pts',(0.0194728109227757,-0.153171812079122,
-0.938184888825036));
#43665=CARTESIAN_POINT('Ctrl Pts',(-0.0356894636938444,-0.15022335558122,
-0.940833985927687));
#43666=CARTESIAN_POINT('Ctrl Pts',(-0.0769637619862466,-0.124761842650303,
-0.943483083030338));
#43667=CARTESIAN_POINT('Ctrl Pts',(-0.118238060278645,-0.0993003297193876,
-0.946132180132989));
#43668=CARTESIAN_POINT('Ctrl Pts',(-0.145624382246826,-0.0513257603554585,
-0.948781277235639));
#43669=CARTESIAN_POINT('Ctrl Pts',(-0.146563565077574,-0.00283891393427424,
-0.95143037433829));
#43670=CARTESIAN_POINT('Ctrl Pts',(-0.146581778562416,-0.00189861305417535,
-0.951481748030764));
#43671=CARTESIAN_POINT('Ctrl Pts',(-0.146590045679609,-0.000958119514449902,
-0.951533121723238));
#43672=CARTESIAN_POINT('Ctrl Pts',(-0.146588451745324,-1.75972019087617E-5,
-0.951584495415713));
#43673=CARTESIAN_POINT('Ctrl Pts',(-0.146590666816024,6.75222312525112E-6,
-0.958715504584286));
#43674=CARTESIAN_POINT('Ctrl Pts',(-0.146558397152076,-0.0481297502687534,
-0.956086060726891));
#43675=CARTESIAN_POINT('Ctrl Pts',(-0.120553234067385,-0.0962961323745566,
-0.953456616869495));
#43676=CARTESIAN_POINT('Ctrl Pts',(-0.0802764615941904,-0.122656542592026,
-0.9508271730121));
#43677=CARTESIAN_POINT('Ctrl Pts',(-0.0396986485472351,-0.149213978353728,
-0.948178075909449));
#43678=CARTESIAN_POINT('Ctrl Pts',(0.0153649116778716,-0.153638255398045,
-0.945528978806799));
#43679=CARTESIAN_POINT('Ctrl Pts',(0.059662481416401,-0.133900433300086,
-0.942879881704148));
#43680=CARTESIAN_POINT('Ctrl Pts',(0.10396005115493,-0.114162611202126,
-0.940230784601498));
#43681=CARTESIAN_POINT('Ctrl Pts',(0.137491630406883,-0.0702626899618913,
-0.937581687498847));
#43682=CARTESIAN_POINT('Ctrl Pts',(0.144879887243613,-0.0223328457432308,
-0.934932590396196));
#43683=CARTESIAN_POINT('Ctrl Pts',(0.152268144080344,0.0255969984754297,
-0.932283493293546));
#43684=CARTESIAN_POINT('Ctrl Pts',(0.133513078501854,0.0775567656725155,
-0.929634396190896));
#43685=CARTESIAN_POINT('Ctrl Pts',(0.0972156235741606,0.10971809449585,
-0.926985299088245));
#43686=CARTESIAN_POINT('Ctrl Pts',(0.0609181686464652,0.141879423319186,
-0.924336201985595));
#43687=CARTESIAN_POINT('Ctrl Pts',(0.00707832436956497,0.154242313768768,
-0.921687104882944));
#43688=CARTESIAN_POINT('Ctrl Pts',(-0.0396133585905054,0.141137236574524,
-0.919038007780294));
#43689=CARTESIAN_POINT('Ctrl Pts',(-0.0863050415505731,0.12803215938028,
-0.916388910677643));
#43690=CARTESIAN_POINT('Ctrl Pts',(-0.125848563193812,0.0894591145422132,
-0.913739813574992));
#43691=CARTESIAN_POINT('Ctrl Pts',(-0.140109559690632,0.043107412471758,
-0.911090716472341));
#43692=CARTESIAN_POINT('Ctrl Pts',(-0.144371752568961,0.0292542504920058,
-0.910298979176323));
#43693=CARTESIAN_POINT('Ctrl Pts',(-0.14637561806891,0.0147062704712071,
-0.909507241880305));
#43694=CARTESIAN_POINT('Ctrl Pts',(-0.14625608928872,0.000126173321545744,
-0.908715504584286));
#43695=CARTESIAN_POINT('Origin',(0.,0.,-1.487));
#43696=CARTESIAN_POINT('',(-0.146124565373613,-5.00382259003701E-5,-0.851584495415712));
#43697=CARTESIAN_POINT('',(-0.146140623441789,-6.94491364294977E-5,-0.858715504584287));
#43698=CARTESIAN_POINT('',(-0.14635,-1.79227059055215E-17,-1.487));
#43699=CARTESIAN_POINT('Ctrl Pts',(-0.146124565373613,-5.00382259003701E-5,
-0.851584495415712));
#43700=CARTESIAN_POINT('Ctrl Pts',(-0.146040186260976,0.0275024656860341,
-0.853077289824765));
#43701=CARTESIAN_POINT('Ctrl Pts',(-0.138564166815548,0.0550974423910985,
-0.854570084233817));
#43702=CARTESIAN_POINT('Ctrl Pts',(-0.123983835914978,0.0782109101876611,
-0.85606287864287));
#43703=CARTESIAN_POINT('Ctrl Pts',(-0.0981097355632086,0.119227824640698,
-0.858711975745521));
#43704=CARTESIAN_POINT('Ctrl Pts',(-0.0498629687339267,0.14613171705648,
-0.861361072848171));
#43705=CARTESIAN_POINT('Ctrl Pts',(-0.00136914252851839,0.146584663213145,
-0.864010169950822));
#43706=CARTESIAN_POINT('Ctrl Pts',(0.0471246836768899,0.14703760936981,
-0.866659267053472));
#43707=CARTESIAN_POINT('Ctrl Pts',(0.0958655692584217,0.121039609267357,
-0.869308364156122));
#43708=CARTESIAN_POINT('Ctrl Pts',(0.12250130794355,0.0805131516753259,
-0.871957461258773));
#43709=CARTESIAN_POINT('Ctrl Pts',(0.149137046628681,0.0399866940832921,
-0.874606558361424));
#43710=CARTESIAN_POINT('Ctrl Pts',(0.153667638417403,-0.0150682209983281,
-0.877255655464076));
#43711=CARTESIAN_POINT('Ctrl Pts',(0.134015387736689,-0.0594038205030583,
-0.879904752566726));
#43712=CARTESIAN_POINT('Ctrl Pts',(0.114363137055977,-0.103739420007784,
-0.882553849669376));
#43713=CARTESIAN_POINT('Ctrl Pts',(0.0705280439058388,-0.137355703935627,
-0.885202946772025));
#43714=CARTESIAN_POINT('Ctrl Pts',(0.0226125547719502,-0.144836495425912,
-0.887852043874676));
#43715=CARTESIAN_POINT('Ctrl Pts',(-0.0253029343619412,-0.152317286916197,
-0.890501140977326));
#43716=CARTESIAN_POINT('Ctrl Pts',(-0.0772988194795806,-0.13366258596892,
-0.893150238079978));
#43717=CARTESIAN_POINT('Ctrl Pts',(-0.109530175820052,-0.0974272991794556,
-0.895799335182629));
#43718=CARTESIAN_POINT('Ctrl Pts',(-0.132992705848706,-0.0710501434862831,
-0.897727721926991));
#43719=CARTESIAN_POINT('Ctrl Pts',(-0.145982045835535,-0.0353570653824267,
-0.899656108671351));
#43720=CARTESIAN_POINT('Ctrl Pts',(-0.146292875288708,0.000132171896627023,
-0.901584495415713));
#43721=CARTESIAN_POINT('Ctrl Pts',(-0.14625608928872,0.000126173321545744,
-0.908715504584286));
#43722=CARTESIAN_POINT('Ctrl Pts',(-0.145975683208097,-0.0340777053624083,
-0.906858144777654));
#43723=CARTESIAN_POINT('Ctrl Pts',(-0.134009421342487,-0.0684583369648513,
-0.905000784971022));
#43724=CARTESIAN_POINT('Ctrl Pts',(-0.112099364503826,-0.0944598867485631,
-0.90314342516439));
#43725=CARTESIAN_POINT('Ctrl Pts',(-0.0808497014697991,-0.131545124595585,
-0.90049432806174));
#43726=CARTESIAN_POINT('Ctrl Pts',(-0.0293719040513464,-0.151585240986786,
-0.897845230959089));
#43727=CARTESIAN_POINT('Ctrl Pts',(0.0187266941418953,-0.145389988146464,
-0.895196133856439));
#43728=CARTESIAN_POINT('Ctrl Pts',(0.0668252923351411,-0.139194735306142,
-0.892547036753788));
#43729=CARTESIAN_POINT('Ctrl Pts',(0.111544691303172,-0.106764113234289,
-0.889897939651137));
#43730=CARTESIAN_POINT('Ctrl Pts',(0.132376908513643,-0.0629705631155036,
-0.887248842548487));
#43731=CARTESIAN_POINT('Ctrl Pts',(0.153209125724114,-0.0191770129967208,
-0.884599745445836));
#43732=CARTESIAN_POINT('Ctrl Pts',(0.150154161177028,0.0359794651689932,
-0.881950648343186));
#43733=CARTESIAN_POINT('Ctrl Pts',(0.12461299880809,0.0772045222429877,
-0.879301551240535));
#43734=CARTESIAN_POINT('Ctrl Pts',(0.0990718364391528,0.118429579316982,
-0.876652454137885));
#43735=CARTESIAN_POINT('Ctrl Pts',(0.0510444762483626,0.145723215299258,
-0.874003357035234));
#43736=CARTESIAN_POINT('Ctrl Pts',(0.00255590709058795,0.146568772477828,
-0.871354259932583));
#43737=CARTESIAN_POINT('Ctrl Pts',(-0.0459326620671895,0.147414329656398,
-0.868705162829933));
#43738=CARTESIAN_POINT('Ctrl Pts',(-0.094882440191953,0.121811808031259,
-0.866056065727283));
#43739=CARTESIAN_POINT('Ctrl Pts',(-0.121845424450247,0.0815023328945396,
-0.863406968624632));
#43740=CARTESIAN_POINT('Ctrl Pts',(-0.137762277899623,0.0577067469821571,
-0.86184314727785));
#43741=CARTESIAN_POINT('Ctrl Pts',(-0.146017161763102,0.0287860741111531,
-0.860279325931069));
#43742=CARTESIAN_POINT('Ctrl Pts',(-0.146140623441789,-6.94491364294977E-5,
-0.858715504584287));
#43743=CARTESIAN_POINT('Origin',(0.,0.,-1.487));
#43744=CARTESIAN_POINT('',(-0.146476704385463,-0.000110408673293372,-0.801584495415713));
#43745=CARTESIAN_POINT('',(-0.146510711569069,-9.54240844848774E-5,-0.808715504584287));
#43746=CARTESIAN_POINT('',(-0.14635,-1.79227059055215E-17,-1.487));
#43747=CARTESIAN_POINT('Ctrl Pts',(-0.146476704385463,-0.000110408673293372,
-0.801584495415713));
#43748=CARTESIAN_POINT('Ctrl Pts',(-0.146128043182839,0.0414372295960993,
-0.803849373875529));
#43749=CARTESIAN_POINT('Ctrl Pts',(-0.127578682884935,0.0832570258228007,
-0.806114252335345));
#43750=CARTESIAN_POINT('Ctrl Pts',(-0.0963241152735199,0.11050159662805,
-0.808379130795161));
#43751=CARTESIAN_POINT('Ctrl Pts',(-0.0597674584934802,0.142367992491521,
-0.811028227897811));
#43752=CARTESIAN_POINT('Ctrl Pts',(-0.00582928347880528,0.154294568390982,
-0.813677325000461));
#43753=CARTESIAN_POINT('Ctrl Pts',(0.0407547653621746,0.140811885651917,
-0.816326422103112));
#43754=CARTESIAN_POINT('Ctrl Pts',(0.0873388142031571,0.127329202912852,
-0.818975519205763));
#43755=CARTESIAN_POINT('Ctrl Pts',(0.126568736870447,0.0884372615352578,
-0.821624616308414));
#43756=CARTESIAN_POINT('Ctrl Pts',(0.140453983683775,0.0419716155030087,
-0.824273713411064));
#43757=CARTESIAN_POINT('Ctrl Pts',(0.154339230497103,-0.00449403052923781,
-0.826922810513715));
#43758=CARTESIAN_POINT('Ctrl Pts',(0.142879801456478,-0.0585333812161332,
-0.829571907616364));
#43759=CARTESIAN_POINT('Ctrl Pts',(0.111330905174243,-0.0953643937413661,
-0.832221004719015));
#43760=CARTESIAN_POINT('Ctrl Pts',(0.0797820088920082,-0.132195406266599,
-0.834870101821665));
#43761=CARTESIAN_POINT('Ctrl Pts',(0.0281436453681626,-0.151818080630163,
-0.837519198924316));
#43762=CARTESIAN_POINT('Ctrl Pts',(-0.0199032173703552,-0.145233604853983,
-0.840168296026967));
#43763=CARTESIAN_POINT('Ctrl Pts',(-0.0679500801088757,-0.138649129077803,
-0.842817393129618));
#43764=CARTESIAN_POINT('Ctrl Pts',(-0.112405442062071,-0.105857503161875,
-0.845466490232268));
#43765=CARTESIAN_POINT('Ctrl Pts',(-0.132882406101538,-0.0618967219587649,
-0.848115587334919));
#43766=CARTESIAN_POINT('Ctrl Pts',(-0.141820382988776,-0.0427083087945367,
-0.849271890028517));
#43767=CARTESIAN_POINT('Ctrl Pts',(-0.146189924538032,-0.0213919151082998,
-0.850428192722114));
#43768=CARTESIAN_POINT('Ctrl Pts',(-0.146124565373613,-5.00382259003701E-5,
-0.851584495415712));
#43769=CARTESIAN_POINT('Ctrl Pts',(-0.146140623441789,-6.94491364294977E-5,
-0.858715504584287));
#43770=CARTESIAN_POINT('Ctrl Pts',(-0.146226304563187,-0.0200948822640432,
-0.857630228828418));
#43771=CARTESIAN_POINT('Ctrl Pts',(-0.142395717371333,-0.0400889379277852,
-0.856544953072549));
#43772=CARTESIAN_POINT('Ctrl Pts',(-0.134491951859747,-0.0583168295749055,
-0.85545967731668));
#43773=CARTESIAN_POINT('Ctrl Pts',(-0.11519930461913,-0.102810088259337,
-0.85281058021403));
#43774=CARTESIAN_POINT('Ctrl Pts',(-0.0716378197460715,-0.136780176979901,
-0.85016148311138));
#43775=CARTESIAN_POINT('Ctrl Pts',(-0.0237844690128919,-0.144648666639164,
-0.847512386008729));
#43776=CARTESIAN_POINT('Ctrl Pts',(0.0240688817202849,-0.152517156298425,
-0.844863288906079));
#43777=CARTESIAN_POINT('Ctrl Pts',(0.0762140983135795,-0.134284046896388,
-0.842214191803427));
#43778=CARTESIAN_POINT('Ctrl Pts',(0.108737773706116,-0.0983109062929979,
-0.839565094700777));
#43779=CARTESIAN_POINT('Ctrl Pts',(0.141261449098654,-0.0623377656896056,
-0.836915997598127));
#43780=CARTESIAN_POINT('Ctrl Pts',(0.154163583290429,-0.00862459388485129,
-0.834266900495477));
#43781=CARTESIAN_POINT('Ctrl Pts',(0.141527353856701,0.0381961495053259,
-0.831617803392826));
#43782=CARTESIAN_POINT('Ctrl Pts',(0.128891124422972,0.0850168928955057,
-0.828968706290175));
#43783=CARTESIAN_POINT('Ctrl Pts',(0.0907165313637413,0.124945207871112,
-0.826319609187524));
#43784=CARTESIAN_POINT('Ctrl Pts',(0.0445101580791478,0.139670267252849,
-0.823670512084873));
#43785=CARTESIAN_POINT('Ctrl Pts',(-0.00169621520544052,0.154395326634585,
-0.821021414982223));
#43786=CARTESIAN_POINT('Ctrl Pts',(-0.0559343687153863,0.143917130422458,
-0.818372317879574));
#43787=CARTESIAN_POINT('Ctrl Pts',(-0.0933310901438021,0.113040901178656,
-0.815723220776923));
#43788=CARTESIAN_POINT('Ctrl Pts',(-0.126306553122389,0.0858150397807172,
-0.813387315379378));
#43789=CARTESIAN_POINT('Ctrl Pts',(-0.14618737006938,0.0427291837577693,
-0.811051409981832));
#43790=CARTESIAN_POINT('Ctrl Pts',(-0.146510711569069,-9.54240844848774E-5,
-0.808715504584287));
#43791=CARTESIAN_POINT('Origin',(0.,0.,-1.487));
#43792=CARTESIAN_POINT('',(-0.146474864373602,0.000111087822697115,-0.751584495415713));
#43793=CARTESIAN_POINT('',(-0.146437634202152,0.000122457214444137,-0.758715504584287));
#43794=CARTESIAN_POINT('',(-0.14635,-1.79227059055215E-17,-1.487));
#43795=CARTESIAN_POINT('Ctrl Pts',(-0.146474864373602,0.000111087822697115,
-0.751584495415713));
#43796=CARTESIAN_POINT('Ctrl Pts',(-0.146534826115463,0.0072264447354974,
-0.751972360823642));
#43797=CARTESIAN_POINT('Ctrl Pts',(-0.146061280249954,0.0143337876220666,
-0.752360226231571));
#43798=CARTESIAN_POINT('Ctrl Pts',(-0.145026728944115,0.0213585096002675,
-0.7527480916395));
#43799=CARTESIAN_POINT('Ctrl Pts',(-0.137960806562755,0.0693369326794158,
-0.75539718874215));
#43800=CARTESIAN_POINT('Ctrl Pts',(-0.104725064437985,0.113461250034078,
-0.7580462858448));
#43801=CARTESIAN_POINT('Ctrl Pts',(-0.0605611658003746,0.133496379117466,
-0.76069538294745));
#43802=CARTESIAN_POINT('Ctrl Pts',(-0.0163972671627661,0.153531508200852,
-0.763344480050101));
#43803=CARTESIAN_POINT('Ctrl Pts',(0.0386947879876798,0.149477449012966,
-0.765993577152752));
#43804=CARTESIAN_POINT('Ctrl Pts',(0.0794501944261966,0.12319336283345,
-0.768642674255402));
#43805=CARTESIAN_POINT('Ctrl Pts',(0.120205600864716,0.0969092766539328,
-0.771291771358053));
#43806=CARTESIAN_POINT('Ctrl Pts',(0.146624358591304,0.0483951634827755,
-0.773940868460703));
#43807=CARTESIAN_POINT('Ctrl Pts',(0.146591022530981,-0.000100766542003826,
-0.776589965563353));
#43808=CARTESIAN_POINT('Ctrl Pts',(0.146557686470658,-0.0485966965667832,
-0.779239062666004));
#43809=CARTESIAN_POINT('Ctrl Pts',(0.12007225662343,-0.0970744434451872,
-0.781888159768655));
#43810=CARTESIAN_POINT('Ctrl Pts',(0.079280753401082,-0.12330247434959,
-0.784537256871306));
#43811=CARTESIAN_POINT('Ctrl Pts',(0.0384892501787335,-0.149530505253994,
-0.787186353973957));
#43812=CARTESIAN_POINT('Ctrl Pts',(-0.0166083264187326,-0.153508820184394,
-0.789835451076606));
#43813=CARTESIAN_POINT('Ctrl Pts',(-0.0607446390721617,-0.133412993612194,
-0.792484548179257));
#43814=CARTESIAN_POINT('Ctrl Pts',(-0.104880951725593,-0.113317167039993,
-0.795133645281907));
#43815=CARTESIAN_POINT('Ctrl Pts',(-0.138056000434984,-0.0691471989651908,
-0.797782742384558));
#43816=CARTESIAN_POINT('Ctrl Pts',(-0.145055955516975,-0.021159107014046,
-0.800431839487209));
#43817=CARTESIAN_POINT('Ctrl Pts',(-0.146071212088286,-0.0141990301096382,
-0.800816058130044));
#43818=CARTESIAN_POINT('Ctrl Pts',(-0.146535851989388,-0.00715863553052973,
-0.801200276772879));
#43819=CARTESIAN_POINT('Ctrl Pts',(-0.146476704385463,-0.000110408673293372,
-0.801584495415713));
#43820=CARTESIAN_POINT('Ctrl Pts',(-0.146510711569069,-9.54240844848774E-5,
-0.808715504584287));
#43821=CARTESIAN_POINT('Ctrl Pts',(-0.146554064298903,-0.00583722851058804,
-0.808402312879181));
#43822=CARTESIAN_POINT('Ctrl Pts',(-0.146245838134586,-0.0115743365561838,
-0.808089121174076));
#43823=CARTESIAN_POINT('Ctrl Pts',(-0.145570455937086,-0.0172678917352987,
-0.807775929468971));
#43824=CARTESIAN_POINT('Ctrl Pts',(-0.139857810955068,-0.0654261931299693,
-0.80512683236632));
#43825=CARTESIAN_POINT('Ctrl Pts',(-0.107877231644147,-0.110468533643833,
-0.80247773526367));
#43826=CARTESIAN_POINT('Ctrl Pts',(-0.0642947729383683,-0.131738832162414,
-0.799828638161019));
#43827=CARTESIAN_POINT('Ctrl Pts',(-0.0207123142325892,-0.153009130680996,
-0.797179541058369));
#43828=CARTESIAN_POINT('Ctrl Pts',(0.0344720238680508,-0.150507387204297,
-0.794530443955718));
#43829=CARTESIAN_POINT('Ctrl Pts',(0.0759511158667185,-0.125380882614988,
-0.791881346853068));
#43830=CARTESIAN_POINT('Ctrl Pts',(0.117430207865391,-0.100254378025676,
-0.789232249750417));
#43831=CARTESIAN_POINT('Ctrl Pts',(0.145204053762091,-0.0525031123237477,
-0.786583152647766));
#43832=CARTESIAN_POINT('Ctrl Pts',(0.146535775162883,-0.00402545949255462,
-0.783934055545115));
#43833=CARTESIAN_POINT('Ctrl Pts',(0.147867496563675,0.0444521933386329,
-0.781284958442465));
#43834=CARTESIAN_POINT('Ctrl Pts',(0.122757093468571,0.0936562332990816,
-0.778635861339814));
#43835=CARTESIAN_POINT('Ctrl Pts',(0.0827200092855296,0.121022054975591,
-0.775986764237164));
#43836=CARTESIAN_POINT('Ctrl Pts',(0.0426829251024876,0.148387876652101,
-0.773337667134513));
#43837=CARTESIAN_POINT('Ctrl Pts',(-0.012280840168493,0.153915480044665,
-0.770688570031864));
#43838=CARTESIAN_POINT('Ctrl Pts',(-0.0569653140836648,0.135069947501517,
-0.768039472929213));
#43839=CARTESIAN_POINT('Ctrl Pts',(-0.101649787998837,0.116224414958369,
-0.765390375826563));
#43840=CARTESIAN_POINT('Ctrl Pts',(-0.136054970558202,0.0730057464795088,
-0.762741278723911));
#43841=CARTESIAN_POINT('Ctrl Pts',(-0.144402901877865,0.0252337007980361,
-0.760092181621261));
#43842=CARTESIAN_POINT('Ctrl Pts',(-0.145848980158966,0.0169583431006113,
-0.759633289275603));
#43843=CARTESIAN_POINT('Ctrl Pts',(-0.146513152571914,0.00854635117719349,
-0.759174396929945));
#43844=CARTESIAN_POINT('Ctrl Pts',(-0.146437634202152,0.000122457214444137,
-0.758715504584287));
#43845=CARTESIAN_POINT('Origin',(0.,0.,-1.487));
#43846=CARTESIAN_POINT('',(-0.146123885372185,4.90033357487263E-5,-0.701584495415714));
#43847=CARTESIAN_POINT('',(-0.146113547113789,2.8286021952426E-5,-0.708715504584287));
#43848=CARTESIAN_POINT('',(-0.14635,-1.79227059055215E-17,-1.487));
#43849=CARTESIAN_POINT('Ctrl Pts',(-0.146123885372185,4.90033357487263E-5,
-0.701584495415714));
#43850=CARTESIAN_POINT('Ctrl Pts',(-0.14618807769588,0.0214584373064795,
-0.702744444874405));
#43851=CARTESIAN_POINT('Ctrl Pts',(-0.141789805581938,0.0428427648591023,
-0.703904394333097));
#43852=CARTESIAN_POINT('Ctrl Pts',(-0.132797185057065,0.0620793498797645,
-0.705064343791789));
#43853=CARTESIAN_POINT('Ctrl Pts',(-0.112259803191701,0.106011937857001,
-0.70771344089444));
#43854=CARTESIAN_POINT('Ctrl Pts',(-0.0677594014011252,0.138742415657928,
-0.71036253799709));
#43855=CARTESIAN_POINT('Ctrl Pts',(-0.0197035317469352,0.145260830499044,
-0.713011635099741));
#43856=CARTESIAN_POINT('Ctrl Pts',(0.0283523379072549,0.151779245340161,
-0.715660732202392));
#43857=CARTESIAN_POINT('Ctrl Pts',(0.0799636754250591,0.132085597221468,
-0.718309829305043));
#43858=CARTESIAN_POINT('Ctrl Pts',(0.111461906704158,0.095211246155316,
-0.720958926407693));
#43859=CARTESIAN_POINT('Ctrl Pts',(0.142960137983255,0.0583368950891666,
-0.723608023510343));
#43860=CARTESIAN_POINT('Ctrl Pts',(0.154345263023649,0.0042818410755612,
-0.726257120612994));
#43861=CARTESIAN_POINT('Ctrl Pts',(0.140396148472813,-0.0421646716407751,
-0.728906217715644));
#43862=CARTESIAN_POINT('Ctrl Pts',(0.126447033921977,-0.0886111843571114,
-0.731555314818295));
#43863=CARTESIAN_POINT('Ctrl Pts',(0.0871636797799121,-0.127449155776179,
-0.734204411920946));
#43864=CARTESIAN_POINT('Ctrl Pts',(0.0405611390023424,-0.140867782134196,
-0.736853509023596));
#43865=CARTESIAN_POINT('Ctrl Pts',(-0.00604140177522741,-0.154286408492213,
-0.739502606126247));
#43866=CARTESIAN_POINT('Ctrl Pts',(-0.0599631291883016,-0.14228568978918,
-0.742151703228897));
#43867=CARTESIAN_POINT('Ctrl Pts',(-0.0964759415758636,-0.110369066035847,
-0.744800800331547));
#43868=CARTESIAN_POINT('Ctrl Pts',(-0.127642760093604,-0.0831254889139159,
-0.747062032026269));
#43869=CARTESIAN_POINT('Ctrl Pts',(-0.146125291072154,-0.0413710094243759,
-0.749323263720991));
#43870=CARTESIAN_POINT('Ctrl Pts',(-0.146474864373602,0.000111087822697115,
-0.751584495415713));
#43871=CARTESIAN_POINT('Ctrl Pts',(-0.146437634202152,0.000122457214444137,
-0.758715504584287));
#43872=CARTESIAN_POINT('Ctrl Pts',(-0.146077199572424,-0.0400831657474447,
-0.756525299827295));
#43873=CARTESIAN_POINT('Ctrl Pts',(-0.128866838266126,-0.0805599134748815,
-0.754335095070302));
#43874=CARTESIAN_POINT('Ctrl Pts',(-0.0993963040313856,-0.107746519533642,
-0.75214489031331));
#43875=CARTESIAN_POINT('Ctrl Pts',(-0.0637510947852846,-0.140629271299759,
-0.74949579321066));
#43876=CARTESIAN_POINT('Ctrl Pts',(-0.0101699962131163,-0.154069351947909,
-0.746846696108008));
#43877=CARTESIAN_POINT('Ctrl Pts',(0.036775099867708,-0.141903240824279,
-0.744197599005358));
#43878=CARTESIAN_POINT('Ctrl Pts',(0.0837201959485351,-0.129737129700647,
-0.741548501902707));
#43879=CARTESIAN_POINT('Ctrl Pts',(0.124029289538022,-0.0919648268052367,
-0.738899404800057));
#43880=CARTESIAN_POINT('Ctrl Pts',(0.139216931227097,-0.0459084282721892,
-0.736250307697407));
#43881=CARTESIAN_POINT('Ctrl Pts',(0.154404572916172,0.000147970260858429,
-0.733601210594756));
#43882=CARTESIAN_POINT('Ctrl Pts',(0.144470762704835,0.054488464431539,
-0.730952113492105));
#43883=CARTESIAN_POINT('Ctrl Pts',(0.113971071799202,0.0921929092699334,
-0.728303016389454));
#43884=CARTESIAN_POINT('Ctrl Pts',(0.0834713808935699,0.129897354108328,
-0.725653919286804));
#43885=CARTESIAN_POINT('Ctrl Pts',(0.0324058092936452,0.150965749614433,
-0.723004822184153));
#43886=CARTESIAN_POINT('Ctrl Pts',(-0.0158073530740039,0.145736286886646,
-0.720355725081503));
#43887=CARTESIAN_POINT('Ctrl Pts',(-0.0640205154416559,0.140506824158859,
-0.717706627978853));
#43888=CARTESIAN_POINT('Ctrl Pts',(-0.109381268577035,0.108979503197173,
-0.715057530876202));
#43889=CARTESIAN_POINT('Ctrl Pts',(-0.13108750971441,0.0656125180402923,
-0.712408433773551));
#43890=CARTESIAN_POINT('Ctrl Pts',(-0.141173916312492,0.0454608463410335,
-0.71117745737713));
#43891=CARTESIAN_POINT('Ctrl Pts',(-0.146152713380701,0.0227526906323401,
-0.709946480980708));
#43892=CARTESIAN_POINT('Ctrl Pts',(-0.146113547113789,2.8286021952426E-5,
-0.708715504584287));
#43893=CARTESIAN_POINT('Origin',(0.,0.,-1.487));
#43894=CARTESIAN_POINT('',(-0.146294822930562,-0.000132384695170809,-0.651584495415713));
#43895=CARTESIAN_POINT('',(-0.146333590452415,-0.000134607837447892,-0.658715504584287));
#43896=CARTESIAN_POINT('',(-0.14635,-1.79227059055215E-17,-1.487));
#43897=CARTESIAN_POINT('Ctrl Pts',(-0.146294822930562,-0.000132384695170809,
-0.651584495415713));
#43898=CARTESIAN_POINT('Ctrl Pts',(-0.145982575394241,0.0354227639412815,
-0.653516528925169));
#43899=CARTESIAN_POINT('Ctrl Pts',(-0.132939339037653,0.0711830937012871,
-0.655448562434624));
#43900=CARTESIAN_POINT('Ctrl Pts',(-0.109396129491268,0.0975777889322379,
-0.65738059594408));
#43901=CARTESIAN_POINT('Ctrl Pts',(-0.077114987424532,0.133768729886137,
-0.660029693046731));
#43902=CARTESIAN_POINT('Ctrl Pts',(-0.0250935050063507,0.152351929385001,
-0.662678790149382));
#43903=CARTESIAN_POINT('Ctrl Pts',(0.0228116542714107,0.14480527086393,
-0.665327887252032));
#43904=CARTESIAN_POINT('Ctrl Pts',(0.0707168135491666,0.137258612342861,
-0.667976984354682));
#43905=CARTESIAN_POINT('Ctrl Pts',(0.114505649686507,0.103582095801863,
-0.670626081457333));
#43906=CARTESIAN_POINT('Ctrl Pts',(0.134096929318507,0.0592195203283678,
-0.673275178559983));
#43907=CARTESIAN_POINT('Ctrl Pts',(0.153688208950508,0.01485694485487,-0.675924275662634));
#43908=CARTESIAN_POINT('Ctrl Pts',(0.14908193207717,-0.0401916895511217,
-0.678573372765284));
#43909=CARTESIAN_POINT('Ctrl Pts',(0.122390502886327,-0.0806814900941138,
-0.681222469867935));
#43910=CARTESIAN_POINT('Ctrl Pts',(0.0956990736954827,-0.121171290637108,
-0.683871566970585));
#43911=CARTESIAN_POINT('Ctrl Pts',(0.0469224921871279,-0.147102257317095,
-0.686520664073236));
#43912=CARTESIAN_POINT('Ctrl Pts',(-0.00157066548063597,-0.146582642391664,
-0.689169761175886));
#43913=CARTESIAN_POINT('Ctrl Pts',(-0.0500638231483971,-0.146063027466233,
-0.691818858278537));
#43914=CARTESIAN_POINT('Ctrl Pts',(-0.0982735569755703,-0.119092830935388,
-0.694467955381187));
#43915=CARTESIAN_POINT('Ctrl Pts',(-0.124091242919077,-0.0780403835931955,
-0.697117052483838));
#43916=CARTESIAN_POINT('Ctrl Pts',(-0.138604242898114,-0.0549634057137551,
-0.698606200127797));
#43917=CARTESIAN_POINT('Ctrl Pts',(-0.146041475016394,-0.0274365115865579,
-0.700095347771755));
#43918=CARTESIAN_POINT('Ctrl Pts',(-0.146123885372185,4.90033357487263E-5,
-0.701584495415714));
#43919=CARTESIAN_POINT('Ctrl Pts',(-0.146113547113789,2.8286021952426E-5,
-0.708715504584287));
#43920=CARTESIAN_POINT('Ctrl Pts',(-0.146068426432147,-0.0261508907749407,
-0.707297383878057));
#43921=CARTESIAN_POINT('Ctrl Pts',(-0.139363609380872,-0.0523516326460269,
-0.705879263171828));
#43922=CARTESIAN_POINT('Ctrl Pts',(-0.126136159605208,-0.0746900727457313,
-0.704461142465599));
#43923=CARTESIAN_POINT('Ctrl Pts',(-0.101426839219253,-0.116419029022818,
-0.701812045362949));
#43924=CARTESIAN_POINT('Ctrl Pts',(-0.0539564693079595,-0.144670292224918,
-0.699162948260299));
#43925=CARTESIAN_POINT('Ctrl Pts',(-0.00549460714200485,-0.146488043945805,
-0.696513851157648));
#43926=CARTESIAN_POINT('Ctrl Pts',(0.0429672550239443,-0.148305795666692,
-0.693864754054998));
#43927=CARTESIAN_POINT('Ctrl Pts',(0.0924206094445576,-0.123690035906373,
-0.691215656952347));
#43928=CARTESIAN_POINT('Ctrl Pts',(0.120186516956348,-0.0839293683320362,
-0.688566559849696));
#43929=CARTESIAN_POINT('Ctrl Pts',(0.14795242446814,-0.044168700757697,
-0.685917462747046));
#43930=CARTESIAN_POINT('Ctrl Pts',(0.154030885071109,0.0107368746306564,
-0.683268365644396));
#43931=CARTESIAN_POINT('Ctrl Pts',(0.135634362108998,0.0556080708350706,
-0.680619268541746));
#43932=CARTESIAN_POINT('Ctrl Pts',(0.117237839146887,0.100479267039487,
-0.677970171439095));
#43933=CARTESIAN_POINT('Ctrl Pts',(0.0743663326196887,0.135316084059958,
-0.675321074336444));
#43934=CARTESIAN_POINT('Ctrl Pts',(0.0266803953810701,0.144142617670912,
-0.672671977233793));
#43935=CARTESIAN_POINT('Ctrl Pts',(-0.0210055418575457,0.152969151281866,
-0.670022880131143));
#43936=CARTESIAN_POINT('Ctrl Pts',(-0.0735059098075844,0.135785401483307,
-0.667373783028492));
#43937=CARTESIAN_POINT('Ctrl Pts',(-0.106744431647197,0.100471707654593,
-0.664724685925842));
#43938=CARTESIAN_POINT('Ctrl Pts',(-0.131877058289386,0.0737699822699243,
-0.662721625478657));
#43939=CARTESIAN_POINT('Ctrl Pts',(-0.14599707480881,0.0367027911865322,
-0.660718565031472));
#43940=CARTESIAN_POINT('Ctrl Pts',(-0.146333590452415,-0.000134607837447892,
-0.658715504584287));
#43941=CARTESIAN_POINT('Origin',(0.,0.,-1.487));
#43942=CARTESIAN_POINT('',(-0.146588075907495,1.88366579988541E-5,-0.601584495415713));
#43943=CARTESIAN_POINT('',(-0.146576141592014,4.24426192752484E-5,-0.608715504584288));
#43944=CARTESIAN_POINT('',(-0.14635,-1.79227059055215E-17,-1.487));
#43945=CARTESIAN_POINT('Ctrl Pts',(-0.146588075907495,1.88366579988541E-5,
-0.601584495415713));
#43946=CARTESIAN_POINT('Ctrl Pts',(-0.146589897057712,0.00102612895765277,
-0.601639515873282));
#43947=CARTESIAN_POINT('Ctrl Pts',(-0.146580414477156,0.00203338605800054,
-0.60169453633085));
#43948=CARTESIAN_POINT('Ctrl Pts',(-0.146559523637802,0.00304040649174867,
-0.601749556788419));
#43949=CARTESIAN_POINT('Ctrl Pts',(-0.145553682093586,0.051525915904862,
-0.604398653891069));
#43950=CARTESIAN_POINT('Ctrl Pts',(-0.118101430682682,0.0994627892809135,
-0.60704775099372));
#43951=CARTESIAN_POINT('Ctrl Pts',(-0.0767921669685648,0.124867534342785,
-0.60969684809637));
#43952=CARTESIAN_POINT('Ctrl Pts',(-0.0354829032544475,0.150272279404657,
-0.612345945199021));
#43953=CARTESIAN_POINT('Ctrl Pts',(0.01968337276288,0.153144896152347,-0.614995042301671));
#43954=CARTESIAN_POINT('Ctrl Pts',(0.0634078187231624,0.132168023989712,
-0.617644139404322));
#43955=CARTESIAN_POINT('Ctrl Pts',(0.107132264683442,0.111191151827078,
-0.620293236506972));
#43956=CARTESIAN_POINT('Ctrl Pts',(0.139414880586675,0.066364790754123,
-0.622942333609623));
#43957=CARTESIAN_POINT('Ctrl Pts',(0.145451099772318,0.0182459753260203,
-0.625591430712273));
#43958=CARTESIAN_POINT('Ctrl Pts',(0.151487318957961,-0.0298728401020852,
-0.628240527814924));
#43959=CARTESIAN_POINT('Ctrl Pts',(0.131277141426005,-0.0812841098853423,
-0.630889624917574));
#43960=CARTESIAN_POINT('Ctrl Pts',(0.0940888037217889,-0.112411009490962,
-0.633538722020225));
#43961=CARTESIAN_POINT('Ctrl Pts',(0.0569004660175705,-0.143537909096584,
-0.636187819122875));
#43962=CARTESIAN_POINT('Ctrl Pts',(0.00273396814109076,-0.154380438524573,
-0.638836916225527));
#43963=CARTESIAN_POINT('Ctrl Pts',(-0.0435703383393503,-0.139966294719726,
-0.641486013328177));
#43964=CARTESIAN_POINT('Ctrl Pts',(-0.0898746448197888,-0.125552150914879,
-0.644135110430828));
#43965=CARTESIAN_POINT('Ctrl Pts',(-0.128316759904187,-0.0858813338771997,
-0.646784207533478));
#43966=CARTESIAN_POINT('Ctrl Pts',(-0.14126741658874,-0.0391465841538942,
-0.649433304636128));
#43967=CARTESIAN_POINT('Ctrl Pts',(-0.144772929620772,-0.026496316434326,
-0.650150368229323));
#43968=CARTESIAN_POINT('Ctrl Pts',(-0.146410711883453,-0.0133284822333657,
-0.650867431822518));
#43969=CARTESIAN_POINT('Ctrl Pts',(-0.146294822930562,-0.000132384695170809,
-0.651584495415713));
#43970=CARTESIAN_POINT('Ctrl Pts',(-0.146333590452415,-0.000134607837447892,
-0.658715504584287));
#43971=CARTESIAN_POINT('Ctrl Pts',(-0.146442125090604,-0.0120155823207427,
-0.658069467928821));
#43972=CARTESIAN_POINT('Ctrl Pts',(-0.145116869066501,-0.0238726533188477,
-0.657423431273356));
#43973=CARTESIAN_POINT('Ctrl Pts',(-0.142264859682514,-0.0353503525615738,
-0.65677739461789));
#43974=CARTESIAN_POINT('Ctrl Pts',(-0.130570090149032,-0.0824150810901572,
-0.65412829751524));
#43975=CARTESIAN_POINT('Ctrl Pts',(-0.0932038753528797,-0.123100900288456,
-0.651479200412589));
#43976=CARTESIAN_POINT('Ctrl Pts',(-0.047302082457368,-0.138749597195485,
-0.648830103309939));
#43977=CARTESIAN_POINT('Ctrl Pts',(-0.00140028956185621,-0.154398294102514,
-0.646181006207288));
#43978=CARTESIAN_POINT('Ctrl Pts',(0.0530370814330175,-0.145009868718274,
-0.643531909104638));
#43979=CARTESIAN_POINT('Ctrl Pts',(0.0910454585689465,-0.114889782838525,
-0.640882812001987));
#43980=CARTESIAN_POINT('Ctrl Pts',(0.129053835704878,-0.0847696969587736,
-0.638233714899337));
#43981=CARTESIAN_POINT('Ctrl Pts',(0.150633218981865,-0.0339179505835095,
-0.635584617796686));
#43982=CARTESIAN_POINT('Ctrl Pts',(0.145887464321147,0.0143452250124984,
-0.632935520694035));
#43983=CARTESIAN_POINT('Ctrl Pts',(0.141141709660429,0.0626084006085036,
-0.630286423591385));
#43984=CARTESIAN_POINT('Ctrl Pts',(0.110070817062014,0.108283005425247,
-0.627637326488734));
#43985=CARTESIAN_POINT('Ctrl Pts',(0.0669236659244788,0.130423006658878,
-0.624988229386084));
#43986=CARTESIAN_POINT('Ctrl Pts',(0.0237765147869411,0.152563007892511,
-0.622339132283433));
#43987=CARTESIAN_POINT('Ctrl Pts',(-0.0314468948897182,0.15116840554302,
-0.619690035180783));
#43988=CARTESIAN_POINT('Ctrl Pts',(-0.0734215196755741,0.126878753837049,
-0.617040938078132));
#43989=CARTESIAN_POINT('Ctrl Pts',(-0.115396144461428,0.102589102131079,
-0.614391840975482));
#43990=CARTESIAN_POINT('Ctrl Pts',(-0.144121984356482,0.0554044010686303,
-0.611742743872831));
#43991=CARTESIAN_POINT('Ctrl Pts',(-0.146425583625881,0.00696320231884148,
-0.609093646770181));
#43992=CARTESIAN_POINT('Ctrl Pts',(-0.146535191796691,0.00465830873023068,
-0.608967599374883));
#43993=CARTESIAN_POINT('Ctrl Pts',(-0.146584980624434,0.00235057045985025,
-0.608841551979585));
#43994=CARTESIAN_POINT('Ctrl Pts',(-0.146576141592014,4.24426192752484E-5,
-0.608715504584288));
#43995=CARTESIAN_POINT('Origin',(0.,0.,-1.487));
#43996=CARTESIAN_POINT('',(-0.146238745768959,0.000121916852571603,-0.551584495415713));
#43997=CARTESIAN_POINT('',(-0.146206336570823,0.000110995926028272,-0.558715504584287));
#43998=CARTESIAN_POINT('',(-0.14635,-1.79227059055215E-17,-1.487));
#43999=CARTESIAN_POINT('Ctrl Pts',(-0.146238745768959,0.000121916852571603,
-0.551584495415713));
#44000=CARTESIAN_POINT('Ctrl Pts',(-0.146358386267051,0.0153578781833637,
-0.552411599924045));
#44001=CARTESIAN_POINT('Ctrl Pts',(-0.14416750967714,0.0305602873884727,
-0.553238704432377));
#44002=CARTESIAN_POINT('Ctrl Pts',(-0.139522367613658,0.0449716241207044,
-0.554065808940709));
#44003=CARTESIAN_POINT('Ctrl Pts',(-0.124644643870395,0.0911290685525648,
-0.556714906043359));
#44004=CARTESIAN_POINT('Ctrl Pts',(-0.0845903527646418,0.12917146201847,
-0.559364003146011));
#44005=CARTESIAN_POINT('Ctrl Pts',(-0.0377280931885555,0.141652846864898,
-0.562013100248661));
#44006=CARTESIAN_POINT('Ctrl Pts',(0.00913416638753079,0.154134231711326,
-0.564662197351312));
#44007=CARTESIAN_POINT('Ctrl Pts',(0.06280439443395,0.141054607938275,-0.567311294453962));
#44008=CARTESIAN_POINT('Ctrl Pts',(0.0986698250217679,0.108412193367482,
-0.569960391556612));
#44009=CARTESIAN_POINT('Ctrl Pts',(0.134535255609584,0.0757697787966903,
-0.572609488659263));
#44010=CARTESIAN_POINT('Ctrl Pts',(0.1525958887388,0.0235645734281581,-0.575258585761914));
#44011=CARTESIAN_POINT('Ctrl Pts',(0.144569252880636,-0.0242625052727336,
-0.577907682864564));
#44012=CARTESIAN_POINT('Ctrl Pts',(0.13654261702247,-0.0720895839736307,
-0.580556779967215));
#44013=CARTESIAN_POINT('Ctrl Pts',(0.102428712176916,-0.115538536006886,
-0.583205877069865));
#44014=CARTESIAN_POINT('Ctrl Pts',(0.0578719204427318,-0.134683996320441,
-0.585854974172515));
#44015=CARTESIAN_POINT('Ctrl Pts',(0.0133151287085501,-0.153829456633996,
-0.588504071275166));
#44016=CARTESIAN_POINT('Ctrl Pts',(-0.0416845499142605,-0.148671425227854,
-0.591153168377817));
#44017=CARTESIAN_POINT('Ctrl Pts',(-0.0819046733869025,-0.121575336799696,
-0.593802265480467));
#44018=CARTESIAN_POINT('Ctrl Pts',(-0.12128944446921,-0.0950420209411587,
-0.596396342125549));
#44019=CARTESIAN_POINT('Ctrl Pts',(-0.146502213240191,-0.0474724701172907,
-0.598990418770631));
#44020=CARTESIAN_POINT('Ctrl Pts',(-0.146588075907495,1.88366579988541E-5,
-0.601584495415713));
#44021=CARTESIAN_POINT('Ctrl Pts',(-0.146576141592014,4.24426192752484E-5,
-0.608715504584288));
#44022=CARTESIAN_POINT('Ctrl Pts',(-0.146399213555472,-0.0461586015113418,
-0.606192454876935));
#44023=CARTESIAN_POINT('Ctrl Pts',(-0.122732021093535,-0.0925157336666332,
-0.603669405169581));
#44024=CARTESIAN_POINT('Ctrl Pts',(-0.0851302884352363,-0.119338894404325,
-0.601146355462229));
#44025=CARTESIAN_POINT('Ctrl Pts',(-0.0456500353314474,-0.14750209594057,
-0.598497258359578));
#44026=CARTESIAN_POINT('Ctrl Pts',(0.00919182951988212,-0.154130802575932,
-0.595848161256928));
#44027=CARTESIAN_POINT('Ctrl Pts',(0.0542452362974532,-0.136185138931333,
-0.593199064154278));
#44028=CARTESIAN_POINT('Ctrl Pts',(0.0992986430750269,-0.118239475286734,
-0.590549967051627));
#44029=CARTESIAN_POINT('Ctrl Pts',(0.134563591778846,-0.0757194413621744,
-0.587900869948976));
#44030=CARTESIAN_POINT('Ctrl Pts',(0.143867840189404,-0.0281244072995196,
-0.585251772846325));
#44031=CARTESIAN_POINT('Ctrl Pts',(0.153172088599961,0.0194706267631353,
-0.582602675743675));
#44032=CARTESIAN_POINT('Ctrl Pts',(0.136515636717257,0.0721406609638817,
-0.579953578641024));
#44033=CARTESIAN_POINT('Ctrl Pts',(0.101537009032763,0.105731610804876,
-0.577304481538374));
#44034=CARTESIAN_POINT('Ctrl Pts',(0.0665583813482707,0.139322560645868,
-0.574655384435724));
#44035=CARTESIAN_POINT('Ctrl Pts',(0.0132575778619858,0.153834426127109,
-0.572006287333074));
#44036=CARTESIAN_POINT('Ctrl Pts',(-0.0339220508426392,0.142612174071299,
-0.569357190230423));
#44037=CARTESIAN_POINT('Ctrl Pts',(-0.0811016795472695,0.131389922015488,
-0.566708093127772));
#44038=CARTESIAN_POINT('Ctrl Pts',(-0.122160133470241,0.0944335524226259,
-0.564058996025121));
#44039=CARTESIAN_POINT('Ctrl Pts',(-0.13826831214759,0.0486909805053239,
-0.56140989892247));
#44040=CARTESIAN_POINT('Ctrl Pts',(-0.143729516946169,0.0331827372546198,
-0.560511767476409));
#44041=CARTESIAN_POINT('Ctrl Pts',(-0.146322852208524,0.016664578011516,
-0.559613636030348));
#44042=CARTESIAN_POINT('Ctrl Pts',(-0.146206336570823,0.000110995926028272,
-0.558715504584287));
#44043=CARTESIAN_POINT('Origin',(0.,0.,-1.487));
#44044=CARTESIAN_POINT('',(-0.146150555575012,-7.84903020770444E-5,-0.501584495415714));
#44045=CARTESIAN_POINT('',(-0.146174139180207,-9.5097358159532E-5,-0.508715504584288));
#44046=CARTESIAN_POINT('',(-0.14635,-1.79227059055215E-17,-1.487));
#44047=CARTESIAN_POINT('Ctrl Pts',(-0.146150555575012,-7.84903020770445E-5,
-0.501584495415714));
#44048=CARTESIAN_POINT('Ctrl Pts',(-0.146007294441014,0.0294246106181032,
-0.503183683974809));
#44049=CARTESIAN_POINT('Ctrl Pts',(-0.137347762399225,0.0590050543034279,
-0.504782872533904));
#44050=CARTESIAN_POINT('Ctrl Pts',(-0.120747946537013,0.083119621315723,
-0.506382061093));
#44051=CARTESIAN_POINT('Ctrl Pts',(-0.0932499233332972,0.123066023658725,
-0.50903115819565));
#44052=CARTESIAN_POINT('Ctrl Pts',(-0.0439631442342578,0.14801363562143,
-0.511680255298301));
#44053=CARTESIAN_POINT('Ctrl Pts',(0.00450984179559201,0.146521668593943,
-0.514329352400951));
#44054=CARTESIAN_POINT('Ctrl Pts',(0.0529828278254446,0.145029701566456,
-0.516978449503602));
#44055=CARTESIAN_POINT('Ctrl Pts',(0.100642020786108,0.117098155548773,
-0.519627546606252));
#44056=CARTESIAN_POINT('Ctrl Pts',(0.125631270566046,0.0755362290330639,
-0.522276643708903));
#44057=CARTESIAN_POINT('Ctrl Pts',(0.150620520345982,0.0339743025173592,
-0.524925740811553));
#44058=CARTESIAN_POINT('Ctrl Pts',(0.152939826945199,-0.0212180044963688,
-0.527574837914204));
#44059=CARTESIAN_POINT('Ctrl Pts',(0.131525573671132,-0.0647299120272388,
-0.530223935016854));
#44060=CARTESIAN_POINT('Ctrl Pts',(0.110111320397064,-0.108241819558111,
-0.532873032119505));
#44061=CARTESIAN_POINT('Ctrl Pts',(0.0649635072497097,-0.140073327606124,
-0.535522129222155));
#44062=CARTESIAN_POINT('Ctrl Pts',(0.0167865843058967,-0.145626744205574,
-0.538171226324806));
#44063=CARTESIAN_POINT('Ctrl Pts',(-0.0313903386379162,-0.151180160805023,
-0.540820323427456));
#44064=CARTESIAN_POINT('Ctrl Pts',(-0.0825963713781873,-0.130455485955909,
-0.543469420530107));
#44065=CARTESIAN_POINT('Ctrl Pts',(-0.113348809557938,-0.0929569008324441,
-0.546118517632757));
#44066=CARTESIAN_POINT('Ctrl Pts',(-0.134499681892776,-0.0671661722389087,
-0.547940510227076));
#44067=CARTESIAN_POINT('Ctrl Pts',(-0.145975194912557,-0.0334407205558631,
-0.549762502821394));
#44068=CARTESIAN_POINT('Ctrl Pts',(-0.146238745768959,0.000121916852571603,
-0.551584495415713));
#44069=CARTESIAN_POINT('Ctrl Pts',(-0.146206336570823,0.000110995926028272,
-0.558715504584287));
#44070=CARTESIAN_POINT('Ctrl Pts',(-0.145979181758502,-0.0321612887738781,
-0.556964538927698));
#44071=CARTESIAN_POINT('Ctrl Pts',(-0.135452415366245,-0.0645682087474814,
-0.555213573271108));
#44072=CARTESIAN_POINT('Ctrl Pts',(-0.115796941921911,-0.0898888534149074,
-0.553462607614519));
#44073=CARTESIAN_POINT('Ctrl Pts',(-0.086059489587164,-0.128197341176096,
-0.550813510511868));
#44074=CARTESIAN_POINT('Ctrl Pts',(-0.0354266814859555,-0.150285542456739,
-0.548164413409218));
#44075=CARTESIAN_POINT('Ctrl Pts',(0.0128816545650474,-0.146023973039977,
-0.545515316306567));
#44076=CARTESIAN_POINT('Ctrl Pts',(0.0611899906160503,-0.141762403623215,
-0.542866219203917));
#44077=CARTESIAN_POINT('Ctrl Pts',(0.107173854616843,-0.111151063509043,
-0.540217122101267));
#44078=CARTESIAN_POINT('Ctrl Pts',(0.129745389810405,-0.0682280847573729,
-0.537568024998616));
#44079=CARTESIAN_POINT('Ctrl Pts',(0.152316925003966,-0.0253051060057029,
-0.534918927895966));
#44080=CARTESIAN_POINT('Ctrl Pts',(0.151476131390297,0.0299295113834688,
-0.532269830793315));
#44081=CARTESIAN_POINT('Ctrl Pts',(0.127608590644025,0.0721455842069272,
-0.529620733690664));
#44082=CARTESIAN_POINT('Ctrl Pts',(0.103741049897751,0.114361657030388,
-0.526971636588014));
#44083=CARTESIAN_POINT('Ctrl Pts',(0.0568467620188787,0.143559185288134,
-0.524322539485364));
#44084=CARTESIAN_POINT('Ctrl Pts',(0.00843109735850967,0.146348400483382,
-0.521673442382713));
#44085=CARTESIAN_POINT('Ctrl Pts',(-0.0399845673018567,0.14913761567863,
-0.519024345280063));
#44086=CARTESIAN_POINT('Ctrl Pts',(-0.0899216087437181,0.125518517811378,
-0.516375248177412));
#44087=CARTESIAN_POINT('Ctrl Pts',(-0.118479272546407,0.0863226488448269,
-0.513726151074762));
#44088=CARTESIAN_POINT('Ctrl Pts',(-0.136484445927416,0.0616102486485755,
-0.512055935577937));
#44089=CARTESIAN_POINT('Ctrl Pts',(-0.145991079342716,0.0307059090068275,
-0.510385720081113));
#44090=CARTESIAN_POINT('Ctrl Pts',(-0.146174139180207,-9.5097358159532E-5,
-0.508715504584288));
#44091=CARTESIAN_POINT('Origin',(0.,0.,-1.487));
#44092=CARTESIAN_POINT('',(-0.146526107979514,-8.67851139334103E-5,-0.451584495415714));
#44093=CARTESIAN_POINT('',(-0.146553134476222,-6.73440674254749E-5,-0.458715504584288));
#44094=CARTESIAN_POINT('',(-0.14635,-1.79227059055215E-17,-1.487));
#44095=CARTESIAN_POINT('Ctrl Pts',(-0.146526107979514,-8.67851139334103E-5,
-0.451584495415714));
#44096=CARTESIAN_POINT('Ctrl Pts',(-0.146221087695475,0.0433742309703717,
-0.453955768025573));
#44097=CARTESIAN_POINT('Ctrl Pts',(-0.125655901340594,0.0870858989641212,
-0.456327040635431));
#44098=CARTESIAN_POINT('Ctrl Pts',(-0.0918156512980374,0.114275212611011,
-0.45869831324529));
#44099=CARTESIAN_POINT('Ctrl Pts',(-0.0540105891689472,0.144650097263912,
-0.46134741034794));
#44100=CARTESIAN_POINT('Ctrl Pts',(0.000362446750819749,0.154404219544638,
-0.463996507450591));
#44101=CARTESIAN_POINT('Ctrl Pts',(0.0463683880881343,0.139064411790662,
-0.466645604553242));
#44102=CARTESIAN_POINT('Ctrl Pts',(0.0923743294254462,0.123724604036686,
-0.469294701655892));
#44103=CARTESIAN_POINT('Ctrl Pts',(0.130013176180307,0.0832908662480113,
-0.471943798758543));
#44104=CARTESIAN_POINT('Ctrl Pts',(0.142024034208366,0.0363058087329784,
-0.474592895861193));
#44105=CARTESIAN_POINT('Ctrl Pts',(0.154034892236424,-0.0106792487820545,
-0.477241992963844));
#44106=CARTESIAN_POINT('Ctrl Pts',(0.14041776153768,-0.0642156260234454,
-0.479891090066494));
#44107=CARTESIAN_POINT('Ctrl Pts',(0.107417356597453,-0.0997519400422375,
-0.482540187169145));
#44108=CARTESIAN_POINT('Ctrl Pts',(0.0744169516572266,-0.13528825406103,
-0.485189284271795));
#44109=CARTESIAN_POINT('Ctrl Pts',(0.0220332724755176,-0.152824504857223,
-0.487838381374446));
#44110=CARTESIAN_POINT('Ctrl Pts',(-0.0257109167238908,-0.144318698725396,
-0.490487478477097));
#44111=CARTESIAN_POINT('Ctrl Pts',(-0.0734551059232992,-0.13581289259357,
-0.493136575579747));
#44112=CARTESIAN_POINT('Ctrl Pts',(-0.116559805140407,-0.101265029533724,
-0.495785672682397));
#44113=CARTESIAN_POINT('Ctrl Pts',(-0.135257521094765,-0.0565185016421515,
-0.498434769785048));
#44114=CARTESIAN_POINT('Ctrl Pts',(-0.142667929609352,-0.0387842472500441,
-0.499484678328603));
#44115=CARTESIAN_POINT('Ctrl Pts',(-0.14624461020521,-0.0194480371521357,
-0.500534586872158));
#44116=CARTESIAN_POINT('Ctrl Pts',(-0.146150555575012,-7.84903020770445E-5,
-0.501584495415714));
#44117=CARTESIAN_POINT('Ctrl Pts',(-0.146174139180207,-9.5097358159532E-5,
-0.508715504584288));
#44118=CARTESIAN_POINT('Ctrl Pts',(-0.146281427076904,-0.0181469826561639,
-0.507736622978462));
#44119=CARTESIAN_POINT('Ctrl Pts',(-0.143186151690998,-0.036163373907249,
-0.506757741372636));
#44120=CARTESIAN_POINT('Ctrl Pts',(-0.136722222588937,-0.0528769475012909,
-0.50577885976681));
#44121=CARTESIAN_POINT('Ctrl Pts',(-0.119229222665258,-0.0981080348150043,
-0.503129762664159));
#44122=CARTESIAN_POINT('Ctrl Pts',(-0.0770649366543811,-0.133797569376577,
-0.500480665561509));
#44123=CARTESIAN_POINT('Ctrl Pts',(-0.0295655913606476,-0.143578597061708,
-0.497831568458858));
#44124=CARTESIAN_POINT('Ctrl Pts',(0.0179337539330859,-0.153359624746839,
-0.495182471356208));
#44125=CARTESIAN_POINT('Ctrl Pts',(0.0707681585096733,-0.137232145555528,
-0.492533374253557));
#44126=CARTESIAN_POINT('Ctrl Pts',(0.104708158843949,-0.102592101051803,
-0.489884277150907));
#44127=CARTESIAN_POINT('Ctrl Pts',(0.138648159178227,-0.0679520565480773,
-0.487235180048256));
#44128=CARTESIAN_POINT('Ctrl Pts',(0.153693755270189,-0.0147994467319301,
-0.484586082945605));
#44129=CARTESIAN_POINT('Ctrl Pts',(0.142945149068807,0.0324903383240258,
-0.481936985842954));
#44130=CARTESIAN_POINT('Ctrl Pts',(0.132196542867426,0.0797801233799763,
-0.479287888740303));
#44131=CARTESIAN_POINT('Ctrl Pts',(0.0956537343727117,0.121207083675741,
-0.476638791637653));
#44132=CARTESIAN_POINT('Ctrl Pts',(0.0500749827649339,0.137773124475729,
-0.473989694535003));
#44133=CARTESIAN_POINT('Ctrl Pts',(0.00449623115715341,0.154339165275717,
-0.471340597432353));
#44134=CARTESIAN_POINT('Ctrl Pts',(-0.0501184635636887,0.146044286579924,
-0.468691500329702));
#44135=CARTESIAN_POINT('Ctrl Pts',(-0.0887232101023002,0.116692457836212,
-0.466042403227052));
#44136=CARTESIAN_POINT('Ctrl Pts',(-0.124314338457565,0.089631932954011,
-0.463600103679464));
#44137=CARTESIAN_POINT('Ctrl Pts',(-0.146297537989927,0.0446736938370164,
-0.461157804131876));
#44138=CARTESIAN_POINT('Ctrl Pts',(-0.146553134476222,-6.73440674254749E-5,
-0.458715504584288));
#44139=CARTESIAN_POINT('Origin',(0.,0.,-1.487));
#44140=CARTESIAN_POINT('',(-0.146418337016564,0.000126760208650031,-0.401584495415714));
#44141=CARTESIAN_POINT('',(-0.146378762148194,0.000132588536401338,-0.408715504584289));
#44142=CARTESIAN_POINT('',(-0.14635,-1.79227059055215E-17,-1.487));
#44143=CARTESIAN_POINT('Ctrl Pts',(-0.146418337016564,0.000126760208650031,
-0.401584495415714));
#44144=CARTESIAN_POINT('Ctrl Pts',(-0.146501206702558,0.00920298031833213,
-0.402078754973686));
#44145=CARTESIAN_POINT('Ctrl Pts',(-0.145729860464663,0.0182651549238106,
-0.402573014531657));
#44146=CARTESIAN_POINT('Ctrl Pts',(-0.144053633590977,0.0271567429897478,
-0.403067274089629));
#44147=CARTESIAN_POINT('Ctrl Pts',(-0.135069512428623,0.0748132420974375,
-0.405716371192279));
#44148=CARTESIAN_POINT('Ctrl Pts',(-0.100091164878443,0.117569354400337,
-0.40836546829493));
#44149=CARTESIAN_POINT('Ctrl Pts',(-0.0551594000103929,0.135817445974617,
-0.41101456539758));
#44150=CARTESIAN_POINT('Ctrl Pts',(-0.0102276351423427,0.154065537548897,
-0.413663662500231));
#44151=CARTESIAN_POINT('Ctrl Pts',(0.0446575470435807,0.14780560839456,
-0.416312759602881));
#44152=CARTESIAN_POINT('Ctrl Pts',(0.084326211719807,0.119908415290841,
-0.418961856705532));
#44153=CARTESIAN_POINT('Ctrl Pts',(0.123994876396033,0.0920112221871226,
-0.421610953808183));
#44154=CARTESIAN_POINT('Ctrl Pts',(0.148447023562565,0.0424767651340214,
-0.424260050910833));
#44155=CARTESIAN_POINT('Ctrl Pts',(0.146469081066342,-0.00597882364315429,
-0.426909148013484));
#44156=CARTESIAN_POINT('Ctrl Pts',(0.144491138570118,-0.05443441242033,
-0.429558245116134));
#44157=CARTESIAN_POINT('Ctrl Pts',(0.116083106411145,-0.101811132921574,
-0.432207342218784));
#44158=CARTESIAN_POINT('Ctrl Pts',(0.0742726960689661,-0.126382374796573,
-0.434856439321434));
#44159=CARTESIAN_POINT('Ctrl Pts',(0.0324622857267876,-0.150953616671573,
-0.437505536424085));
#44160=CARTESIAN_POINT('Ctrl Pts',(-0.0227505027985957,-0.152719379920319,
-0.440154633526736));
#44161=CARTESIAN_POINT('Ctrl Pts',(-0.0660454968579486,-0.130869898698522,
-0.442803730629386));
#44162=CARTESIAN_POINT('Ctrl Pts',(-0.109340490917302,-0.109020417476724,
-0.445452827732037));
#44163=CARTESIAN_POINT('Ctrl Pts',(-0.140717690510626,-0.0635556917843813,
-0.448101924834687));
#44164=CARTESIAN_POINT('Ctrl Pts',(-0.145787746138083,-0.0153255054256747,
-0.450751021937338));
#44165=CARTESIAN_POINT('Ctrl Pts',(-0.146319469052927,-0.0102673567270214,
-0.45102884643013));
#44166=CARTESIAN_POINT('Ctrl Pts',(-0.146561844952713,-0.0051787912795902,
-0.451306670922922));
#44167=CARTESIAN_POINT('Ctrl Pts',(-0.146526107979514,-8.67851139334103E-5,
-0.451584495415714));
#44168=CARTESIAN_POINT('Ctrl Pts',(-0.146553134476222,-6.73440674254749E-5,
-0.458715504584288));
#44169=CARTESIAN_POINT('Ctrl Pts',(-0.14657477667343,-0.00385571525995354,
-0.458508707029226));
#44170=CARTESIAN_POINT('Ctrl Pts',(-0.146440641359803,-0.00764252921378538,
-0.458301909474163));
#44171=CARTESIAN_POINT('Ctrl Pts',(-0.146145799317435,-0.0114167888909704,
-0.4580951119191));
#44172=CARTESIAN_POINT('Ctrl Pts',(-0.14236884363758,-0.0597654280828125,
-0.45544601481645));
#44173=CARTESIAN_POINT('Ctrl Pts',(-0.11222013392149,-0.106053927674869,
-0.452796917713799));
#44174=CARTESIAN_POINT('Ctrl Pts',(-0.0695256433820942,-0.129054727302098,
-0.450147820611148));
#44175=CARTESIAN_POINT('Ctrl Pts',(-0.0268311528426982,-0.152055526929327,
-0.447498723508498));
#44176=CARTESIAN_POINT('Ctrl Pts',(0.0284091185200062,-0.15176862659173,
-0.444849626405847));
#44177=CARTESIAN_POINT('Ctrl Pts',(0.0708623946327502,-0.12832559664239,
-0.442200529303197));
#44178=CARTESIAN_POINT('Ctrl Pts',(0.113315670745497,-0.10488256669305,
-0.439551432200546));
#44179=CARTESIAN_POINT('Ctrl Pts',(0.142981951608284,-0.0582834071319632,
-0.436902335097896));
#44180=CARTESIAN_POINT('Ctrl Pts',(0.146256502278931,-0.00989814466686844,
-0.434253237995245));
#44181=CARTESIAN_POINT('Ctrl Pts',(0.149531052949577,0.0384871177982236,
-0.431604140892594));
#44182=CARTESIAN_POINT('Ctrl Pts',(0.126413873428091,0.0886584831673204,
-0.428955043789944));
#44183=CARTESIAN_POINT('Ctrl Pts',(0.0875063296711659,0.117607737815988,
-0.426305946687294));
#44184=CARTESIAN_POINT('Ctrl Pts',(0.0485987859142427,0.146556992464655,
-0.423656849584643));
#44185=CARTESIAN_POINT('Ctrl Pts',(-0.00609912207811904,0.154284136392889,
-0.421007752481993));
#44186=CARTESIAN_POINT('Ctrl Pts',(-0.0515033420254999,0.137245559079037,
-0.418358655379343));
#44187=CARTESIAN_POINT('Ctrl Pts',(-0.0969075619728886,0.120206981765183,
-0.415709558276692));
#44188=CARTESIAN_POINT('Ctrl Pts',(-0.133018093875295,0.0784026832092323,
-0.413060461174041));
#44189=CARTESIAN_POINT('Ctrl Pts',(-0.14327491737069,0.0310038026560445,
-0.410411364071391));
#44190=CARTESIAN_POINT('Ctrl Pts',(-0.145463604151907,0.0208894330992497,
-0.40984607757569));
#44191=CARTESIAN_POINT('Ctrl Pts',(-0.146475052824873,0.0105203165242242,
-0.409280791079989));
#44192=CARTESIAN_POINT('Ctrl Pts',(-0.146378762148194,0.000132588536401338,
-0.408715504584289));
#44193=CARTESIAN_POINT('Origin',(0.,0.,-1.487));
#44194=CARTESIAN_POINT('',(-0.146110499255218,1.76731672666269E-5,-0.351584495415714));
#44195=CARTESIAN_POINT('',(-0.146108623880082,-3.90423146910683E-6,-0.358715504584288));
#44196=CARTESIAN_POINT('',(-0.14635,-1.79227059055215E-17,-1.487));
#44197=CARTESIAN_POINT('Ctrl Pts',(-0.146110499255218,1.76731672666269E-5,
-0.351584495415714));
#44198=CARTESIAN_POINT('Ctrl Pts',(-0.146135644293297,0.0233961899908976,
-0.352850839024449));
#44199=CARTESIAN_POINT('Ctrl Pts',(-0.140852738332724,0.046763976627278,
-0.354117182633184));
#44200=CARTESIAN_POINT('Ctrl Pts',(-0.130201064998778,0.0673544409356841,
-0.355383526241919));
#44201=CARTESIAN_POINT('Ctrl Pts',(-0.107918552754314,0.110428168291655,
-0.358032623344569));
#44202=CARTESIAN_POINT('Ctrl Pts',(-0.062141485911361,0.141347904510693,
-0.36068172044722));
#44203=CARTESIAN_POINT('Ctrl Pts',(-0.0138628855941101,0.145934089381403,
-0.363330817549871));
#44204=CARTESIAN_POINT('Ctrl Pts',(0.0344157147231407,0.150520274252112,
-0.365979914652521));
#44205=CARTESIAN_POINT('Ctrl Pts',(0.085195848514686,0.128772907774494,
-0.368629011755171));
#44206=CARTESIAN_POINT('Ctrl Pts',(0.115190125502062,0.090665169869106,
-0.371278108857822));
#44207=CARTESIAN_POINT('Ctrl Pts',(0.145184402489437,0.0525574319637175,
-0.373927205960472));
#44208=CARTESIAN_POINT('Ctrl Pts',(0.154392822672642,-0.00191067736944712,
-0.376576303063124));
#44209=CARTESIAN_POINT('Ctrl Pts',(0.138592473297352,-0.0477604897995976,
-0.379225400165774));
#44210=CARTESIAN_POINT('Ctrl Pts',(0.122792123922063,-0.0936103022297454,
-0.381874497268425));
#44211=CARTESIAN_POINT('Ctrl Pts',(0.0819830049882875,-0.130841817756885,
-0.384523594371075));
#44212=CARTESIAN_POINT('Ctrl Pts',(0.0348798737952518,-0.142380941296937,
-0.387172691473725));
#44213=CARTESIAN_POINT('Ctrl Pts',(-0.0122232573977919,-0.153920064836991,
-0.389821788576376));
#44214=CARTESIAN_POINT('Ctrl Pts',(-0.0656204008500953,-0.139766796389948,
-0.392470885679027));
#44215=CARTESIAN_POINT('Ctrl Pts',(-0.100824025188982,-0.10641171921018,
-0.395119982781678));
#44216=CARTESIAN_POINT('Ctrl Pts',(-0.129459476625735,-0.0792799192694744,
-0.397274820326357));
#44217=CARTESIAN_POINT('Ctrl Pts',(-0.146057047674118,-0.0394430964399088,
-0.399429657871036));
#44218=CARTESIAN_POINT('Ctrl Pts',(-0.146418337016564,0.000126760208650031,
-0.401584495415714));
#44219=CARTESIAN_POINT('Ctrl Pts',(-0.146378762148194,0.000132588536401338,
-0.408715504584289));
#44220=CARTESIAN_POINT('Ctrl Pts',(-0.146023806678814,-0.0381596012253703,
-0.406631693977338));
#44221=CARTESIAN_POINT('Ctrl Pts',(-0.130616066484444,-0.076704696682295,
-0.404547883370388));
#44222=CARTESIAN_POINT('Ctrl Pts',(-0.103636877624151,-0.10367417867063,
-0.402464072763439));
#44223=CARTESIAN_POINT('Ctrl Pts',(-0.0693388992938295,-0.137959816893702,
-0.399814975660788));
#44224=CARTESIAN_POINT('Ctrl Pts',(-0.0163398275447988,-0.153537630789426,
-0.397165878558138));
#44225=CARTESIAN_POINT('Ctrl Pts',(0.0310553589617483,-0.143263751195025,
-0.394516781455487));
#44226=CARTESIAN_POINT('Ctrl Pts',(0.0784505454682954,-0.132989871600625,
-0.391867684352837));
#44227=CARTESIAN_POINT('Ctrl Pts',(0.120241846732356,-0.0968642985161015,
-0.389218587250186));
#44228=CARTESIAN_POINT('Ctrl Pts',(0.137264083970114,-0.0514539500773136,
-0.386569490147535));
#44229=CARTESIAN_POINT('Ctrl Pts',(0.154286321207871,-0.00604360163852821,
-0.383920393044885));
#44230=CARTESIAN_POINT('Ctrl Pts',(0.146539494419324,0.0486515221545255,
-0.381271295942235));
#44231=CARTESIAN_POINT('Ctrl Pts',(0.117576240538934,0.087548645834438,
-0.378622198839584));
#44232=CARTESIAN_POINT('Ctrl Pts',(0.0886129866585401,0.126445769514355,
-0.375973101736933));
#44233=CARTESIAN_POINT('Ctrl Pts',(0.0384333056862997,0.149544893081133,
-0.373324004634282));
#44234=CARTESIAN_POINT('Ctrl Pts',(-0.00995077527981938,0.146252930904114,
-0.370674907531632));
#44235=CARTESIAN_POINT('Ctrl Pts',(-0.0583348562459329,0.142960968727096,
-0.368025810428981));
#44236=CARTESIAN_POINT('Ctrl Pts',(-0.104923337205923,0.113277920806288,
-0.365376713326331));
#44237=CARTESIAN_POINT('Ctrl Pts',(-0.128351088578806,0.0708162113315071,
-0.362727616223681));
#44238=CARTESIAN_POINT('Ctrl Pts',(-0.140178357811268,0.0493798360671646,
-0.361390245677217));
#44239=CARTESIAN_POINT('Ctrl Pts',(-0.146102800938292,0.0246866455660807,
-0.360052875130753));
#44240=CARTESIAN_POINT('Ctrl Pts',(-0.146108662346803,-3.9036092742423E-6,
-0.358715504584288));
#44241=CARTESIAN_POINT('Origin',(0.,0.,-1.487));
#44242=CARTESIAN_POINT('',(-0.146353309704914,-0.000134325699099658,-0.301584495415715));
#44243=CARTESIAN_POINT('',(-0.146393127902371,-0.000130920977438367,-0.308715504584288));
#44244=CARTESIAN_POINT('',(-0.14635,-1.79227059055215E-17,-1.487));
#44245=CARTESIAN_POINT('Ctrl Pts',(-0.146353309704914,-0.000134325699099658,
-0.301584495415715));
#44246=CARTESIAN_POINT('Ctrl Pts',(-0.146007391017754,0.0373405958603415,
-0.303622923075213));
#44247=CARTESIAN_POINT('Ctrl Pts',(-0.131331784984381,0.0750562040210813,
-0.305661350734711));
#44248=CARTESIAN_POINT('Ctrl Pts',(-0.105395382320675,0.101885972665794,
-0.307699778394209));
#44249=CARTESIAN_POINT('Ctrl Pts',(-0.0716889866929201,0.136753367665229,
-0.31034887549686));
#44250=CARTESIAN_POINT('Ctrl Pts',(-0.0189641785476722,0.153235616985242,
-0.312997972599511));
#44251=CARTESIAN_POINT('Ctrl Pts',(0.0285998386951484,0.143774084129184,
-0.315647069702161));
#44252=CARTESIAN_POINT('Ctrl Pts',(0.0761638559379663,0.134312551273126,
-0.318296166804812));
#44253=CARTESIAN_POINT('Ctrl Pts',(0.118567082278357,0.0989072362409995,
-0.320945263907462));
#44254=CARTESIAN_POINT('Ctrl Pts',(0.136363714660583,0.0537947522026214,
-0.323594361010112));
#44255=CARTESIAN_POINT('Ctrl Pts',(0.154160347042808,0.00868226816424576,
-0.326243458112763));
#44256=CARTESIAN_POINT('Ctrl Pts',(0.147350385466869,-0.0461373848803806,
-0.328892555215414));
#44257=CARTESIAN_POINT('Ctrl Pts',(0.119056827474505,-0.0855243232787071,
-0.331541652318064));
#44258=CARTESIAN_POINT('Ctrl Pts',(0.0907632694821371,-0.124911261677038,
-0.334190749420715));
#44259=CARTESIAN_POINT('Ctrl Pts',(0.0409861150733369,-0.148865485429065,
-0.336839846523365));
#44260=CARTESIAN_POINT('Ctrl Pts',(-0.00744720433101837,-0.146401766342577,
-0.339488943626016));
#44261=CARTESIAN_POINT('Ctrl Pts',(-0.0558805237353709,-0.143938047256089,
-0.342138040728666));
#44262=CARTESIAN_POINT('Ctrl Pts',(-0.102970008135279,-0.11505638533109,
-0.344787137831317));
#44263=CARTESIAN_POINT('Ctrl Pts',(-0.127120771512246,-0.0730016951221395,
-0.347436234933968));
#44264=CARTESIAN_POINT('Ctrl Pts',(-0.139726784484295,-0.0510503405403165,
-0.348818988427883));
#44265=CARTESIAN_POINT('Ctrl Pts',(-0.146083042734713,-0.0255099368727371,
-0.350201741921799));
#44266=CARTESIAN_POINT('Ctrl Pts',(-0.146110499255218,1.76731672666269E-5,
-0.351584495415714));
#44267=CARTESIAN_POINT('Ctrl Pts',(-0.146108662346803,-3.9036092742423E-6,
-0.358715504584288));
#44268=CARTESIAN_POINT('Ctrl Pts',(-0.1461144113632,-0.0242210131648569,
-0.357403778028102));
#44269=CARTESIAN_POINT('Ctrl Pts',(-0.140426379341273,-0.0484355817180389,
-0.356092051471915));
#44270=CARTESIAN_POINT('Ctrl Pts',(-0.129029699738514,-0.0695720799753903,
-0.354780324915729));
#44271=CARTESIAN_POINT('Ctrl Pts',(-0.106013537739563,-0.112258290778747,
-0.352131227813079));
#44272=CARTESIAN_POINT('Ctrl Pts',(-0.0597141919558894,-0.142390341356705,
-0.349482130710428));
#44273=CARTESIAN_POINT('Ctrl Pts',(-0.0113641967350396,-0.14614989825272,
-0.346833033607778));
#44274=CARTESIAN_POINT('Ctrl Pts',(0.0369857984858101,-0.149909455148735,
-0.344183936505127));
#44275=CARTESIAN_POINT('Ctrl Pts',(0.0873864431438355,-0.127296518362809,
-0.341534839402477));
#44276=CARTESIAN_POINT('Ctrl Pts',(0.11672437784428,-0.0886812118973283,
-0.338885742299826));
#44277=CARTESIAN_POINT('Ctrl Pts',(0.146062312544727,-0.0500659054318454,
-0.336236645197175));
#44278=CARTESIAN_POINT('Ctrl Pts',(0.15433753728759,0.00455177071319376,
-0.333587548094525));
#44279=CARTESIAN_POINT('Ctrl Pts',(0.137755095781102,0.0501245579836111,
-0.330938450991874));
#44280=CARTESIAN_POINT('Ctrl Pts',(0.121172654274615,0.0956973452540258,
-0.328289353889224));
#44281=CARTESIAN_POINT('Ctrl Pts',(0.0797325465187796,0.13222524364982,
-0.325640256786573));
#44282=CARTESIAN_POINT('Ctrl Pts',(0.032438896576232,0.14295683165078,-0.322991159683923));
#44283=CARTESIAN_POINT('Ctrl Pts',(-0.0148547533663157,0.153688419651741,
-0.320342062581272));
#44284=CARTESIAN_POINT('Ctrl Pts',(-0.0680019454955752,0.138623697257868,
-0.317692965478621));
#44285=CARTESIAN_POINT('Ctrl Pts',(-0.102629774249709,0.104671233699461,
-0.315043868375971));
#44286=CARTESIAN_POINT('Ctrl Pts',(-0.130203634220464,0.0776351615717817,
-0.312934413778743));
#44287=CARTESIAN_POINT('Ctrl Pts',(-0.146034721274829,0.0386227352408806,
-0.310824959181516));
#44288=CARTESIAN_POINT('Ctrl Pts',(-0.146393127902371,-0.000130920977438367,
-0.308715504584288));
#44289=CARTESIAN_POINT('Origin',(0.,0.,-1.487));
#44290=CARTESIAN_POINT('',(-0.146567193673927,5.3661049326555E-5,-0.251584495415715));
#44291=CARTESIAN_POINT('',(-0.146544032588096,7.46631685089006E-5,-0.258715504584289));
#44292=CARTESIAN_POINT('',(-0.14635,-1.79227059055215E-17,-1.487));
#44293=CARTESIAN_POINT('Ctrl Pts',(-0.146567193673927,5.3661049326555E-5,
-0.251584495415715));
#44294=CARTESIAN_POINT('Ctrl Pts',(-0.146581110999607,0.00300989945102091,
-0.251745910023326));
#44295=CARTESIAN_POINT('Ctrl Pts',(-0.146499434569904,0.00596535408209463,
-0.251907324630937));
#44296=CARTESIAN_POINT('Ctrl Pts',(-0.146319731190637,0.00891483621586715,
-0.252068739238548));
#44297=CARTESIAN_POINT('Ctrl Pts',(-0.143370483235966,0.0573210163660909,
-0.254717836341199));
#44298=CARTESIAN_POINT('Ctrl Pts',(-0.114018095543567,0.104118529904453,
-0.257366933443849));
#44299=CARTESIAN_POINT('Ctrl Pts',(-0.0717233539896174,0.127846386468801,
-0.2600160305465));
#44300=CARTESIAN_POINT('Ctrl Pts',(-0.0294286124356675,0.151574243033149,
-0.26266512764915));
#44301=CARTESIAN_POINT('Ctrl Pts',(0.0258084829798361,0.152232442623483,
-0.265314224751801));
#44302=CARTESIAN_POINT('Ctrl Pts',(0.0686566126486147,0.129519139821814,
-0.267963321854451));
#44303=CARTESIAN_POINT('Ctrl Pts',(0.111504742317396,0.106805837020143,
-0.270612418957102));
#44304=CARTESIAN_POINT('Ctrl Pts',(0.141963906239453,0.060721031826464,
-0.273261516059753));
#44305=CARTESIAN_POINT('Ctrl Pts',(0.14606575922093,0.0123988718749984,
-0.275910613162403));
#44306=CARTESIAN_POINT('Ctrl Pts',(0.150167612202407,-0.0359232880764644,
-0.278559710265054));
#44307=CARTESIAN_POINT('Ctrl Pts',(0.127912154243313,-0.08648280278571,
-0.281208807367704));
#44308=CARTESIAN_POINT('Ctrl Pts',(0.089505572224467,-0.116093456238312,
-0.283857904470355));
#44309=CARTESIAN_POINT('Ctrl Pts',(0.0510989902056226,-0.145704109690911,
-0.286507001573005));
#44310=CARTESIAN_POINT('Ctrl Pts',(-0.00345871587297271,-0.154365901886864,
-0.289156098675655));
#44311=CARTESIAN_POINT('Ctrl Pts',(-0.0491477892818325,-0.138106599586265,
-0.291805195778306));
#44312=CARTESIAN_POINT('Ctrl Pts',(-0.0948368626906975,-0.121847297285664,
-0.294454292880956));
#44313=CARTESIAN_POINT('Ctrl Pts',(-0.131657303429827,-0.0806669004885042,
-0.297103389983607));
#44314=CARTESIAN_POINT('Ctrl Pts',(-0.142723532244259,-0.0334504317504969,
-0.299752487086258));
#44315=CARTESIAN_POINT('Ctrl Pts',(-0.1452745175521,-0.0225660988798718,
-0.30036315652941));
#44316=CARTESIAN_POINT('Ctrl Pts',(-0.146456939564468,-0.011361012785221,
-0.300973825972562));
#44317=CARTESIAN_POINT('Ctrl Pts',(-0.146353309704914,-0.000134325699099658,
-0.301584495415715));
#44318=CARTESIAN_POINT('Ctrl Pts',(-0.146393127902371,-0.000130920977438367,
-0.308715504584288));
#44319=CARTESIAN_POINT('Ctrl Pts',(-0.146484815796816,-0.0100449149375058,
-0.308175862078865));
#44320=CARTESIAN_POINT('Ctrl Pts',(-0.145563904698664,-0.0199419738644643,
-0.307636219573443));
#44321=CARTESIAN_POINT('Ctrl Pts',(-0.143567948415088,-0.0296172570403707,
-0.30709657706802));
#44322=CARTESIAN_POINT('Ctrl Pts',(-0.133769828447326,-0.0771130794988537,
-0.304447479965369));
#44323=CARTESIAN_POINT('Ctrl Pts',(-0.0980651231327929,-0.11926451969288,
-0.301798382862718));
#44324=CARTESIAN_POINT('Ctrl Pts',(-0.0528277437898429,-0.136741241813826,
-0.299149285760068));
#44325=CARTESIAN_POINT('Ctrl Pts',(-0.00759036444689028,-0.154217963934774,
-0.296500188657417));
#44326=CARTESIAN_POINT('Ctrl Pts',(0.0471796889244828,-0.147019967982639,
-0.293851091554767));
#44327=CARTESIAN_POINT('Ctrl Pts',(0.0863652787115969,-0.118448201167358,
-0.291201994452116));
#44328=CARTESIAN_POINT('Ctrl Pts',(0.125550868498709,-0.0898764343520795,
-0.288552897349466));
#44329=CARTESIAN_POINT('Ctrl Pts',(0.149151994701565,-0.0399308966736649,
-0.285903800246815));
#44330=CARTESIAN_POINT('Ctrl Pts',(0.146345357028125,0.00848376113654518,
-0.283254703144165));
#44331=CARTESIAN_POINT('Ctrl Pts',(0.143538719354685,0.0568984189467553,
-0.280605606041514));
#44332=CARTESIAN_POINT('Ctrl Pts',(0.114324317804944,0.103782196888758,
-0.277956508938864));
#44333=CARTESIAN_POINT('Ctrl Pts',(0.0720996588413956,0.127634544390087,
-0.275307411836213));
#44334=CARTESIAN_POINT('Ctrl Pts',(0.0298749998778472,0.151486891891416,
-0.272658314733563));
#44335=CARTESIAN_POINT('Ctrl Pts',(-0.0253599164995117,0.152307808952074,
-0.270009217630912));
#44336=CARTESIAN_POINT('Ctrl Pts',(-0.0682747699736325,0.129720829136157,
-0.267360120528262));
#44337=CARTESIAN_POINT('Ctrl Pts',(-0.111189623447756,0.107133849320239,
-0.264711023425611));
#44338=CARTESIAN_POINT('Ctrl Pts',(-0.141784414018642,0.0611389726277425,
-0.26206192632296));
#44339=CARTESIAN_POINT('Ctrl Pts',(-0.146028599123545,0.0128291061540969,
-0.25941282922031));
#44340=CARTESIAN_POINT('Ctrl Pts',(-0.146400999570288,0.00859022038162686,
-0.259180387674969));
#44341=CARTESIAN_POINT('Ctrl Pts',(-0.146570527904556,0.00433351160816856,
-0.258947946129629));
#44342=CARTESIAN_POINT('Ctrl Pts',(-0.146544032588096,7.46631685089006E-5,
-0.258715504584289));
#44343=CARTESIAN_POINT('Origin',(0.,0.,-1.487));
#44344=CARTESIAN_POINT('',(-0.146191577767457,0.000104459130465896,-0.201584495415715));
#44345=CARTESIAN_POINT('',(-0.146165083001347,8.93600630285772E-5,-0.208715504584289));
#44346=CARTESIAN_POINT('',(-0.14635,-1.79227059055215E-17,-1.487));
#44347=CARTESIAN_POINT('Ctrl Pts',(-0.146191577767457,0.000104459130465896,
-0.201584495415715));
#44348=CARTESIAN_POINT('Ctrl Pts',(-0.14630480808494,0.0173142675966806,
-0.202517994074089));
#44349=CARTESIAN_POINT('Ctrl Pts',(-0.143497504164964,0.0344883226025476,
-0.203451492732464));
#44350=CARTESIAN_POINT('Ctrl Pts',(-0.137606839493189,0.0505301470283315,
-0.204384991390838));
#44351=CARTESIAN_POINT('Ctrl Pts',(-0.12089021909455,0.0960538874497384,
-0.207034088493489));
#44352=CARTESIAN_POINT('Ctrl Pts',(-0.0793426850817587,0.13245955120465,
-0.209683185596139));
#44353=CARTESIAN_POINT('Ctrl Pts',(-0.0320176263359178,0.143051772611944,
-0.21233228269879));
#44354=CARTESIAN_POINT('Ctrl Pts',(0.0153074324099204,0.153643994019238,
-0.21498137980144));
#44355=CARTESIAN_POINT('Ctrl Pts',(0.0684100158888131,0.138422773078912,
-0.217630476904091));
#44356=CARTESIAN_POINT('Ctrl Pts',(0.102937675700814,0.104368448115231,
-0.220279574006741));
#44357=CARTESIAN_POINT('Ctrl Pts',(0.13746533551282,0.0703141231515449,
-0.222928671109392));
#44358=CARTESIAN_POINT('Ctrl Pts',(0.153418071657937,0.0174266941644967,
-0.225577768212043));
#44359=CARTESIAN_POINT('Ctrl Pts',(0.143480078445581,-0.030040058737127,
-0.228226865314694));
#44360=CARTESIAN_POINT('Ctrl Pts',(0.133542085233227,-0.0775068116387426,
-0.230875962417345));
#44361=CARTESIAN_POINT('Ctrl Pts',(0.0977133626634111,-0.119552888454932,
-0.233525059519995));
#44362=CARTESIAN_POINT('Ctrl Pts',(0.0524246954330384,-0.136896272227596,
-0.236174156622645));
#44363=CARTESIAN_POINT('Ctrl Pts',(0.00713602820266312,-0.154239656000261,
-0.238823253725296));
#44364=CARTESIAN_POINT('Ctrl Pts',(-0.0476125836882674,-0.146880346729396,
-0.241472350827946));
#44365=CARTESIAN_POINT('Ctrl Pts',(-0.086713835525261,-0.11819326871292,
-0.244121447930597));
#44366=CARTESIAN_POINT('Ctrl Pts',(-0.123432572498585,-0.0912541498168937,
-0.246609130425636));
#44367=CARTESIAN_POINT('Ctrl Pts',(-0.146352703250883,-0.0455071629176186,
-0.249096812920676));
#44368=CARTESIAN_POINT('Ctrl Pts',(-0.146567193673927,5.3661049326555E-5,
-0.251584495415715));
#44369=CARTESIAN_POINT('Ctrl Pts',(-0.146544032588096,7.46631685089006E-5,
-0.258715504584289));
#44370=CARTESIAN_POINT('Ctrl Pts',(-0.146268565249962,-0.0442038660177313,
-0.256298849026979));
#44371=CARTESIAN_POINT('Ctrl Pts',(-0.124804097187225,-0.0887136805030915,
-0.253882193469668));
#44372=CARTESIAN_POINT('Ctrl Pts',(-0.0898471773911594,-0.115829281451386,
-0.251465537912358));
#44373=CARTESIAN_POINT('Ctrl Pts',(-0.0515279909149432,-0.145552946328443,
-0.248816440809708));
#44374=CARTESIAN_POINT('Ctrl Pts',(0.00300396167641406,-0.154375419827755,
-0.246167343707057));
#44375=CARTESIAN_POINT('Ctrl Pts',(0.0487407340099472,-0.138250781462385,
-0.243518246604407));
#44376=CARTESIAN_POINT('Ctrl Pts',(0.0944775063434778,-0.122126143097015,
-0.240869149501756));
#44377=CARTESIAN_POINT('Ctrl Pts',(0.131419098419185,-0.0810543928669649,
-0.238220052399106));
#44378=CARTESIAN_POINT('Ctrl Pts',(0.142624371884594,-0.0338707288247468,
-0.235570955296455));
#44379=CARTESIAN_POINT('Ctrl Pts',(0.153829645350003,0.0133129352174713,
-0.232921858193804));
#44380=CARTESIAN_POINT('Ctrl Pts',(0.139298600205113,0.0666085130718572,
-0.230272761091154));
#44381=CARTESIAN_POINT('Ctrl Pts',(0.105695065275732,0.10157505059336,-0.227623663988504));
#44382=CARTESIAN_POINT('Ctrl Pts',(0.0720915303463524,0.136541588114861,
-0.224974566885853));
#44383=CARTESIAN_POINT('Ctrl Pts',(0.0194155056324831,0.153179085303482,
-0.222325469783203));
#44384=CARTESIAN_POINT('Ctrl Pts',(-0.028176177159521,0.143857710143993,
-0.219676372680552));
#44385=CARTESIAN_POINT('Ctrl Pts',(-0.0757678599515305,0.134536334984504,
-0.217027275577902));
#44386=CARTESIAN_POINT('Ctrl Pts',(-0.118275200821673,0.0992560874768987,
-0.214378178475251));
#44387=CARTESIAN_POINT('Ctrl Pts',(-0.136204650575506,0.0541962257673195,
-0.2117290813726));
#44388=CARTESIAN_POINT('Ctrl Pts',(-0.143003416533825,0.0371097307502518,
-0.210724555776496));
#44389=CARTESIAN_POINT('Ctrl Pts',(-0.146268147255594,0.0186170328565388,
-0.209720030180393));
#44390=CARTESIAN_POINT('Ctrl Pts',(-0.146165083001347,8.93600630285772E-5,
-0.208715504584289));
#44391=CARTESIAN_POINT('Origin',(0.,0.,-1.487));
#44392=CARTESIAN_POINT('',(-0.146187581536877,-0.000102482699927964,-0.151584495415715));
#44393=CARTESIAN_POINT('',(-0.146217633328538,-0.000115290056034918,-0.158715504584289));
#44394=CARTESIAN_POINT('',(-0.14635,-1.79227059055215E-17,-1.487));
#44395=CARTESIAN_POINT('Ctrl Pts',(-0.146187581536877,-0.000102482699927964,
-0.151584495415715));
#44396=CARTESIAN_POINT('Ctrl Pts',(-0.145984962940154,0.0313434842482817,
-0.153290078124853));
#44397=CARTESIAN_POINT('Ctrl Pts',(-0.136039089214935,0.0629063216346523,
-0.154995660833991));
#44398=CARTESIAN_POINT('Ctrl Pts',(-0.117317824998014,0.0878946281013525,
-0.156701243543129));
#44399=CARTESIAN_POINT('Ctrl Pts',(-0.0882401106606897,0.126706261161662,
-0.15935034064578));
#44400=CARTESIAN_POINT('Ctrl Pts',(-0.0379926020706468,0.149657464192199,
-0.16199943774843));
#44401=CARTESIAN_POINT('Ctrl Pts',(0.0103815712888817,0.146222984256681,
-0.164648534851081));
#44402=CARTESIAN_POINT('Ctrl Pts',(0.0587557446484075,0.142788504321163,
-0.167297631953731));
#44403=CARTESIAN_POINT('Ctrl Pts',(0.105256582777419,0.112968341419593,
-0.169946729056382));
#44404=CARTESIAN_POINT('Ctrl Pts',(0.128559146939399,0.0704378009967336,
-0.172595826159032));
#44405=CARTESIAN_POINT('Ctrl Pts',(0.151861711101382,0.0279072605738691,
-0.175244923261682));
#44406=CARTESIAN_POINT('Ctrl Pts',(0.151966001296327,-0.0273336573702886,
-0.177894020364333));
#44407=CARTESIAN_POINT('Ctrl Pts',(0.128824191611502,-0.0699518809554031,
-0.180543117466984));
#44408=CARTESIAN_POINT('Ctrl Pts',(0.105682381926679,-0.112570104540515,
-0.183192214569634));
#44409=CARTESIAN_POINT('Ctrl Pts',(0.0592944723620888,-0.142565633766586,
-0.185841311672285));
#44410=CARTESIAN_POINT('Ctrl Pts',(0.0109336115367446,-0.146182742475658,
-0.188490408774935));
#44411=CARTESIAN_POINT('Ctrl Pts',(-0.0374272492885997,-0.14979985118473,
-0.191139505877586));
#44412=CARTESIAN_POINT('Ctrl Pts',(-0.0877610613746981,-0.127038539376803,
-0.193788602980236));
#44413=CARTESIAN_POINT('Ctrl Pts',(-0.116985114025505,-0.0883369749288895,
-0.196437700082887));
#44414=CARTESIAN_POINT('Ctrl Pts',(-0.135911086657086,-0.0632732112444792,
-0.198153298527163));
#44415=CARTESIAN_POINT('Ctrl Pts',(-0.145983481317853,-0.0315239962144383,
-0.199868896971439));
#44416=CARTESIAN_POINT('Ctrl Pts',(-0.146191577767457,0.000104459130465896,
-0.201584495415715));
#44417=CARTESIAN_POINT('Ctrl Pts',(-0.146165083001347,8.93600630285772E-5,
-0.208715504584289));
#44418=CARTESIAN_POINT('Ctrl Pts',(-0.145996350082509,-0.0302434486548492,
-0.207070933077742));
#44419=CARTESIAN_POINT('Ctrl Pts',(-0.136800914172156,-0.0606700006186409,
-0.205426361571195));
#44420=CARTESIAN_POINT('Ctrl Pts',(-0.119308252051597,-0.0851732277138702,
-0.203781790064649));
#44421=CARTESIAN_POINT('Ctrl Pts',(-0.0911308451363325,-0.124643343573932,
-0.201132692961998));
#44422=CARTESIAN_POINT('Ctrl Pts',(-0.0414244726682828,-0.148744099382509,
-0.198483595859348));
#44423=CARTESIAN_POINT('Ctrl Pts',(0.00701589397457254,-0.146423068406191,
-0.195834498756698));
#44424=CARTESIAN_POINT('Ctrl Pts',(0.0554562606174306,-0.144102037429874,
-0.193185401654047));
#44425=CARTESIAN_POINT('Ctrl Pts',(0.102630621435091,-0.115359219668657,
-0.190536304551397));
#44426=CARTESIAN_POINT('Ctrl Pts',(0.126905166768256,-0.0733758568444998,
-0.187887207448746));
#44427=CARTESIAN_POINT('Ctrl Pts',(0.151179712101423,-0.0313924940203378,
-0.185238110346095));
#44428=CARTESIAN_POINT('Ctrl Pts',(0.152554441950085,0.0238314138667743,
-0.182589013243444));
#44429=CARTESIAN_POINT('Ctrl Pts',(0.130398915371771,0.0669705950335863,
-0.179939916140793));
#44430=CARTESIAN_POINT('Ctrl Pts',(0.10824338879346,0.110109776200391,-0.177290819038143));
#44431=CARTESIAN_POINT('Ctrl Pts',(0.0625576057881857,0.141164230646906,
-0.174641721935492));
#44432=CARTESIAN_POINT('Ctrl Pts',(0.0142927255765135,0.145892617156203,
-0.171992624832842));
#44433=CARTESIAN_POINT('Ctrl Pts',(-0.0339721546351587,0.150621003665501,
-0.169343527730192));
#44434=CARTESIAN_POINT('Ctrl Pts',(-0.0848161320532254,0.129023322237581,
-0.166694430627541));
#44435=CARTESIAN_POINT('Ctrl Pts',(-0.114922538535846,0.0910041087871558,
-0.164045333524891));
#44436=CARTESIAN_POINT('Ctrl Pts',(-0.135113316796115,0.0655066284136506,
-0.162268723878024));
#44437=CARTESIAN_POINT('Ctrl Pts',(-0.14597700518956,0.0326232731273325,
-0.160492114231156));
#44438=CARTESIAN_POINT('Ctrl Pts',(-0.146217633328538,-0.000115290056034918,
-0.158715504584289));
#44439=CARTESIAN_POINT('Origin',(0.,0.,-1.487));
#44440=CARTESIAN_POINT('',(-0.146564414435351,-5.66789191273343E-5,-0.101584495415716));
#44441=CARTESIAN_POINT('',(-0.146581435366625,-3.40469869341234E-5,-0.10871550458429));
#44442=CARTESIAN_POINT('',(-0.14635,-1.79227059055215E-17,-1.487));
#44443=CARTESIAN_POINT('Ctrl Pts',(-0.146564414435351,-5.66789191273343E-5,
-0.101584495415716));
#44444=CARTESIAN_POINT('Ctrl Pts',(-0.146340217108257,0.0453231005231363,
-0.104062162175617));
#44445=CARTESIAN_POINT('Ctrl Pts',(-0.12362882200582,0.0908964496879157,
-0.106539828935518));
#44446=CARTESIAN_POINT('Ctrl Pts',(-0.0871594563241677,0.117864973908624,
-0.109017495695419));
#44447=CARTESIAN_POINT('Ctrl Pts',(-0.0481667666992645,0.14669945662925,
-0.11166659279807));
#44448=CARTESIAN_POINT('Ctrl Pts',(0.00655359128472432,0.154265503361126,
-0.11431568990072));
#44449=CARTESIAN_POINT('Ctrl Pts',(0.0519074034152914,0.137093261865771,
-0.116964787003371));
#44450=CARTESIAN_POINT('Ctrl Pts',(0.0972612155458585,0.119921020370417,
-0.119613884106021));
#44451=CARTESIAN_POINT('Ctrl Pts',(0.133248481823007,0.0780104906478297,
-0.122262981208672));
#44452=CARTESIAN_POINT('Ctrl Pts',(0.143365640264857,0.0305815918194669,
-0.124912078311322));
#44453=CARTESIAN_POINT('Ctrl Pts',(0.153482798706707,-0.016847307008896,
-0.127561175413973));
#44454=CARTESIAN_POINT('Ctrl Pts',(0.137729849313264,-0.0697945749430308,
-0.130210272516623));
#44455=CARTESIAN_POINT('Ctrl Pts',(0.10333101412408,-0.103979023385252,
-0.132859369619274));
#44456=CARTESIAN_POINT('Ctrl Pts',(0.0689321789348948,-0.138163471827475,
-0.135508466721924));
#44457=CARTESIAN_POINT('Ctrl Pts',(0.015887457949965,-0.153585100777775,
-0.138157563824575));
#44458=CARTESIAN_POINT('Ctrl Pts',(-0.0314772552874305,-0.143171648821433,
-0.140806660927225));
#44459=CARTESIAN_POINT('Ctrl Pts',(-0.078841968524826,-0.132758196865091,
-0.143455758029876));
#44460=CARTESIAN_POINT('Ctrl Pts',(-0.12052667401469,-0.0965096640021071,
-0.146104855132527));
#44461=CARTESIAN_POINT('Ctrl Pts',(-0.137415066717318,-0.0510493660255724,
-0.148753952235178));
#44462=CARTESIAN_POINT('Ctrl Pts',(-0.143430112969218,-0.0348580208946959,
-0.14969746662869));
#44463=CARTESIAN_POINT('Ctrl Pts',(-0.146299668486034,-0.0174981342122152,
-0.150640981022202));
#44464=CARTESIAN_POINT('Ctrl Pts',(-0.146187581536877,-0.000102482699927964,
-0.151584495415715));
#44465=CARTESIAN_POINT('Ctrl Pts',(-0.146217633328538,-0.000115290056034918,
-0.158715504584289));
#44466=CARTESIAN_POINT('Ctrl Pts',(-0.146335805056997,-0.0161930963137119,
-0.157843017128505));
#44467=CARTESIAN_POINT('Ctrl Pts',(-0.143891948052167,-0.0322359821699961,
-0.156970529672722));
#44468=CARTESIAN_POINT('Ctrl Pts',(-0.138732566475733,-0.0473520089990637,
-0.156098042216939));
#44469=CARTESIAN_POINT('Ctrl Pts',(-0.123067352385828,-0.0932481678619148,
-0.153448945114288));
#44470=CARTESIAN_POINT('Ctrl Pts',(-0.082368088658853,-0.130599740114677,
-0.150799848011638));
#44471=CARTESIAN_POINT('Ctrl Pts',(-0.0352991550669112,-0.142277571968052,
-0.148150750908987));
#44472=CARTESIAN_POINT('Ctrl Pts',(0.011769778525028,-0.153955403821426,
-0.145501653806337));
#44473=CARTESIAN_POINT('Ctrl Pts',(0.0652083819819311,-0.13995949527541,
-0.142852556703686));
#44474=CARTESIAN_POINT('Ctrl Pts',(0.100510113056305,-0.106708268520858,
-0.140203459601036));
#44475=CARTESIAN_POINT('Ctrl Pts',(0.135811844130678,-0.0734570417663067,
-0.137554362498385));
#44476=CARTESIAN_POINT('Ctrl Pts',(0.152976702822525,-0.0209504968032168,
-0.134905265395735));
#44477=CARTESIAN_POINT('Ctrl Pts',(0.144133008567398,0.0267322625321848,
-0.132256168293084));
#44478=CARTESIAN_POINT('Ctrl Pts',(0.135289314312271,0.0744150218675864,
-0.129607071190434));
#44479=CARTESIAN_POINT('Ctrl Pts',(0.10043706711017,0.117273995575304,-0.126957974087783));
#44480=CARTESIAN_POINT('Ctrl Pts',(0.055559255904687,0.135654367406582,
-0.124308876985133));
#44481=CARTESIAN_POINT('Ctrl Pts',(0.0106814446992037,0.15403473923786,
-0.121659779882482));
#44482=CARTESIAN_POINT('Ctrl Pts',(-0.0442219305096567,0.147936509192702,
-0.119010682779832));
#44483=CARTESIAN_POINT('Ctrl Pts',(-0.0839726079418993,0.120156300644783,
-0.116361585677182));
#44484=CARTESIAN_POINT('Ctrl Pts',(-0.122216695312928,0.0934289895265518,
-0.113812891979551));
#44485=CARTESIAN_POINT('Ctrl Pts',(-0.146434922801896,0.0466320910035745,
-0.11126419828192));
#44486=CARTESIAN_POINT('Ctrl Pts',(-0.146581435366625,-3.40469869341234E-5,
-0.10871550458429));
#44487=CARTESIAN_POINT('Origin',(0.,0.,-1.487));
#44488=CARTESIAN_POINT('',(-0.146359156828661,0.000134286233873571,-0.051584495415716));
#44489=CARTESIAN_POINT('',(-0.146319403921505,0.000134192518820611,-0.0587155045842896));
#44490=CARTESIAN_POINT('',(-0.14635,-1.79227059055215E-17,-1.487));
#44491=CARTESIAN_POINT('Ctrl Pts',(-0.146359156828661,0.000134286233873571,
-0.051584495415716));
#44492=CARTESIAN_POINT('Ctrl Pts',(-0.146462627304662,0.0111769826627363,
-0.05218514912373));
#44493=CARTESIAN_POINT('Ctrl Pts',(-0.145320316174143,0.0221985827027607,
-0.0527858028317441));
#44494=CARTESIAN_POINT('Ctrl Pts',(-0.142852300121244,0.0329144147112076,
-0.0533864565397581));
#44495=CARTESIAN_POINT('Ctrl Pts',(-0.13196746899842,0.0801750561545543,
-0.0560355536424086));
#44496=CARTESIAN_POINT('Ctrl Pts',(-0.0952960250695133,0.121488128341987,
-0.0586846507450591));
#44497=CARTESIAN_POINT('Ctrl Pts',(-0.0496670712318524,0.137918395416419,
-0.0613337478477096));
#44498=CARTESIAN_POINT('Ctrl Pts',(-0.00403811739418901,0.154348662490852,
-0.0639828449503602));
#44499=CARTESIAN_POINT('Ctrl Pts',(0.0505483463522294,0.145896124452282,
-0.0666319420530108));
#44500=CARTESIAN_POINT('Ctrl Pts',(0.0890656175158321,0.116431454056438,
-0.0692810391556615));
#44501=CARTESIAN_POINT('Ctrl Pts',(0.127582888679433,0.0869667836605948,
-0.071930136258312));
#44502=CARTESIAN_POINT('Ctrl Pts',(0.150030967260219,0.0364899809074799,
-0.0745792333609626));
#44503=CARTESIAN_POINT('Ctrl Pts',(0.146112043556668,-0.0118477202811764,
-0.0772283304636131));
#44504=CARTESIAN_POINT('Ctrl Pts',(0.142193119853117,-0.0601854214698328,
-0.0798774275662636));
#44505=CARTESIAN_POINT('Ctrl Pts',(0.111907193865229,-0.106384021094031,
-0.0825265246689142));
#44506=CARTESIAN_POINT('Ctrl Pts',(0.0691448976157257,-0.129258739853145,
-0.0851756217715646));
#44507=CARTESIAN_POINT('Ctrl Pts',(0.02638260136622,-0.152133458612262,
-0.0878247188742153));
#44508=CARTESIAN_POINT('Ctrl Pts',(-0.028856065144902,-0.151684296506292,
-0.0904738159768659));
#44509=CARTESIAN_POINT('Ctrl Pts',(-0.0712399745379113,-0.128116417425042,
-0.0931229130795165));
#44510=CARTESIAN_POINT('Ctrl Pts',(-0.113623883930918,-0.104548538343794,
-0.0957720101821671));
#44511=CARTESIAN_POINT('Ctrl Pts',(-0.143153036205815,-0.0578619422872685,
-0.0984211072848177));
#44512=CARTESIAN_POINT('Ctrl Pts',(-0.146285101710351,-0.00946718490431867,
-0.101070204387468));
#44513=CARTESIAN_POINT('Ctrl Pts',(-0.146487786263673,-0.0063354273567671,
-0.101241634730217));
#44514=CARTESIAN_POINT('Ctrl Pts',(-0.146579926700862,-0.00319651647499787,
-0.101413065072967));
#44515=CARTESIAN_POINT('Ctrl Pts',(-0.146564414435351,-5.66789191273343E-5,
-0.101584495415716));
#44516=CARTESIAN_POINT('Ctrl Pts',(-0.146581435366625,-3.40469869341234E-5,
-0.10871550458429));
#44517=CARTESIAN_POINT('Ctrl Pts',(-0.146587207092113,-0.00187241585713054,
-0.10861510117927));
#44518=CARTESIAN_POINT('Ctrl Pts',(-0.146555622107311,-0.00371058180105663,
-0.108514697774249));
#44519=CARTESIAN_POINT('Ctrl Pts',(-0.146486066255375,-0.00554730986340993,
-0.108414294369229));
#44520=CARTESIAN_POINT('Ctrl Pts',(-0.144650867480983,-0.0540085247729829,
-0.105765197266578));
#44521=CARTESIAN_POINT('Ctrl Pts',(-0.116382490276587,-0.101468767541441,
-0.103116100163928));
#44522=CARTESIAN_POINT('Ctrl Pts',(-0.0746446598804173,-0.126163050920102,
-0.100467003061277));
#44523=CARTESIAN_POINT('Ctrl Pts',(-0.0329068294842501,-0.150857334298762,
-0.0978179059586271));
#44524=CARTESIAN_POINT('Ctrl Pts',(0.0223004541036862,-0.152785658287626,
-0.0951688088559769));
#44525=CARTESIAN_POINT('Ctrl Pts',(0.0656596537528744,-0.131063848755951,
-0.0925197117533265));
#44526=CARTESIAN_POINT('Ctrl Pts',(0.109018853402065,-0.109342039224275,
-0.0898706146506759));
#44527=CARTESIAN_POINT('Ctrl Pts',(0.140529969112507,-0.0639700961720474,
-0.0872215175480249));
#44528=CARTESIAN_POINT('Ctrl Pts',(0.145742027776359,-0.0157549866249117,
-0.0845724204453744));
#44529=CARTESIAN_POINT('Ctrl Pts',(0.150954086440211,0.0324601229222266,
-0.0819233233427238));
#44530=CARTESIAN_POINT('Ctrl Pts',(0.129867088057477,0.0835183989642793,
-0.0792742262400732));
#44531=CARTESIAN_POINT('Ctrl Pts',(0.0921517725471056,0.114004389811336,
-0.0766251291374225));
#44532=CARTESIAN_POINT('Ctrl Pts',(0.054436457036736,0.14449038065839,-0.0739760320347719));
#44533=CARTESIAN_POINT('Ctrl Pts',(9.28243987341967E-5,0.15440408631045,
-0.0713269349321214));
#44534=CARTESIAN_POINT('Ctrl Pts',(-0.0459583001113908,0.139200118538303,
-0.0686778378294708));
#44535=CARTESIAN_POINT('Ctrl Pts',(-0.0920094246215131,0.123996150766157,
-0.0660287407268205));
#44536=CARTESIAN_POINT('Ctrl Pts',(-0.129768041003757,0.0836745095698077,
-0.0633796436241703));
#44537=CARTESIAN_POINT('Ctrl Pts',(-0.141916889037382,0.0367245704198023,
-0.0607305465215199));
#44538=CARTESIAN_POINT('Ctrl Pts',(-0.144997238974008,0.024820376566606,
-0.0600588658757764));
#44539=CARTESIAN_POINT('Ctrl Pts',(-0.1464311881288,0.012490062696057,-0.059387185230033));
#44540=CARTESIAN_POINT('Ctrl Pts',(-0.146319403921505,0.000134192518820611,
-0.0587155045842896));
#44541=CARTESIAN_POINT('Origin',(0.,0.,-3.06008671147362));
#44542=CARTESIAN_POINT('',(-0.117782368947698,0.000108066697646992,-0.0350867114736242));
#44543=CARTESIAN_POINT('',(-0.117559568560248,-6.5321138236249E-5,-0.0252132885263911));
#44544=CARTESIAN_POINT('',(-0.117775,1.13296574333067E-13,-3.06008671147362));
#44545=CARTESIAN_POINT('',(0.106356886625425,-0.0510349087439493,-0.0136500000000001));
#44546=CARTESIAN_POINT('Ctrl Pts',(-0.117782368947698,0.000108066697646985,
-0.0350867114736242));
#44547=CARTESIAN_POINT('Ctrl Pts',(-0.117498396216706,-0.0301984012316938,
-0.0330382680789872));
#44548=CARTESIAN_POINT('Ctrl Pts',(-0.0901079789233812,-0.100150743397372,
-0.0283407275816995));
#44549=CARTESIAN_POINT('Ctrl Pts',(0.0244229449298219,-0.135448756285299,
-0.0211951570904917));
#44550=CARTESIAN_POINT('Ctrl Pts',(0.0905597122481844,-0.0834873633603501,
-0.0160980299939206));
#44551=CARTESIAN_POINT('Ctrl Pts',(0.106356886625425,-0.0510349087439493,
-0.0136500000000001));
#44552=CARTESIAN_POINT('',(-0.0138313775859597,-0.116960008631475,-0.0136500000000002));
#44553=CARTESIAN_POINT('Origin',(0.,0.,-0.0136500000000002));
#44554=CARTESIAN_POINT('Ctrl Pts',(-0.117559568560248,-6.53211382362472E-5,
-0.0252132885263911));
#44555=CARTESIAN_POINT('Ctrl Pts',(-0.117588588566995,-0.0179836296355686,
-0.0240079561202446));
#44556=CARTESIAN_POINT('Ctrl Pts',(-0.105317098863147,-0.075201842880568,
-0.0201535266114477));
#44557=CARTESIAN_POINT('Ctrl Pts',(-0.0527668217477812,-0.112355607212729,
-0.0162990971026507));
#44558=CARTESIAN_POINT('Ctrl Pts',(-0.0138313775859597,-0.116960008631475,
-0.0136500000000002));
#44559=CARTESIAN_POINT('Origin',(0.,0.,-3.06008671147362));
#44560=CARTESIAN_POINT('',(-0.117947549778773,-4.5612297192055E-5,-0.0850867114736239));
#44561=CARTESIAN_POINT('',(-0.117750377839804,0.000107991280655955,-0.0752132885263904));
#44562=CARTESIAN_POINT('',(-0.117775,1.13296574333067E-13,-3.06008671147362));
#44563=CARTESIAN_POINT('Ctrl Pts',(-0.117947549778773,-4.56122971920513E-5,
-0.0850867114736239));
#44564=CARTESIAN_POINT('Ctrl Pts',(-0.11796003325722,-0.00257239308396317,
-0.0849152811308741));
#44565=CARTESIAN_POINT('Ctrl Pts',(-0.116740051627237,-0.0441330121862037,
-0.0820947536854738));
#44566=CARTESIAN_POINT('Ctrl Pts',(-0.0676751419254551,-0.12170630648443,
-0.0766251291374228));
#44567=CARTESIAN_POINT('Ctrl Pts',(0.0656846246959371,-0.122790694602604,
-0.0686778378294716));
#44568=CARTESIAN_POINT('Ctrl Pts',(0.138802320628112,-0.0112558793500066,
-0.0607305465215197));
#44569=CARTESIAN_POINT('Ctrl Pts',(0.0846071216902694,0.110607573555673,
-0.0527832552135683));
#44570=CARTESIAN_POINT('Ctrl Pts',(-0.0471780665789619,0.131014085359439,
-0.0448359639056163));
#44571=CARTESIAN_POINT('Ctrl Pts',(-0.112892038546555,0.0569824744721723,
-0.0389371159923019));
#44572=CARTESIAN_POINT('Ctrl Pts',(-0.117865636698367,0.00899466438748865,
-0.0356873651816377));
#44573=CARTESIAN_POINT('Ctrl Pts',(-0.117782368947698,0.000108066697646985,
-0.0350867114736242));
#44574=CARTESIAN_POINT('Ctrl Pts',(-0.117750377839804,0.000107991280655946,
-0.0752132885263904));
#44575=CARTESIAN_POINT('Ctrl Pts',(-0.117485542371871,-0.0291651300276833,
-0.0732358720694808));
#44576=CARTESIAN_POINT('Ctrl Pts',(-0.0916414878538697,-0.0980717922490419,
-0.0686093585099205));
#44577=CARTESIAN_POINT('Ctrl Pts',(0.0240158013170603,-0.137163045762996,
-0.0613337478477098));
#44578=CARTESIAN_POINT('Ctrl Pts',(0.128339992499329,-0.0540801177957914,
-0.0533864565397582));
#44579=CARTESIAN_POINT('Ctrl Pts',(0.114921489370477,0.0786438502502632,
-0.0454391652318065));
#44580=CARTESIAN_POINT('Ctrl Pts',(-0.0038420162804081,0.139161560048721,
-0.0374918739238548));
#44581=CARTESIAN_POINT('Ctrl Pts',(-0.101699995939352,0.0823447168505036,
-0.0307499150220496));
#44582=CARTESIAN_POINT('Ctrl Pts',(-0.117524807973858,0.0213974895334067,
-0.0266570532228951));
#44583=CARTESIAN_POINT('Ctrl Pts',(-0.117559568560248,-6.53211382362472E-5,
-0.0252132885263911));
#44584=CARTESIAN_POINT('Origin',(0.,0.,-3.06008671147362));
#44585=CARTESIAN_POINT('',(-0.117644293922143,-8.24728389195078E-5,-0.135086711473624));
#44586=CARTESIAN_POINT('',(-0.117961247354316,-2.73992748022617E-5,-0.12521328852639));
#44587=CARTESIAN_POINT('',(-0.117775,1.13296574333067E-13,-3.06008671147362));
#44588=CARTESIAN_POINT('Ctrl Pts',(-0.117644293922143,-8.24728389195242E-5,
-0.135086711473624));
#44589=CARTESIAN_POINT('Ctrl Pts',(-0.117734495770028,-0.0140816040781494,
-0.134143197080111));
#44590=CARTESIAN_POINT('Ctrl Pts',(-0.108941502454585,-0.0672763816880252,
-0.130550585583947));
#44591=CARTESIAN_POINT('Ctrl Pts',(-0.0299022661697765,-0.136007978091718,
-0.124308876985132));
#44592=CARTESIAN_POINT('Ctrl Pts',(0.0981607747731693,-0.0987763617687909,
-0.116361585677181));
#44593=CARTESIAN_POINT('Ctrl Pts',(0.136192280372371,0.0290514034709051,
-0.108414294369229));
#44594=CARTESIAN_POINT('Ctrl Pts',(0.0493101426383743,0.130233760247366,
-0.100467003061278));
#44595=CARTESIAN_POINT('Ctrl Pts',(-0.0799485994171707,0.112361477994011,
-0.092691142096076));
#44596=CARTESIAN_POINT('Ctrl Pts',(-0.117767127228718,0.0364737148214392,
-0.0875643782335247));
#44597=CARTESIAN_POINT('Ctrl Pts',(-0.117947549778773,-4.56122971920513E-5,
-0.0850867114736239));
#44598=CARTESIAN_POINT('Ctrl Pts',(-0.117961247354316,-2.73992748022543E-5,
-0.12521328852639));
#44599=CARTESIAN_POINT('Ctrl Pts',(-0.117965892143996,-0.001506824581892,
-0.125112885121367));
#44600=CARTESIAN_POINT('Ctrl Pts',(-0.11726983255438,-0.0420157259051257,
-0.122363384613694));
#44601=CARTESIAN_POINT('Ctrl Pts',(-0.0709097346571945,-0.11985045568327,
-0.116964787003371));
#44602=CARTESIAN_POINT('Ctrl Pts',(0.0623742658464559,-0.124505905450053,
-0.109017495695419));
#44603=CARTESIAN_POINT('Ctrl Pts',(0.138449871985116,-0.0149668430727117,
-0.101070204387468));
#44604=CARTESIAN_POINT('Ctrl Pts',(0.0875406563815945,0.108300429783857,
-0.093122913079516));
#44605=CARTESIAN_POINT('Ctrl Pts',(-0.0436582776930319,0.132234560631268,
-0.0851756217715646));
#44606=CARTESIAN_POINT('Ctrl Pts',(-0.112135132893251,0.0591095510259165,
-0.0792057469205228));
#44607=CARTESIAN_POINT('Ctrl Pts',(-0.117840336056494,0.0100513640863849,
-0.0758849691721313));
#44608=CARTESIAN_POINT('Ctrl Pts',(-0.117750377839804,0.000107991280655946,
-0.0752132885263904));
#44609=CARTESIAN_POINT('Origin',(0.,0.,-3.06008671147362));
#44610=CARTESIAN_POINT('',(-0.117647509884266,8.40633693049918E-5,-0.185086711473623));
#44611=CARTESIAN_POINT('',(-0.117668478068114,-9.27795444453927E-5,-0.17521328852639));
#44612=CARTESIAN_POINT('',(-0.117775,1.13296574333067E-13,-3.06008671147362));
#44613=CARTESIAN_POINT('Ctrl Pts',(-0.117647509884266,8.40633693049864E-5,
-0.185086711473623));
#44614=CARTESIAN_POINT('Ctrl Pts',(-0.117480044497517,-0.0253689009508002,
-0.183371113029347));
#44615=CARTESIAN_POINT('Ctrl Pts',(-0.096858013655478,-0.0903716449468221,
-0.17900641748242));
#44616=CARTESIAN_POINT('Ctrl Pts',(0.0103865420804345,-0.138868404314727,
-0.171992624832842));
#44617=CARTESIAN_POINT('Ctrl Pts',(0.12237839822605,-0.0664517977974861,
-0.164045333524891));
#44618=CARTESIAN_POINT('Ctrl Pts',(0.122126615970329,0.0669134043386132,
-0.156098042216939));
#44619=CARTESIAN_POINT('Ctrl Pts',(0.00986212241425144,0.138906633291134,
-0.148150750908988));
#44620=CARTESIAN_POINT('Ctrl Pts',(-0.0970456661352901,0.0900751105073112,
-0.141146973994549));
#44621=CARTESIAN_POINT('Ctrl Pts',(-0.117481236831397,0.025223634146552,
-0.136792294182761));
#44622=CARTESIAN_POINT('Ctrl Pts',(-0.117644293922143,-8.24728389195242E-5,
-0.135086711473624));
#44623=CARTESIAN_POINT('Ctrl Pts',(-0.117668478068114,-9.27795444453997E-5,
-0.17521328852639));
#44624=CARTESIAN_POINT('Ctrl Pts',(-0.117763576635394,-0.0130313762783267,
-0.174340801070604));
#44625=CARTESIAN_POINT('Ctrl Pts',(-0.109825503309218,-0.0651414645689068,
-0.170819216512168));
#44626=CARTESIAN_POINT('Ctrl Pts',(-0.0335329405968919,-0.135158632142634,
-0.16464853485108));
#44627=CARTESIAN_POINT('Ctrl Pts',(0.0954810297919763,-0.101369056556591,
-0.156701243543129));
#44628=CARTESIAN_POINT('Ctrl Pts',(0.136921232711689,0.0253946947183125,
-0.148753952235177));
#44629=CARTESIAN_POINT('Ctrl Pts',(0.0527793109988149,0.128866829226554,
-0.140806660927226));
#44630=CARTESIAN_POINT('Ctrl Pts',(-0.0780963839282828,0.114330198428394,
-0.132959773024297));
#44631=CARTESIAN_POINT('Ctrl Pts',(-0.117843341530487,0.0375271234571879,
-0.127761982224018));
#44632=CARTESIAN_POINT('Ctrl Pts',(-0.117961247354316,-2.73992748022543E-5,
-0.12521328852639));
#44633=CARTESIAN_POINT('Origin',(0.,0.,-3.06008671147362));
#44634=CARTESIAN_POINT('',(-0.117949786367931,4.31836698983784E-5,-0.235086711473623));
#44635=CARTESIAN_POINT('',(-0.117626188250658,7.19124116373773E-5,-0.22521328852639));
#44636=CARTESIAN_POINT('',(-0.117775,1.13296574333067E-13,-3.06008671147362));
#44637=CARTESIAN_POINT('Ctrl Pts',(-0.117949786367931,4.31836698983855E-5,
-0.235086711473623));
#44638=CARTESIAN_POINT('Ctrl Pts',(-0.117777175438158,-0.0366218388289575,
-0.232599028978583));
#44639=CARTESIAN_POINT('Ctrl Pts',(-0.0796904654718219,-0.112640263012373,
-0.227462249380893));
#44640=CARTESIAN_POINT('Ctrl Pts',(0.0498015954015689,-0.130046587870231,
-0.219676372680552));
#44641=CARTESIAN_POINT('Ctrl Pts',(0.136300969518302,-0.0285369869745706,
-0.2117290813726));
#44642=CARTESIAN_POINT('Ctrl Pts',(0.0977871294194325,0.099146312286434,
-0.203781790064648));
#44643=CARTESIAN_POINT('Ctrl Pts',(-0.0304156058568074,0.135894094238902,
-0.195834498756697));
#44644=CARTESIAN_POINT('Ctrl Pts',(-0.109068335787174,0.0669753266805635,
-0.189602805893022));
#44645=CARTESIAN_POINT('Ctrl Pts',(-0.117738631856529,0.0139336376235387,
-0.186020210131997));
#44646=CARTESIAN_POINT('Ctrl Pts',(-0.117647509884266,8.40633693049864E-5,
-0.185086711473623));
#44647=CARTESIAN_POINT('Ctrl Pts',(-0.117626188250658,7.19124116373634E-5,
-0.22521328852639));
#44648=CARTESIAN_POINT('Ctrl Pts',(-0.117490400621603,-0.0243383817240207,
-0.22356871701984));
#44649=CARTESIAN_POINT('Ctrl Pts',(-0.0981703407268072,-0.0882660532411596,
-0.219275048410641));
#44650=CARTESIAN_POINT('Ctrl Pts',(0.00666484966802229,-0.139096705296418,
-0.21233228269879));
#44651=CARTESIAN_POINT('Ctrl Pts',(0.12055539313165,-0.0697044532603406,
-0.204384991390839));
#44652=CARTESIAN_POINT('Ctrl Pts',(0.123874330089505,0.0636196824021741,
-0.196437700082887));
#44653=CARTESIAN_POINT('Ctrl Pts',(0.0135775806509123,0.138592795605587,
-0.188490408774936));
#44654=CARTESIAN_POINT('Ctrl Pts',(-0.0956963157972435,0.0921750501080625,
-0.181415604922769));
#44655=CARTESIAN_POINT('Ctrl Pts',(-0.117474832840424,0.0262535428260036,
-0.176989898173254));
#44656=CARTESIAN_POINT('Ctrl Pts',(-0.117668478068114,-9.27795444453997E-5,
-0.17521328852639));
#44657=CARTESIAN_POINT('Origin',(0.,0.,-3.06008671147362));
#44658=CARTESIAN_POINT('',(-0.117777663481355,-0.000108098457152765,-0.285086711473623));
#44659=CARTESIAN_POINT('',(-0.117931147509827,6.00851020906984E-5,-0.27521328852639));
#44660=CARTESIAN_POINT('',(-0.117775,1.13296574333067E-13,-3.06008671147362));
#44661=CARTESIAN_POINT('Ctrl Pts',(-0.117777663481355,-0.000108098457152784,
-0.285086711473623));
#44662=CARTESIAN_POINT('Ctrl Pts',(-0.117861059495769,-0.0091427624241447,
-0.28447604203047));
#44663=CARTESIAN_POINT('Ctrl Pts',(-0.112781650293578,-0.057277199051128,
-0.281216275484667));
#44664=CARTESIAN_POINT('Ctrl Pts',(-0.0466886511469119,-0.131196355795028,
-0.275307411836213));
#44665=CARTESIAN_POINT('Ctrl Pts',(0.0850271090185907,-0.11028465283889,
-0.267360120528261));
#44666=CARTESIAN_POINT('Ctrl Pts',(0.138757274262191,0.0117784871313546,
-0.25941282922031));
#44667=CARTESIAN_POINT('Ctrl Pts',(0.0652213392245596,0.123038574559143,
-0.251465537912358));
#44668=CARTESIAN_POINT('Ctrl Pts',(-0.0681346343844765,0.121449518390703,
-0.243518246604407));
#44669=CARTESIAN_POINT('Ctrl Pts',(-0.116816528750904,0.043834312617339,
-0.238058637791495));
#44670=CARTESIAN_POINT('Ctrl Pts',(-0.117960986320319,0.00242221324119258,
-0.235248126081234));
#44671=CARTESIAN_POINT('Ctrl Pts',(-0.117949786367931,4.31836698983855E-5,
-0.235086711473623));
#44672=CARTESIAN_POINT('Ctrl Pts',(-0.117931147509827,6.00851020906897E-5,
-0.27521328852639));
#44673=CARTESIAN_POINT('Ctrl Pts',(-0.117709465475371,-0.0355730120958269,
-0.272796632969077));
#44674=CARTESIAN_POINT('Ctrl Pts',(-0.0815010314853682,-0.110656665461582,
-0.267730880309114));
#44675=CARTESIAN_POINT('Ctrl Pts',(0.0463019631218519,-0.131333323447874,
-0.2600160305465));
#44676=CARTESIAN_POINT('Ctrl Pts',(0.135488078736147,-0.0321759872672793,
-0.252068739238548));
#44677=CARTESIAN_POINT('Ctrl Pts',(0.100406551398842,0.0964926840371405,
-0.244121447930597));
#44678=CARTESIAN_POINT('Ctrl Pts',(-0.0267663657998475,0.136659706204361,
-0.236174156622645));
#44679=CARTESIAN_POINT('Ctrl Pts',(-0.108153254503891,0.0691102072572639,
-0.229871436821243));
#44680=CARTESIAN_POINT('Ctrl Pts',(-0.117709129094809,0.0149820365199399,
-0.226217814122491));
#44681=CARTESIAN_POINT('Ctrl Pts',(-0.117626188250658,7.19124116373634E-5,
-0.22521328852639));
#44682=CARTESIAN_POINT('Origin',(0.,0.,-3.06008671147362));
#44683=CARTESIAN_POINT('',(-0.117582262041567,1.42224617900698E-5,-0.335086711473623));
#44684=CARTESIAN_POINT('',(-0.117809707131545,-0.000105358511082676,-0.32521328852639));
#44685=CARTESIAN_POINT('',(-0.117775,1.13296574333067E-13,-3.06008671147362));
#44686=CARTESIAN_POINT('Ctrl Pts',(-0.117582262041567,1.42224617900675E-5,
-0.335086711473623));
#44687=CARTESIAN_POINT('Ctrl Pts',(-0.117560166437186,-0.0205290933732839,
-0.333703957979707));
#44688=CARTESIAN_POINT('Ctrl Pts',(-0.102645223840771,-0.0804595807109724,
-0.32967210738314));
#44689=CARTESIAN_POINT('Ctrl Pts',(-0.00707457914409293,-0.139076469072788,
-0.322991159683922));
#44690=CARTESIAN_POINT('Ctrl Pts',(0.113099750076884,-0.08124506417234,
-0.315043868375971));
#44691=CARTESIAN_POINT('Ctrl Pts',(0.12954067712726,0.0511031005833377,
-0.307096577068019));
#44692=CARTESIAN_POINT('Ctrl Pts',(0.0271688291824932,0.136580264462594,
-0.299149285760068));
#44693=CARTESIAN_POINT('Ctrl Pts',(-0.0903408531884669,0.0998456806777311,
-0.291812663895269));
#44694=CARTESIAN_POINT('Ctrl Pts',(-0.117499285801941,0.0300498030574484,
-0.287125139133121));
#44695=CARTESIAN_POINT('Ctrl Pts',(-0.117777663481355,-0.000108098457152784,
-0.285086711473623));
#44696=CARTESIAN_POINT('Ctrl Pts',(-0.117809707131545,-0.000105358511082682,
-0.32521328852639));
#44697=CARTESIAN_POINT('Ctrl Pts',(-0.117883492862803,-0.00808363414246525,
-0.324673646020964));
#44698=CARTESIAN_POINT('Ctrl Pts',(-0.113504330986124,-0.055146616911953,
-0.321484906412888));
#44699=CARTESIAN_POINT('Ctrl Pts',(-0.0501844769972613,-0.129899314490461,
-0.315647069702161));
#44700=CARTESIAN_POINT('Ctrl Pts',(0.0820439419124697,-0.112521576739974,
-0.30769977839421));
#44701=CARTESIAN_POINT('Ctrl Pts',(0.139022882231082,0.00805927122877484,
-0.299752487086258));
#44702=CARTESIAN_POINT('Ctrl Pts',(0.0684921106044416,0.12124827595279,
-0.291805195778306));
#44703=CARTESIAN_POINT('Ctrl Pts',(-0.0648586022690144,0.123230172231987,
-0.283857904470355));
#44704=CARTESIAN_POINT('Ctrl Pts',(-0.116261197910494,0.0459537469292771,
-0.278327268719716));
#44705=CARTESIAN_POINT('Ctrl Pts',(-0.117952469586325,0.00348738865504856,
-0.275445730071727));
#44706=CARTESIAN_POINT('Ctrl Pts',(-0.117931147509827,6.00851020906897E-5,
-0.27521328852639));
#44707=CARTESIAN_POINT('Origin',(0.,0.,-3.06008671147362));
#44708=CARTESIAN_POINT('',(-0.117829994138202,0.000102010137211548,-0.385086711473623));
#44709=CARTESIAN_POINT('',(-0.117580749259438,-3.1419836459024E-6,-0.375213288526389));
#44710=CARTESIAN_POINT('',(-0.117775,1.13296574333067E-13,-3.06008671147362));
#44711=CARTESIAN_POINT('Ctrl Pts',(-0.117829994138202,0.000102010137211534,
-0.385086711473623));
#44712=CARTESIAN_POINT('Ctrl Pts',(-0.11753924694104,-0.0317417880642616,
-0.382931873928943));
#44713=CARTESIAN_POINT('Ctrl Pts',(-0.0877617986391311,-0.103212422463877,
-0.378127939281613));
#44714=CARTESIAN_POINT('Ctrl Pts',(0.0331346390848385,-0.135256828339786,
-0.370674907531632));
#44715=CARTESIAN_POINT('Ctrl Pts',(0.131657918533283,-0.0453707659986463,
-0.362727616223681));
#44716=CARTESIAN_POINT('Ctrl Pts',(0.109426520779767,0.086128685522627,
-0.354780324915729));
#44717=CARTESIAN_POINT('Ctrl Pts',(-0.0131692480750101,0.138632192599552,
-0.346833033607777));
#44718=CARTESIAN_POINT('Ctrl Pts',(-0.104457444059357,0.0769723455536469,
-0.340268495793742));
#44719=CARTESIAN_POINT('Ctrl Pts',(-0.117602497483033,0.0188280579172152,
-0.336353055082357));
#44720=CARTESIAN_POINT('Ctrl Pts',(-0.117582262041567,1.42224617900675E-5,
-0.335086711473623));
#44721=CARTESIAN_POINT('Ctrl Pts',(-0.117580783791559,-3.14142509273696E-6,
-0.375213288526389));
#44722=CARTESIAN_POINT('Ctrl Pts',(-0.117585410306143,-0.0194918334504725,
-0.3739015619702));
#44723=CARTESIAN_POINT('Ctrl Pts',(-0.10376360996306,-0.0783327349515231,
-0.369940738311361));
#44724=CARTESIAN_POINT('Ctrl Pts',(-0.0107955825619163,-0.138837203348852,
-0.363330817549871));
#44725=CARTESIAN_POINT('Ctrl Pts',(0.11088400591638,-0.0842439960384028,
-0.35538352624192));
#44726=CARTESIAN_POINT('Ctrl Pts',(0.130862439686628,0.0476165466602282,
-0.347436234933967));
#44727=CARTESIAN_POINT('Ctrl Pts',(0.0308157975764226,0.135803903685831,
-0.339488943626016));
#44728=CARTESIAN_POINT('Ctrl Pts',(-0.0887820097619692,0.101903565882743,
-0.33208129482349));
#44729=CARTESIAN_POINT('Ctrl Pts',(-0.11752127979595,0.0310816033003742,
-0.327322743123614));
#44730=CARTESIAN_POINT('Ctrl Pts',(-0.117809707131545,-0.000105358511082682,
-0.32521328852639));
#44731=CARTESIAN_POINT('Origin',(0.,0.,-3.06008671147362));
#44732=CARTESIAN_POINT('',(-0.117916722700972,-6.98402240337386E-5,-0.435086711473622));
#44733=CARTESIAN_POINT('',(-0.117798146306824,0.000106700477578273,-0.425213288526389));
#44734=CARTESIAN_POINT('',(-0.117775,1.13296574333067E-13,-3.06008671147362));
#44735=CARTESIAN_POINT('Ctrl Pts',(-0.117916722700972,-6.98402240337384E-5,
-0.435086711473622));
#44736=CARTESIAN_POINT('Ctrl Pts',(-0.117945481990475,-0.00416762653193182,
-0.43480888698083));
#44737=CARTESIAN_POINT('Ctrl Pts',(-0.115890583470698,-0.04730923266947,
-0.431881965385387));
#44738=CARTESIAN_POINT('Ctrl Pts',(-0.0627408721263131,-0.124321747432419,
-0.426305946687293));
#44739=CARTESIAN_POINT('Ctrl Pts',(0.0705564186542189,-0.120058759391021,
-0.418358655379342));
#44740=CARTESIAN_POINT('Ctrl Pts',(0.139140415665318,-0.0056796697353837,
-0.41041136407139));
#44741=CARTESIAN_POINT('Ctrl Pts',(0.0801069008200053,0.113908728203041,
-0.402464072763439));
#44742=CARTESIAN_POINT('Ctrl Pts',(-0.0523994674467565,0.129021741311752,
-0.394516781455487));
#44743=CARTESIAN_POINT('Ctrl Pts',(-0.113948945296141,0.0537861578315203,
-0.388724327692215));
#44744=CARTESIAN_POINT('Ctrl Pts',(-0.117896683425988,0.00740608819267113,
-0.385580971031594));
#44745=CARTESIAN_POINT('Ctrl Pts',(-0.117829994138202,0.000102010137211534,
-0.385086711473623));
#44746=CARTESIAN_POINT('Ctrl Pts',(-0.117798146306824,0.000106700477578266,
-0.425213288526389));
#44747=CARTESIAN_POINT('Ctrl Pts',(-0.117512496286999,-0.030708896715437,
-0.423129477919436));
#44748=CARTESIAN_POINT('Ctrl Pts',(-0.0893501311828865,-0.101161866296878,
-0.418396570209834));
#44749=CARTESIAN_POINT('Ctrl Pts',(0.0295014860686701,-0.136095466332724,
-0.41101456539758));
#44750=CARTESIAN_POINT('Ctrl Pts',(0.130395995936294,-0.0488794218497269,
-0.403067274089629));
#44751=CARTESIAN_POINT('Ctrl Pts',(0.111693245167184,0.083168098575145,
-0.395119982781677));
#44752=CARTESIAN_POINT('Ctrl Pts',(-0.00945288246871811,0.138935080701795,
-0.387172691473725));
#44753=CARTESIAN_POINT('Ctrl Pts',(-0.103364419861196,0.0791009627546925,
-0.380537126721963));
#44754=CARTESIAN_POINT('Ctrl Pts',(-0.117576066829546,0.0198665506085378,
-0.376550659072851));
#44755=CARTESIAN_POINT('Ctrl Pts',(-0.117580783791559,-3.14142509273696E-6,
-0.375213288526389));
#44756=CARTESIAN_POINT('Origin',(0.,0.,-3.06008671147362));
#44757=CARTESIAN_POINT('',(-0.117614497320444,-6.31649834024115E-5,-0.485086711473622));
#44758=CARTESIAN_POINT('',(-0.117938472244188,-5.41950633561744E-5,-0.475213288526389));
#44759=CARTESIAN_POINT('',(-0.117775,1.13296574333067E-13,-3.06008671147362));
#44760=CARTESIAN_POINT('Ctrl Pts',(-0.117614497320444,-6.31649834024247E-5,
-0.485086711473622));
#44761=CARTESIAN_POINT('Ctrl Pts',(-0.117690187679668,-0.0156507863039807,
-0.484036802930066));
#44762=CARTESIAN_POINT('Ctrl Pts',(-0.107549344443015,-0.0704740980699968,
-0.48033779728386));
#44763=CARTESIAN_POINT('Ctrl Pts',(-0.0244244560972015,-0.137097628951694,
-0.473989694535004));
#44764=CARTESIAN_POINT('Ctrl Pts',(0.102042666874295,-0.0947607938812361,
-0.466042403227051));
#44765=CARTESIAN_POINT('Ctrl Pts',(0.134917779304342,0.0344892265411343,
-0.4580951119191));
#44766=CARTESIAN_POINT('Ctrl Pts',(0.0440483189035268,0.132106243310428,
-0.450147820611148));
#44767=CARTESIAN_POINT('Ctrl Pts',(-0.0826326171253195,0.10938061617266,
-0.442478353795989));
#44768=CARTESIAN_POINT('Ctrl Pts',(-0.117671257966059,0.0349053642127825,
-0.43745798408348));
#44769=CARTESIAN_POINT('Ctrl Pts',(-0.117916722700972,-6.98402240337384E-5,
-0.435086711473622));
#44770=CARTESIAN_POINT('Ctrl Pts',(-0.117938472244188,-5.41950633561714E-5,
-0.475213288526389));
#44771=CARTESIAN_POINT('Ctrl Pts',(-0.117955888778364,-0.00310288257415361,
-0.475006490971324));
#44772=CARTESIAN_POINT('Ctrl Pts',(-0.116465154288894,-0.0451882515470556,
-0.472150596313608));
#44773=CARTESIAN_POINT('Ctrl Pts',(-0.0660468875011581,-0.122597399189343,
-0.466645604553241));
#44774=CARTESIAN_POINT('Ctrl Pts',(0.0673167536278285,-0.121904751005003,
-0.45869831324529));
#44775=CARTESIAN_POINT('Ctrl Pts',(0.138938473380797,-0.00940288525907187,
-0.450751021937338));
#44776=CARTESIAN_POINT('Ctrl Pts',(0.0831278997256812,0.111723166459686,
-0.442803730629387));
#44777=CARTESIAN_POINT('Ctrl Pts',(-0.0489263424431069,0.1303783979489,
-0.434856439321435));
#44778=CARTESIAN_POINT('Ctrl Pts',(-0.113247210086591,0.0559156688588903,
-0.428992958620436));
#44779=CARTESIAN_POINT('Ctrl Pts',(-0.117875636121955,0.00846621304170956,
-0.425778575022087));
#44780=CARTESIAN_POINT('Ctrl Pts',(-0.117798146306824,0.000106700477578266,
-0.425213288526389));
#44781=CARTESIAN_POINT('Origin',(0.,0.,-3.06008671147362));
#44782=CARTESIAN_POINT('',(-0.117685468281101,9.81124517920193E-5,-0.535086711473622));
#44783=CARTESIAN_POINT('',(-0.117633476200538,-7.65294932578153E-5,-0.525213288526388));
#44784=CARTESIAN_POINT('',(-0.117775,1.13296574333067E-13,-3.06008671147362));
#44785=CARTESIAN_POINT('Ctrl Pts',(-0.117685468281101,9.81124517920162E-5,
-0.535086711473622));
#44786=CARTESIAN_POINT('Ctrl Pts',(-0.117473376022059,-0.0269113827363188,
-0.533264718879303));
#44787=CARTESIAN_POINT('Ctrl Pts',(-0.094811321954978,-0.0935130246987491,
-0.528793629182333));
#44788=CARTESIAN_POINT('Ctrl Pts',(0.0159466578264506,-0.13834022561781,
-0.521673442382713));
#44789=CARTESIAN_POINT('Ctrl Pts',(0.124944615327587,-0.0614911133454406,
-0.513726151074761));
#44790=CARTESIAN_POINT('Ctrl Pts',(0.119345237096187,0.071756730013814,
-0.50577885976681));
#44791=CARTESIAN_POINT('Ctrl Pts',(0.00428418924635087,0.139190371945483,
-0.497831568458857));
#44792=CARTESIAN_POINT('Ctrl Pts',(-0.0989865471327881,0.0869175656192404,
-0.490934185694462));
#44793=CARTESIAN_POINT('Ctrl Pts',(-0.117499208081921,0.0236794227232818,
-0.486685900032717));
#44794=CARTESIAN_POINT('Ctrl Pts',(-0.117614497320444,-6.31649834024247E-5,
-0.485086711473622));
#44795=CARTESIAN_POINT('Ctrl Pts',(-0.117633476200538,-7.65294932578171E-5,
-0.525213288526388));
#44796=CARTESIAN_POINT('Ctrl Pts',(-0.117719816016294,-0.0146037641429175,
-0.52423440692056));
#44797=CARTESIAN_POINT('Ctrl Pts',(-0.108487849042328,-0.0683394445861028,
-0.52060642821208));
#44798=CARTESIAN_POINT('Ctrl Pts',(-0.0280862598533812,-0.136394558703894,
-0.514329352400952));
#44799=CARTESIAN_POINT('Ctrl Pts',(0.0994690254013135,-0.0974588457878242,
-0.506382061092999));
#44800=CARTESIAN_POINT('Ctrl Pts',(0.135792805648636,0.0308646654064759,
-0.498434769785048));
#44801=CARTESIAN_POINT('Ctrl Pts',(0.0475694519664141,0.130879566305045,
-0.490487478477097));
#44802=CARTESIAN_POINT('Ctrl Pts',(-0.0808529189036142,0.111374779294211,
-0.48274698472421));
#44803=CARTESIAN_POINT('Ctrl Pts',(-0.117732781255603,0.0359511055119116,
-0.477655588073974));
#44804=CARTESIAN_POINT('Ctrl Pts',(-0.117938472244188,-5.41950633561714E-5,
-0.475213288526389));
#44805=CARTESIAN_POINT('Origin',(0.,0.,-3.06008671147362));
#44806=CARTESIAN_POINT('',(-0.117966591322209,1.51587796647229E-5,-0.585086711473623));
#44807=CARTESIAN_POINT('',(-0.117659387014888,8.93238483695505E-5,-0.575213288526388));
#44808=CARTESIAN_POINT('',(-0.117775,1.13296574333067E-13,-3.06008671147362));
#44809=CARTESIAN_POINT('Ctrl Pts',(-0.117966591322209,1.51587796647183E-5,
-0.585086711473623));
#44810=CARTESIAN_POINT('Ctrl Pts',(-0.117897493436053,-0.0382034176156981,
-0.58249263482854));
#44811=CARTESIAN_POINT('Ctrl Pts',(-0.076887247580097,-0.115578456916855,
-0.577249461080806));
#44812=CARTESIAN_POINT('Ctrl Pts',(0.0549762653464128,-0.127945004468253,
-0.569357190230422));
#44813=CARTESIAN_POINT('Ctrl Pts',(0.137335646484491,-0.02304851675287,
-0.561409898922471));
#44814=CARTESIAN_POINT('Ctrl Pts',(0.0937328231132788,0.102987726409681,
-0.553462607614519));
#44815=CARTESIAN_POINT('Ctrl Pts',(-0.0358403461692648,0.134565164534837,
-0.545515316306567));
#44816=CARTESIAN_POINT('Ctrl Pts',(-0.11037166930448,0.0637774950500043,
-0.539390017592935));
#44817=CARTESIAN_POINT('Ctrl Pts',(-0.117781748839092,0.0123592354154572,
-0.535913815981954));
#44818=CARTESIAN_POINT('Ctrl Pts',(-0.117685468281101,9.81124517920162E-5,
-0.535086711473622));
#44819=CARTESIAN_POINT('Ctrl Pts',(-0.117659387014888,8.93238483695418E-5,
-0.575213288526388));
#44820=CARTESIAN_POINT('Ctrl Pts',(-0.117476584431924,-0.0258817614303258,
-0.573462322869796));
#44821=CARTESIAN_POINT('Ctrl Pts',(-0.0961884985075474,-0.0914176792266589,
-0.569062260110554));
#44822=CARTESIAN_POINT('Ctrl Pts',(0.0122371135094518,-0.13871757887715,
-0.562013100248661));
#44823=CARTESIAN_POINT('Ctrl Pts',(0.123253503998567,-0.0648142529746122,
-0.554065808940709));
#44824=CARTESIAN_POINT('Ctrl Pts',(0.121223620817521,0.0685357380676061,
-0.546118517632758));
#44825=CARTESIAN_POINT('Ctrl Pts',(0.00800924251344417,0.139025773405302,
-0.538171226324806));
#44826=CARTESIAN_POINT('Ctrl Pts',(-0.0977014684982498,0.0890269837912308,
-0.531202816622683));
#44827=CARTESIAN_POINT('Ctrl Pts',(-0.117486158999552,0.0247105461789745,
-0.52688350402321));
#44828=CARTESIAN_POINT('Ctrl Pts',(-0.117633476200538,-7.65294932578171E-5,
-0.525213288526388));
#44829=CARTESIAN_POINT('Origin',(0.,0.,-3.06008671147362));
#44830=CARTESIAN_POINT('',(-0.117730596314636,-0.000106536436396233,-0.635086711473622));
#44831=CARTESIAN_POINT('',(-0.117956987195077,3.41556508710135E-5,-0.625213288526389));
#44832=CARTESIAN_POINT('',(-0.117775,1.13296574333067E-13,-3.06008671147362));
#44833=CARTESIAN_POINT('Ctrl Pts',(-0.117730596314636,-0.000106536436396257,
-0.635086711473622));
#44834=CARTESIAN_POINT('Ctrl Pts',(-0.117823857820801,-0.0107260812779556,
-0.634369647880426));
#44835=CARTESIAN_POINT('Ctrl Pts',(-0.111636663996842,-0.0604713644574023,
-0.63100348718458));
#44836=CARTESIAN_POINT('Ctrl Pts',(-0.0413902711963712,-0.13296300000418,
-0.624988229386083));
#44837=CARTESIAN_POINT('Ctrl Pts',(0.0893810158703018,-0.106786459449753,
-0.617040938078132));
#44838=CARTESIAN_POINT('Ctrl Pts',(0.138173369655621,0.0173330273706489,
-0.60909364677018));
#44839=CARTESIAN_POINT('Ctrl Pts',(0.0602351717464476,0.125554920271953,
-0.60114635546223));
#44840=CARTESIAN_POINT('Ctrl Pts',(-0.072949826366452,0.118619714857712,
-0.593199064154276));
#44841=CARTESIAN_POINT('Ctrl Pts',(-0.117593007644085,0.0406641950725845,
-0.587845849491409));
#44842=CARTESIAN_POINT('Ctrl Pts',(-0.117968056890823,0.000825776139351177,
-0.58514173193119));
#44843=CARTESIAN_POINT('Ctrl Pts',(-0.117966591322209,1.51587796647183E-5,
-0.585086711473623));
#44844=CARTESIAN_POINT('Ctrl Pts',(-0.117956987195077,3.41556508710156E-5,
-0.625213288526388));
#44845=CARTESIAN_POINT('Ctrl Pts',(-0.117814604554168,-0.037146083313863,
-0.622690238819033));
#44846=CARTESIAN_POINT('Ctrl Pts',(-0.0787707968119144,-0.113621523240544,
-0.617518092009027));
#44847=CARTESIAN_POINT('Ctrl Pts',(0.0515310444452701,-0.129371036538173,
-0.609696848096371));
#44848=CARTESIAN_POINT('Ctrl Pts',(0.136669329383979,-0.0267171862724199,
-0.601749556788419));
#44849=CARTESIAN_POINT('Ctrl Pts',(0.0964565459097508,0.100441268349926,
-0.593802265480467));
#44850=CARTESIAN_POINT('Ctrl Pts',(-0.0322247413590565,0.135476491248201,
-0.585854974172516));
#44851=CARTESIAN_POINT('Ctrl Pts',(-0.109510475119334,0.065912251287834,
-0.579658648521156));
#44852=CARTESIAN_POINT('Ctrl Pts',(-0.117753152844938,0.0134108006513239,
-0.576111419972447));
#44853=CARTESIAN_POINT('Ctrl Pts',(-0.117659387014888,8.93238483695418E-5,
-0.575213288526388));
#44854=CARTESIAN_POINT('Origin',(0.,0.,-3.06008671147362));
#44855=CARTESIAN_POINT('',(-0.117593034504333,3.94353800751308E-5,-0.685086711473621));
#44856=CARTESIAN_POINT('',(-0.1177617944348,-0.000108325507588214,-0.675213288526388));
#44857=CARTESIAN_POINT('',(-0.117775,1.13296574333067E-13,-3.06008671147362));
#44858=CARTESIAN_POINT('Ctrl Pts',(-0.117593034504333,3.94353800751042E-5,
-0.685086711473621));
#44859=CARTESIAN_POINT('Ctrl Pts',(-0.117526714862022,-0.0220795022350645,
-0.683597563829663));
#44860=CARTESIAN_POINT('Ctrl Pts',(-0.100894498114864,-0.0836391338586082,
-0.679459319083053));
#44861=CARTESIAN_POINT('Ctrl Pts',(-0.00149207632259066,-0.13924829488388,
-0.672671977233793));
#44862=CARTESIAN_POINT('Ctrl Pts',(0.116266623106448,-0.0766445449542468,
-0.664724685925842));
#44863=CARTESIAN_POINT('Ctrl Pts',(0.12738731170417,0.0562564372903673,
-0.65677739461789));
#44864=CARTESIAN_POINT('Ctrl Pts',(0.0216702599226566,0.13755985517114,
-0.648830103309939));
#44865=CARTESIAN_POINT('Ctrl Pts',(-0.0925905262321655,0.0967434292388231,
-0.641599875595182));
#44866=CARTESIAN_POINT('Ctrl Pts',(-0.117479315456474,0.0285064299500534,
-0.637018744983077));
#44867=CARTESIAN_POINT('Ctrl Pts',(-0.117730596314636,-0.000106536436396257,
-0.635086711473622));
#44868=CARTESIAN_POINT('Ctrl Pts',(-0.1177617944348,-0.00010832550758821,
-0.675213288526388));
#44869=CARTESIAN_POINT('Ctrl Pts',(-0.117849137564383,-0.00966952653099531,
-0.67456725187092));
#44870=CARTESIAN_POINT('Ctrl Pts',(-0.112409423629664,-0.0583386690669818,
-0.671272118112801));
#44871=CARTESIAN_POINT('Ctrl Pts',(-0.0449352953335994,-0.131807180646063,
-0.665327887252032));
#44872=CARTESIAN_POINT('Ctrl Pts',(0.086489946256864,-0.109141205935553,
-0.657380595944081));
#44873=CARTESIAN_POINT('Ctrl Pts',(0.138587900451223,0.0136274533609135,
-0.649433304636128));
#44874=CARTESIAN_POINT('Ctrl Pts',(0.0635751014943803,0.123897215895116,
-0.641486013328178));
#44875=CARTESIAN_POINT('Ctrl Pts',(-0.0697478313652302,0.120530301818377,
-0.633538722020224));
#44876=CARTESIAN_POINT('Ctrl Pts',(-0.117081947198759,0.0427798822024834,
-0.628114480419629));
#44877=CARTESIAN_POINT('Ctrl Pts',(-0.1179641003966,0.00189161896770185,
-0.625339335921684));
#44878=CARTESIAN_POINT('Ctrl Pts',(-0.117956987195077,3.41556508710156E-5,
-0.625213288526388));
#44879=CARTESIAN_POINT('Origin',(0.,0.,-3.06008671147362));
#44880=CARTESIAN_POINT('',(-0.117875484466013,8.93978020177876E-5,-0.735086711473622));
#44881=CARTESIAN_POINT('',(-0.117584714802368,2.27631449018287E-5,-0.725213288526388));
#44882=CARTESIAN_POINT('',(-0.117775,1.13296574333067E-13,-3.06008671147362));
#44883=CARTESIAN_POINT('Ctrl Pts',(-0.117875484466013,8.93978020177879E-5,
-0.735086711473622));
#44884=CARTESIAN_POINT('Ctrl Pts',(-0.117594165739836,-0.0332932738978478,
-0.732825479778899));
#44885=CARTESIAN_POINT('Ctrl Pts',(-0.0852952950029288,-0.106260690388895,
-0.727915150981525));
#44886=CARTESIAN_POINT('Ctrl Pts',(0.0385316388930217,-0.133819380973154,
-0.720355725081504));
#44887=CARTESIAN_POINT('Ctrl Pts',(0.13337134577548,-0.0400549378461348,
-0.712408433773551));
#44888=CARTESIAN_POINT('Ctrl Pts',(0.105884845571219,0.0904472962458246,
-0.7044611424656));
#44889=CARTESIAN_POINT('Ctrl Pts',(-0.018717654110887,0.137992620615763,
-0.696513851157648));
#44890=CARTESIAN_POINT('Ctrl Pts',(-0.106021654180243,0.0737796804798823,
-0.690055707493655));
#44891=CARTESIAN_POINT('Ctrl Pts',(-0.117644693205544,0.0172686535960106,
-0.686246660932313));
#44892=CARTESIAN_POINT('Ctrl Pts',(-0.117593034504333,3.94353800751042E-5,
-0.685086711473621));
#44893=CARTESIAN_POINT('Ctrl Pts',(-0.117584714802368,2.27631449018183E-5,
-0.725213288526388));
#44894=CARTESIAN_POINT('Ctrl Pts',(-0.11754840398394,-0.0210449003143397,
-0.723795167820157));
#44895=CARTESIAN_POINT('Ctrl Pts',(-0.102073372171732,-0.0815174398122862,
-0.719727950011274));
#44896=CARTESIAN_POINT('Ctrl Pts',(-0.00521968128764912,-0.139158429726111,
-0.713011635099741));
#44897=CARTESIAN_POINT('Ctrl Pts',(0.114172914890457,-0.0797299137212506,
-0.705064343791791));
#44898=CARTESIAN_POINT('Ctrl Pts',(0.128847818153508,0.0528256887665676,
-0.697117052483838));
#44899=CARTESIAN_POINT('Ctrl Pts',(0.0253454263276182,0.136930358214871,
-0.689169761175887));
#44900=CARTESIAN_POINT('Ctrl Pts',(-0.0910999775854965,0.0988169360777528,
-0.681868506523403));
#44901=CARTESIAN_POINT('Ctrl Pts',(-0.117490983844226,0.0295365304544467,
-0.67721634897357));
#44902=CARTESIAN_POINT('Ctrl Pts',(-0.1177617944348,-0.00010832550758821,
-0.675213288526388));
#44903=CARTESIAN_POINT('Origin',(0.,0.,-3.06008671147362));
#44904=CARTESIAN_POINT('',(-0.117876965213514,-8.8851257191466E-5,-0.785086711473622));
#44905=CARTESIAN_POINT('',(-0.117845523526878,9.85473074824224E-5,-0.775213288526388));
#44906=CARTESIAN_POINT('',(-0.117775,1.13296574333067E-13,-3.06008671147362));
#44907=CARTESIAN_POINT('Ctrl Pts',(-0.117876965213514,-8.88512571914774E-5,
-0.785086711473622));
#44908=CARTESIAN_POINT('Ctrl Pts',(-0.117924564182101,-0.00576090399454924,
-0.784702492830786));
#44909=CARTESIAN_POINT('Ctrl Pts',(-0.114972566077973,-0.0504906643974819,
-0.7816691770853));
#44910=CARTESIAN_POINT('Ctrl Pts',(-0.0577052458335282,-0.126737597117481,
-0.775986764237163));
#44911=CARTESIAN_POINT('Ctrl Pts',(0.0753138949338155,-0.117132963548775,
-0.768039472929213));
#44912=CARTESIAN_POINT('Ctrl Pts',(0.139256255718067,-9.57246296715326E-5,
-0.760092181621259));
#44913=CARTESIAN_POINT('Ctrl Pts',(0.075474857879039,0.117029311490581,
-0.75214489031331));
#44914=CARTESIAN_POINT('Ctrl Pts',(-0.0575309527532313,0.126816810380666,
-0.744197599005357));
#44915=CARTESIAN_POINT('Ctrl Pts',(-0.11493986229245,0.0505997987675953,
-0.738511539392129));
#44916=CARTESIAN_POINT('Ctrl Pts',(-0.117923738611195,0.00581547337703481,
-0.73547457688155));
#44917=CARTESIAN_POINT('Ctrl Pts',(-0.117875484466013,8.93978020177879E-5,
-0.735086711473622));
#44918=CARTESIAN_POINT('Ctrl Pts',(-0.117845523526878,9.8547307482425E-5,
-0.775213288526388));
#44919=CARTESIAN_POINT('Ctrl Pts',(-0.117555464158849,-0.0322568831287426,
-0.773023083769393));
#44920=CARTESIAN_POINT('Ctrl Pts',(-0.086953565764276,-0.10422895270096,
-0.768183781909747));
#44921=CARTESIAN_POINT('Ctrl Pts',(0.0349350364218175,-0.134803029887269,
-0.760695382947452));
#44922=CARTESIAN_POINT('Ctrl Pts',(0.132251131348421,-0.0436113734436843,
-0.752748091639499));
#44923=CARTESIAN_POINT('Ctrl Pts',(0.108268463135797,0.087579983596677,
-0.744800800331548));
#44924=CARTESIAN_POINT('Ctrl Pts',(-0.0150164229970535,0.138444287267318,
-0.736853509023596));
#44925=CARTESIAN_POINT('Ctrl Pts',(-0.10498705715791,0.075911527904859,
-0.730324338421876));
#44926=CARTESIAN_POINT('Ctrl Pts',(-0.117616233812155,0.0183102025229871,
-0.726444264922807));
#44927=CARTESIAN_POINT('Ctrl Pts',(-0.117584714802368,2.27631449018183E-5,
-0.725213288526388));
#44928=CARTESIAN_POINT('Origin',(0.,0.,-3.06008671147362));
#44929=CARTESIAN_POINT('',(-0.117593581734726,-4.02682066843004E-5,-0.835086711473621));
#44930=CARTESIAN_POINT('',(-0.117904332456761,-7.67924259059416E-5,-0.825213288526388));
#44931=CARTESIAN_POINT('',(-0.117775,1.13296574333067E-13,-3.06008671147362));
#44932=CARTESIAN_POINT('Ctrl Pts',(-0.117593581734727,-4.02682066843133E-5,
-0.83508671147362));
#44933=CARTESIAN_POINT('Ctrl Pts',(-0.117646179449728,-0.0172151199308131,
-0.833930408780022));
#44934=CARTESIAN_POINT('Ctrl Pts',(-0.106073737451821,-0.0736701797484393,
-0.830125008983773));
#44935=CARTESIAN_POINT('Ctrl Pts',(-0.0189073483484057,-0.137966757221631,
-0.823670512084875));
#44936=CARTESIAN_POINT('Ctrl Pts',(0.105760398778781,-0.0905927810036414,
-0.81572322077692));
#44937=CARTESIAN_POINT('Ctrl Pts',(0.133426287168139,0.0398715413841222,
-0.807775929468972));
#44938=CARTESIAN_POINT('Ctrl Pts',(0.038715577045716,0.133766281303764,
-0.799828638161018));
#44939=CARTESIAN_POINT('Ctrl Pts',(-0.0852088813915643,0.106364641204736,
-0.792265565495903));
#44940=CARTESIAN_POINT('Ctrl Pts',(-0.117596380497826,0.0333465645075948,
-0.787351589933437));
#44941=CARTESIAN_POINT('Ctrl Pts',(-0.117876965213514,-8.88512571914774E-5,
-0.785086711473622));
#44942=CARTESIAN_POINT('Ctrl Pts',(-0.117904332456761,-7.67924259059459E-5,
-0.825213288526388));
#44943=CARTESIAN_POINT('Ctrl Pts',(-0.117939220517964,-0.00469750316242473,
-0.82490009682128));
#44944=CARTESIAN_POINT('Ctrl Pts',(-0.115593117736479,-0.0483662331465746,
-0.821937808013521));
#44945=CARTESIAN_POINT('Ctrl Pts',(-0.0610777466931965,-0.1251472033066,
-0.816326422103112));
#44946=CARTESIAN_POINT('Ctrl Pts',(0.0721508577441712,-0.119107377451451,
-0.808379130795161));
#44947=CARTESIAN_POINT('Ctrl Pts',(0.139203772684067,-0.00382404329272468,
-0.800431839487209));
#44948=CARTESIAN_POINT('Ctrl Pts',(0.0785810656558809,0.114966646280423,
-0.792484548179258));
#44949=CARTESIAN_POINT('Ctrl Pts',(-0.0541150215622158,0.12831164435819,
-0.784537256871306));
#44950=CARTESIAN_POINT('Ctrl Pts',(-0.114286285428402,0.0527264646981619,
-0.778780170320349));
#44951=CARTESIAN_POINT('Ctrl Pts',(-0.117906296851084,0.00687766662048267,
-0.775672180872043));
#44952=CARTESIAN_POINT('Ctrl Pts',(-0.117845523526878,9.8547307482425E-5,
-0.775213288526388));
#44953=CARTESIAN_POINT('Origin',(0.,0.,-3.06008671147362));
#44954=CARTESIAN_POINT('',(-0.117729028952017,0.000106365187095507,-0.885086711473621));
#44955=CARTESIAN_POINT('',(-0.117606504447261,-5.5889115292404E-5,-0.875213288526388));
#44956=CARTESIAN_POINT('',(-0.117775,1.13296574333067E-13,-3.06008671147362));
#44957=CARTESIAN_POINT('Ctrl Pts',(-0.117729028952017,0.000106365187095494,
-0.885086711473621));
#44958=CARTESIAN_POINT('Ctrl Pts',(-0.117478889294716,-0.0284535591076875,
-0.883158324729259));
#44959=CARTESIAN_POINT('Ctrl Pts',(-0.0926658391403091,-0.0966367106808196,
-0.878580840882248));
#44960=CARTESIAN_POINT('Ctrl Pts',(0.0214811224820551,-0.137589517394064,
-0.871354259932582));
#44961=CARTESIAN_POINT('Ctrl Pts',(0.127309850102664,-0.0564315158989901,
-0.863406968624633));
#44962=CARTESIAN_POINT('Ctrl Pts',(0.116371883968419,0.0764846294458023,
-0.855459677316679));
#44963=CARTESIAN_POINT('Ctrl Pts',(-0.0013006366881828,0.139250214592387,
-0.847512386008729));
#44964=CARTESIAN_POINT('Ctrl Pts',(-0.100832864752058,0.0837479595872449,
-0.840721397394375));
#44965=CARTESIAN_POINT('Ctrl Pts',(-0.117525677737513,0.0221325787234608,
-0.836579505882672));
#44966=CARTESIAN_POINT('Ctrl Pts',(-0.117593581734727,-4.02682066843133E-5,
-0.83508671147362));
#44967=CARTESIAN_POINT('Ctrl Pts',(-0.117606504447261,-5.58891152924006E-5,
-0.875213288526387));
#44968=CARTESIAN_POINT('Ctrl Pts',(-0.117675456234588,-0.0161713341894999,
-0.874128012770516));
#44969=CARTESIAN_POINT('Ctrl Pts',(-0.107068193774824,-0.0715367874318198,
-0.870393639911994));
#44970=CARTESIAN_POINT('Ctrl Pts',(-0.0225943993144704,-0.137411086729565,
-0.864010169950823));
#44971=CARTESIAN_POINT('Ctrl Pts',(0.103297016147289,-0.0933918630912153,
-0.856062878642869));
#44972=CARTESIAN_POINT('Ctrl Pts',(0.134445950642072,0.0362849830168238,
-0.848115587334919));
#44973=CARTESIAN_POINT('Ctrl Pts',(0.0422830665105441,0.132681784443256,
-0.840168296026967));
#44974=CARTESIAN_POINT('Ctrl Pts',(-0.0835008827885007,0.108381751794679,
-0.832534196424123));
#44975=CARTESIAN_POINT('Ctrl Pts',(-0.117644123743871,0.0343862631847281,
-0.827549193923931));
#44976=CARTESIAN_POINT('Ctrl Pts',(-0.117904332456761,-7.67924259059459E-5,
-0.825213288526388));
#44977=CARTESIAN_POINT('Origin',(0.,0.,-3.06008671147362));
#44978=CARTESIAN_POINT('',(-0.117966893777284,-1.41613286548E-5,-0.935086711473621));
#44979=CARTESIAN_POINT('',(-0.117699425459372,0.000101537840546506,-0.925213288526387));
#44980=CARTESIAN_POINT('',(-0.117775,1.13296574333067E-13,-3.06008671147362));
#44981=CARTESIAN_POINT('Ctrl Pts',(-0.117966893777284,-1.41613286548282E-5,
-0.935086711473621));
#44982=CARTESIAN_POINT('Ctrl Pts',(-0.11796817649413,-0.000771045615368247,
-0.935035337781146));
#44983=CARTESIAN_POINT('Ctrl Pts',(-0.117618462361427,-0.0405556373780832,
-0.932334866986021));
#44984=CARTESIAN_POINT('Ctrl Pts',(-0.0731128355279682,-0.118519311510323,
-0.926985299088244));
#44985=CARTESIAN_POINT('Ctrl Pts',(0.0600625022165961,-0.125637612788934,
-0.919038007780293));
#44986=CARTESIAN_POINT('Ctrl Pts',(0.138149409672222,-0.0175229714100354,
-0.911090716472342));
#44987=CARTESIAN_POINT('Ctrl Pts',(0.0895277411724023,0.106663477724982,
-0.903143425164389));
#44988=CARTESIAN_POINT('Ctrl Pts',(-0.0412074348652185,0.133019777595849,
-0.895196133856439));
#44989=CARTESIAN_POINT('Ctrl Pts',(-0.111596070039508,0.0605808954844544,
-0.889177229292848));
#44990=CARTESIAN_POINT('Ctrl Pts',(-0.117822515511475,0.0107802786701471,
-0.885807421831909));
#44991=CARTESIAN_POINT('Ctrl Pts',(-0.117729028952017,0.000106365187095494,
-0.885086711473621));
#44992=CARTESIAN_POINT('Ctrl Pts',(-0.117699425459372,0.000101537840546503,
-0.925213288526387));
#44993=CARTESIAN_POINT('Ctrl Pts',(-0.117473768977369,-0.0274239955520595,
-0.923355928719752));
#44994=CARTESIAN_POINT('Ctrl Pts',(-0.0941091841536456,-0.0945534961756978,
-0.918849471810467));
#44995=CARTESIAN_POINT('Ctrl Pts',(0.017789693141843,-0.1381153157854,-0.911693917798532));
#44996=CARTESIAN_POINT('Ctrl Pts',(0.125753353137608,-0.0598197944766599,
-0.90374662649058));
#44997=CARTESIAN_POINT('Ctrl Pts',(0.118377915156088,0.0733415492056153,
-0.895799335182628));
#44998=CARTESIAN_POINT('Ctrl Pts',(0.00242802079729554,0.139235118959227,
-0.887852043874677));
#44999=CARTESIAN_POINT('Ctrl Pts',(-0.0996106832345008,0.0858651502554784,
-0.880990028322597));
#45000=CARTESIAN_POINT('Ctrl Pts',(-0.117507148798398,0.0231655611783769,
-0.876777109873167));
#45001=CARTESIAN_POINT('Ctrl Pts',(-0.117606504447261,-5.58891152924006E-5,
-0.875213288526387));
#45002=CARTESIAN_POINT('Origin',(0.,0.,-3.06008671147362));
#45003=CARTESIAN_POINT('',(-0.117686879986589,-9.84958757579055E-5,-0.985086711473621));
#45004=CARTESIAN_POINT('',(-0.117968676352971,5.43384420481955E-6,-0.975213288526387));
#45005=CARTESIAN_POINT('',(-0.117775,1.13296574333067E-13,-3.06008671147362));
#45006=CARTESIAN_POINT('Ctrl Pts',(-0.117686879986589,-9.84958757579094E-5,
-0.985086711473621));
#45007=CARTESIAN_POINT('Ctrl Pts',(-0.117783191571813,-0.0123051889181925,
-0.984263253730382));
#45008=CARTESIAN_POINT('Ctrl Pts',(-0.11041493107276,-0.0636679012646631,
-0.980790698884494));
#45009=CARTESIAN_POINT('Ctrl Pts',(-0.0360253121667897,-0.134515764143485,
-0.974669046935953));
#45010=CARTESIAN_POINT('Ctrl Pts',(0.0935911472513838,-0.103116492744809,
-0.966721755628004));
#45011=CARTESIAN_POINT('Ctrl Pts',(0.13736720374351,0.0228596862513367,
-0.958774464320049));
#45012=CARTESIAN_POINT('Ctrl Pts',(0.0551521118795285,0.127869302317047,
-0.950827173012101));
#45013=CARTESIAN_POINT('Ctrl Pts',(-0.0767892156275477,0.115678421683065,
-0.942931255396621));
#45014=CARTESIAN_POINT('Ctrl Pts',(-0.117902032884089,0.038257879003206,
-0.937684434883797));
#45015=CARTESIAN_POINT('Ctrl Pts',(-0.117966893777284,-1.41613286548282E-5,
-0.935086711473621));
#45016=CARTESIAN_POINT('Ctrl Pts',(-0.117968676352971,5.43384420481787E-6,
-0.975213288526387));
#45017=CARTESIAN_POINT('Ctrl Pts',(-0.117942707376789,-0.0387323630877177,
-0.972583844668988));
#45018=CARTESIAN_POINT('Ctrl Pts',(-0.07593103584133,-0.116545765660636,
-0.967305303708942));
#45019=CARTESIAN_POINT('Ctrl Pts',(0.0566772345635106,-0.127200647477969,
-0.959377665646241));
#45020=CARTESIAN_POINT('Ctrl Pts',(0.137630738076998,-0.0212154088568283,
-0.95143037433829));
#45021=CARTESIAN_POINT('Ctrl Pts',(0.0923513834783183,0.104228286017869,
-0.943483083030339));
#45022=CARTESIAN_POINT('Ctrl Pts',(-0.0376312812236582,0.13407535310432,
-0.935535791722386));
#45023=CARTESIAN_POINT('Ctrl Pts',(-0.110787333250892,0.0627146963454166,
-0.92944586022107));
#45024=CARTESIAN_POINT('Ctrl Pts',(-0.117795616112498,0.011834854832662,
-0.926005025822403));
#45025=CARTESIAN_POINT('Ctrl Pts',(-0.117699425459372,0.000101537840546503,
-0.925213288526387));
#45026=CARTESIAN_POINT('Origin',(0.,0.,-3.06008671147362));
#45027=CARTESIAN_POINT('',(-0.117613627014458,6.24323588500954E-5,-1.03508671147362));
#45028=CARTESIAN_POINT('',(-0.11771557645994,-0.000104556441113679,-1.02521328852639));
#45029=CARTESIAN_POINT('',(-0.117775,1.13296574333067E-13,-3.06008671147362));
#45030=CARTESIAN_POINT('Ctrl Pts',(-0.117613627014458,6.24323588500949E-5,
-1.03508671147362));
#45031=CARTESIAN_POINT('Ctrl Pts',(-0.117499984628548,-0.0236264518139759,
-1.03349116967962));
#45032=CARTESIAN_POINT('Ctrl Pts',(-0.0990513846795703,-0.0868091095822184,
-1.02924653078297));
#45033=CARTESIAN_POINT('Ctrl Pts',(0.00409282660561049,-0.13919613029893,
-1.02235279478367));
#45034=CARTESIAN_POINT('Ctrl Pts',(0.119246473329177,-0.0719207377490957,
-1.01440550347571));
#45035=CARTESIAN_POINT('Ctrl Pts',(0.12502903508685,0.0613192816744626,
-1.00645821216776));
#45036=CARTESIAN_POINT('Ctrl Pts',(0.0161368325691865,0.138318171454277,
-0.998510920859808));
#45037=CARTESIAN_POINT('Ctrl Pts',(-0.0947394295923312,0.0936204014483265,
-0.991387087295095));
#45038=CARTESIAN_POINT('Ctrl Pts',(-0.117473353279,0.0269642398256485,-0.986912350833033));
#45039=CARTESIAN_POINT('Ctrl Pts',(-0.117686879986589,-9.84958757579094E-5,
-0.985086711473621));
#45040=CARTESIAN_POINT('Ctrl Pts',(-0.11771557645994,-0.000104556441113676,
-1.02521328852639));
#45041=CARTESIAN_POINT('Ctrl Pts',(-0.117810672883519,-0.011251489233664,
-1.02446085772088));
#45042=CARTESIAN_POINT('Ctrl Pts',(-0.111239157541274,-0.0615337344264252,
-1.02105932981271));
#45043=CARTESIAN_POINT('Ctrl Pts',(-0.0396138321773288,-0.133503025946263,
-1.0150087048019));
#45044=CARTESIAN_POINT('Ctrl Pts',(0.0907968256135503,-0.105585274044654,
-1.00706141349395));
#45045=CARTESIAN_POINT('Ctrl Pts',(0.137929990564865,0.0191737148032896,
-0.999114122186));
#45046=CARTESIAN_POINT('Ctrl Pts',(0.0585558274900352,0.126346858700717,
-0.991166830878047));
#45047=CARTESIAN_POINT('Ctrl Pts',(-0.0745248663094564,0.117636550179523,
-0.983219539570098));
#45048=CARTESIAN_POINT('Ctrl Pts',(-0.117836667080937,0.0396116618043791,
-0.977901692119542));
#45049=CARTESIAN_POINT('Ctrl Pts',(-0.11796887045282,0.000294971657115395,
-0.975232941771639));
#45050=CARTESIAN_POINT('Ctrl Pts',(-0.117968676352971,5.43384420481787E-6,
-0.975213288526387));
#45051=CARTESIAN_POINT('Origin',(0.,0.,-3.06008671147362));
#45052=CARTESIAN_POINT('',(-0.117915488935345,7.05844075192093E-5,-1.08508671147362));
#45053=CARTESIAN_POINT('',(-0.117598824873155,4.73937789327097E-5,-1.07521328852639));
#45054=CARTESIAN_POINT('',(-0.117775,1.13296574333067E-13,-3.06008671147362));
#45055=CARTESIAN_POINT('Ctrl Pts',(-0.117915488935345,7.05844075192083E-5,
-1.08508671147362));
#45056=CARTESIAN_POINT('Ctrl Pts',(-0.117668354362795,-0.0348517922405095,
-1.08271908562885));
#45057=CARTESIAN_POINT('Ctrl Pts',(-0.0827226944694583,-0.109277798319543,
-1.07770236268144));
#45058=CARTESIAN_POINT('Ctrl Pts',(0.043866657927493,-0.132166675989422,
-1.07003654263137));
#45059=CARTESIAN_POINT('Ctrl Pts',(0.134870236095805,-0.0346746785894572,
-1.06208925132342));
#45060=CARTESIAN_POINT('Ctrl Pts',(0.102172847354302,0.0946204163134727,
-1.05414196001547));
#45061=CARTESIAN_POINT('Ctrl Pts',(-0.0242359515212969,0.137131078073783,
-1.04619466870752));
#45062=CARTESIAN_POINT('Ctrl Pts',(-0.107500160123668,0.0705836828280244,
-1.03984291919357));
#45063=CARTESIAN_POINT('Ctrl Pts',(-0.11768866643957,0.0157044855912191,
-1.03614026678227));
#45064=CARTESIAN_POINT('Ctrl Pts',(-0.117613627014458,6.24323588500949E-5,
-1.03508671147362));
#45065=CARTESIAN_POINT('Ctrl Pts',(-0.117598824873155,4.73937789327028E-5,
-1.07521328852639));
#45066=CARTESIAN_POINT('Ctrl Pts',(-0.117516998884501,-0.0225940828510371,
-1.07368877367011));
#45067=CARTESIAN_POINT('Ctrl Pts',(-0.100292170955009,-0.0846940636737381,
-1.06951516171119));
#45068=CARTESIAN_POINT('Ctrl Pts',(0.00036461620057585,-0.139255810261576,
-1.06269245264961));
#45069=CARTESIAN_POINT('Ctrl Pts',(0.117278168930411,-0.0750875803905805,
-1.05474516134166));
#45070=CARTESIAN_POINT('Ctrl Pts',(0.126625936101752,0.0579498571433683,
-1.04679787003371));
#45071=CARTESIAN_POINT('Ctrl Pts',(0.0198342852289171,0.137836550907369,
-1.03885057872576));
#45072=CARTESIAN_POINT('Ctrl Pts',(-0.0933159459371162,0.0957074358369753,
-1.03165571822332));
#45073=CARTESIAN_POINT('Ctrl Pts',(-0.117475865139962,0.0279937239446263,
-1.02710995482353));
#45074=CARTESIAN_POINT('Ctrl Pts',(-0.11771557645994,-0.000104556441113676,
-1.02521328852639));
#45075=CARTESIAN_POINT('Origin',(0.,0.,-3.06008671147362));
#45076=CARTESIAN_POINT('',(-0.117831609157221,-0.000101687419266419,-1.13508671147362));
#45077=CARTESIAN_POINT('',(-0.117889553338148,8.37928209511622E-5,-1.12521328852639));
#45078=CARTESIAN_POINT('',(-0.117775,1.13296574333067E-13,-3.06008671147362));
#45079=CARTESIAN_POINT('Ctrl Pts',(-0.117831609157221,-0.000101687419266441,
-1.13508671147362));
#45080=CARTESIAN_POINT('Ctrl Pts',(-0.117897702251559,-0.00735161785805869,
-1.13459609868074));
#45081=CARTESIAN_POINT('Ctrl Pts',(-0.113984098036961,-0.053676869687243,
-1.13145638878521));
#45082=CARTESIAN_POINT('Ctrl Pts',(-0.0525767967102828,-0.128949580718614,
-1.12566758178704));
#45083=CARTESIAN_POINT('Ctrl Pts',(0.0799502236678128,-0.114018751331906,
-1.11772029047908));
#45084=CARTESIAN_POINT('Ctrl Pts',(0.13914809256923,0.00548837445564355,
-1.10977299917113));
#45085=CARTESIAN_POINT('Ctrl Pts',(0.0707214084725853,0.11996164513491,
-1.10182570786318));
#45086=CARTESIAN_POINT('Ctrl Pts',(-0.0625698955915714,0.124407885945709,
-1.09387841655523));
#45087=CARTESIAN_POINT('Ctrl Pts',(-0.115860262917991,0.0474181950354391,
-1.08829875109204));
#45088=CARTESIAN_POINT('Ctrl Pts',(-0.117944869117673,0.00422227303062001,
-1.08536818273151));
#45089=CARTESIAN_POINT('Ctrl Pts',(-0.117915488935345,7.05844075192083E-5,
-1.08508671147362));
#45090=CARTESIAN_POINT('Ctrl Pts',(-0.117889553338148,8.37928209511596E-5,
-1.12521328852639));
#45091=CARTESIAN_POINT('Ctrl Pts',(-0.117616609082175,-0.0338104601163673,
-1.12291668961935));
#45092=CARTESIAN_POINT('Ctrl Pts',(-0.0844519668986341,-0.107267264374004,
-1.11797099360966));
#45093=CARTESIAN_POINT('Ctrl Pts',(0.0403123913820496,-0.13329375355823,
-1.11037620049732));
#45094=CARTESIAN_POINT('Ctrl Pts',(0.133893531780113,-0.0382731731638424,
-1.10242890918937));
#45095=CARTESIAN_POINT('Ctrl Pts',(0.10466952388434,0.0918509902309573,
-1.09448161788142));
#45096=CARTESIAN_POINT('Ctrl Pts',(-0.0205558085830443,0.137730796737981,
-1.08653432657347));
#45097=CARTESIAN_POINT('Ctrl Pts',(-0.106522535859557,0.0727175613247637,
-1.08011155012179));
#45098=CARTESIAN_POINT('Ctrl Pts',(-0.117659185094477,0.0167492334133705,
-1.07633787077276));
#45099=CARTESIAN_POINT('Ctrl Pts',(-0.117598824873155,4.73937789327028E-5,
-1.07521328852639));
#45100=CARTESIAN_POINT('Origin',(0.,0.,-3.06008671147362));
#45101=CARTESIAN_POINT('',(-0.117582462475556,-1.51080851551548E-5,-1.18508671147362));
#45102=CARTESIAN_POINT('',(-0.117862347076416,-9.38393982804209E-5,-1.17521328852639));
#45103=CARTESIAN_POINT('',(-0.117775,1.13296574333067E-13,-3.06008671147362));
#45104=CARTESIAN_POINT('Ctrl Pts',(-0.117582462475556,-1.51080851551744E-5,
-1.18508671147362));
#45105=CARTESIAN_POINT('Ctrl Pts',(-0.117603898091645,-0.0187746844758571,
-1.18382401462998));
#45106=CARTESIAN_POINT('Ctrl Pts',(-0.104512501002388,-0.0768629882428656,
-1.17991222068369));
#45107=CARTESIAN_POINT('Ctrl Pts',(-0.0133598268380069,-0.138613956536415,
-1.17335132963475));
#45108=CARTESIAN_POINT('Ctrl Pts',(0.10930800785607,-0.0862790434483248,
-1.16540403832679));
#45109=CARTESIAN_POINT('Ctrl Pts',(0.131720169733078,0.0451897201286931,
-1.15745674701884));
#45110=CARTESIAN_POINT('Ctrl Pts',(0.0333205585370974,0.135211147094447,
-1.14950945571089));
#45111=CARTESIAN_POINT('Ctrl Pts',(-0.0876789955812038,0.103317381663382,
-1.14205277719582));
#45112=CARTESIAN_POINT('Ctrl Pts',(-0.117540828098952,0.0317948740366197,
-1.13724519578339));
#45113=CARTESIAN_POINT('Ctrl Pts',(-0.117831609157221,-0.000101687419266441,
-1.13508671147362));
#45114=CARTESIAN_POINT('Ctrl Pts',(-0.117862347076416,-9.38393982804252E-5,
-1.17521328852639));
#45115=CARTESIAN_POINT('Ctrl Pts',(-0.1179162650566,-0.00628999992156921,
-1.17479370267124));
#45116=CARTESIAN_POINT('Ctrl Pts',(-0.114651893565344,-0.0515493094812837,
-1.17172501971343));
#45117=CARTESIAN_POINT('Ctrl Pts',(-0.0560103581567255,-0.127495699597034,
-1.16600723965299));
#45118=CARTESIAN_POINT('Ctrl Pts',(0.0768689022763401,-0.116118411543615,
-1.15805994834503));
#45119=CARTESIAN_POINT('Ctrl Pts',(0.139245153208294,0.00176094990851802,
-1.15011265703708));
#45120=CARTESIAN_POINT('Ctrl Pts',(0.0739078285731691,0.118025194395861,
-1.14216536572913));
#45121=CARTESIAN_POINT('Ctrl Pts',(-0.0592166529718895,0.126038492721028,
-1.13421807442118));
#45122=CARTESIAN_POINT('Ctrl Pts',(-0.11525354823914,0.0495416262248971,
-1.12856738202026));
#45123=CARTESIAN_POINT('Ctrl Pts',(-0.117931446747328,0.00528612178028246,
-1.125565786722));
#45124=CARTESIAN_POINT('Ctrl Pts',(-0.117889553338148,8.37928209511596E-5,
-1.12521328852639));
#45125=CARTESIAN_POINT('Origin',(0.,0.,-3.06008671147362));
#45126=CARTESIAN_POINT('',(-0.117776021319591,0.000108156687832219,-1.23508671147362));
#45127=CARTESIAN_POINT('',(-0.117588764972749,-3.20871466719039E-5,-1.22521328852639));
#45128=CARTESIAN_POINT('',(-0.117775,1.13296574333067E-13,-3.06008671147362));
#45129=CARTESIAN_POINT('Ctrl Pts',(-0.117776021319591,0.000108156687832213,
-1.23508671147362));
#45130=CARTESIAN_POINT('Ctrl Pts',(-0.117498350433057,-0.0299968654539389,
-1.23305193057921));
#45131=CARTESIAN_POINT('Ctrl Pts',(-0.0904196508311549,-0.0997397256260159,
-1.22836805258216));
#45132=CARTESIAN_POINT('Ctrl Pts',(0.0269810332845223,-0.136617487031199,
-1.22103507748245));
#45133=CARTESIAN_POINT('Ctrl Pts',(0.12947029828579,-0.0512811445036981,
-1.2130877861745));
#45134=CARTESIAN_POINT('Ctrl Pts',(0.113211338714528,0.0810894981257437,
-1.20514049486655));
#45135=CARTESIAN_POINT('Ctrl Pts',(-0.00688337045973726,0.139086063755268,
-1.1971932035586));
#45136=CARTESIAN_POINT('Ctrl Pts',(-0.102586721940106,0.0805686970688501,
-1.19050860909429));
#45137=CARTESIAN_POINT('Ctrl Pts',(-0.117558926862991,0.0205822995174214,
-1.18647311173263));
#45138=CARTESIAN_POINT('Ctrl Pts',(-0.117582462475556,-1.51080851551744E-5,
-1.18508671147362));
#45139=CARTESIAN_POINT('Ctrl Pts',(-0.117588764972749,-3.20871466718952E-5,
-1.22521328852639));
#45140=CARTESIAN_POINT('Ctrl Pts',(-0.117631858824093,-0.0177340663052872,
-1.22402161862047));
#45141=CARTESIAN_POINT('Ctrl Pts',(-0.10556436402768,-0.0747319718305033,
-1.22018085161191));
#45142=CARTESIAN_POINT('Ctrl Pts',(-0.01706619414058,-0.138206579634031,
-1.21369098750069));
#45143=CARTESIAN_POINT('Ctrl Pts',(0.106958846585331,-0.0891746532021148,
-1.20574369619274));
#45144=CARTESIAN_POINT('Ctrl Pts',(0.132882830138289,0.0416469337529245,
-1.19779640488479));
#45145=CARTESIAN_POINT('Ctrl Pts',(0.036928665853329,0.134270574866107,
-1.18984911357684));
#45146=CARTESIAN_POINT('Ctrl Pts',(-0.0860416897627608,0.105354972619519,
-1.18232140812404));
#45147=CARTESIAN_POINT('Ctrl Pts',(-0.117575848516499,0.0328300769073127,
-1.17744279977389));
#45148=CARTESIAN_POINT('Ctrl Pts',(-0.117862347076416,-9.38393982804252E-5,
-1.17521328852639));
#45149=CARTESIAN_POINT('Origin',(0.,0.,-3.06008671147362));
#45150=CARTESIAN_POINT('',(-0.117950597231983,-4.22694188566558E-5,-1.28508671147362));
#45151=CARTESIAN_POINT('',(-0.117744385826804,0.000107701528469582,-1.27521328852639));
#45152=CARTESIAN_POINT('',(-0.117775,1.13296574333067E-13,-3.06008671147362));
#45153=CARTESIAN_POINT('Ctrl Pts',(-0.117950597231983,-4.22694188566583E-5,
-1.28508671147362));
#45154=CARTESIAN_POINT('Ctrl Pts',(-0.117961342406869,-0.00236750816820977,
-1.2849289436311));
#45155=CARTESIAN_POINT('Ctrl Pts',(-0.116844235725132,-0.0437255601152145,
-1.28212207868593));
#45156=CARTESIAN_POINT('Ctrl Pts',(-0.0683015385030549,-0.121355732282971,
-1.27666611663811));
#45157=CARTESIAN_POINT('Ctrl Pts',(0.0650521244483742,-0.123128124425631,
-1.26871882533016));
#45158=CARTESIAN_POINT('Ctrl Pts',(0.138740950095853,-0.0119692391704875,
-1.26077153402221));
#45159=CARTESIAN_POINT('Ctrl Pts',(0.0851786477431396,0.110167653548901,
-1.25282424271426));
#45160=CARTESIAN_POINT('Ctrl Pts',(-0.0465082385868169,0.131260419256424,
-1.24487695140631));
#45161=CARTESIAN_POINT('Ctrl Pts',(-0.112743652358229,0.0573866324060485,
-1.23896444099276));
#45162=CARTESIAN_POINT('Ctrl Pts',(-0.117859852324013,0.00919709746870165,
-1.23570102768187));
#45163=CARTESIAN_POINT('Ctrl Pts',(-0.117776021319591,0.000108156687832213,
-1.23508671147362));
#45164=CARTESIAN_POINT('Ctrl Pts',(-0.117744385826804,0.000107701528469589,
-1.27521328852639));
#45165=CARTESIAN_POINT('Ctrl Pts',(-0.117483723357635,-0.0289663776992756,
-1.27324953456971));
#45166=CARTESIAN_POINT('Ctrl Pts',(-0.0919304336464584,-0.0976706501736823,
-1.26863668351038));
#45167=CARTESIAN_POINT('Ctrl Pts',(0.0233136568373885,-0.137290884771896,
-1.2613747353484));
#45168=CARTESIAN_POINT('Ctrl Pts',(0.128050919416408,-0.0547291117522856,
-1.25342744404045));
#45169=CARTESIAN_POINT('Ctrl Pts',(0.115341790530312,0.0780293854508893,
-1.2454801527325));
#45170=CARTESIAN_POINT('Ctrl Pts',(-0.003157106556191,0.139220495311483,
-1.23753286142455));
#45171=CARTESIAN_POINT('Ctrl Pts',(-0.101426030289338,0.0826920768249464,
-1.23077724002251));
#45172=CARTESIAN_POINT('Ctrl Pts',(-0.117536060653668,0.0216176547271468,
-1.22667071572312));
#45173=CARTESIAN_POINT('Ctrl Pts',(-0.117588764972749,-3.20871466718952E-5,
-1.22521328852639));
#45174=CARTESIAN_POINT('Origin',(0.,0.,-3.06008671147362));
#45175=CARTESIAN_POINT('',(-0.117648697715254,-8.46313478923296E-5,-1.33508671147362));
#45176=CARTESIAN_POINT('',(-0.117963151496065,-2.37579109470393E-5,-1.32521328852639));
#45177=CARTESIAN_POINT('',(-0.117775,1.13296574333067E-13,-3.06008671147362));
#45178=CARTESIAN_POINT('Ctrl Pts',(-0.117648697715254,-8.46313478923295E-5,
-1.33508671147362));
#45179=CARTESIAN_POINT('Ctrl Pts',(-0.11774013592033,-0.0138797514576444,
-1.33415685958034));
#45180=CARTESIAN_POINT('Ctrl Pts',(-0.109114338455593,-0.0668657107954565,
-1.33057791058441));
#45181=CARTESIAN_POINT('Ctrl Pts',(-0.0306024039612664,-0.135852150485784,
-1.32434986448582));
#45182=CARTESIAN_POINT('Ctrl Pts',(0.097650730877784,-0.0992806561161591,
-1.31640257317787));
#45183=CARTESIAN_POINT('Ctrl Pts',(0.136340073298976,0.0283495737648783,
-1.30845528186992));
#45184=CARTESIAN_POINT('Ctrl Pts',(0.0499803360725424,0.129977997853083,
-1.30050799056197));
#45185=CARTESIAN_POINT('Ctrl Pts',(-0.0795961955054469,0.112741645408569,
-1.29271846709654));
#45186=CARTESIAN_POINT('Ctrl Pts',(-0.117780918999896,0.036675830040556,
-1.28757804073375));
#45187=CARTESIAN_POINT('Ctrl Pts',(-0.117950597231983,-4.22694188566583E-5,
-1.28508671147362));
#45188=CARTESIAN_POINT('Ctrl Pts',(-0.117963151496065,-2.3757910947049E-5,
-1.32521328852639));
#45189=CARTESIAN_POINT('Ctrl Pts',(-0.11796667100053,-0.00130181316577145,
-1.32512654762159));
#45190=CARTESIAN_POINT('Ctrl Pts',(-0.117368372503623,-0.0416087406635258,
-1.32239070961415));
#45191=CARTESIAN_POINT('Ctrl Pts',(-0.0715261504195623,-0.119483569760616,
-1.31700577450407));
#45192=CARTESIAN_POINT('Ctrl Pts',(0.0617322554776575,-0.124825647485695,
-1.30905848319611));
#45193=CARTESIAN_POINT('Ctrl Pts',(0.138370758324617,-0.0156795050066074,
-1.30111119188816));
#45194=CARTESIAN_POINT('Ctrl Pts',(0.0880976675369301,0.107847645366666,
-1.29316390058021));
#45195=CARTESIAN_POINT('Ctrl Pts',(-0.0429772886013641,0.132458545594676,
-1.28521660927226));
#45196=CARTESIAN_POINT('Ctrl Pts',(-0.111985965485845,0.0595187591475933,
-1.27923307192098));
#45197=CARTESIAN_POINT('Ctrl Pts',(-0.11783535610139,0.0102544517649053,
-1.27589863167236));
#45198=CARTESIAN_POINT('Ctrl Pts',(-0.117744385826804,0.000107701528469589,
-1.27521328852639));
#45199=CARTESIAN_POINT('Origin',(0.,0.,-3.06008671147362));
#45200=CARTESIAN_POINT('',(-0.117643137731857,8.18848197860175E-5,-1.38508671147362));
#45201=CARTESIAN_POINT('',(-0.117673475788507,-9.44926190546702E-5,-1.37521328852639));
#45202=CARTESIAN_POINT('',(-0.117775,1.13296574333067E-13,-3.06008671147362));
#45203=CARTESIAN_POINT('Ctrl Pts',(-0.117643137731858,8.18848197859986E-5,
-1.38508671147362));
#45204=CARTESIAN_POINT('Ctrl Pts',(-0.117481692417359,-0.0251707373262468,
-1.38338477552957));
#45205=CARTESIAN_POINT('Ctrl Pts',(-0.0971137812511854,-0.0899671114874316,
-1.37903374248288));
#45206=CARTESIAN_POINT('Ctrl Pts',(0.00967114594259312,-0.13892005922824,
-1.37203361233354));
#45207=CARTESIAN_POINT('Ctrl Pts',(0.122034507452407,-0.0670812411234985,
-1.36408632102558));
#45208=CARTESIAN_POINT('Ctrl Pts',(0.122469640724355,0.0662834898045348,
-1.35613902971763));
#45209=CARTESIAN_POINT('Ctrl Pts',(0.0105774480180276,0.138853993508456,
-1.34819173840968));
#45210=CARTESIAN_POINT('Ctrl Pts',(-0.0967894748877886,0.0904795809546536,
-1.34117429899501));
#45211=CARTESIAN_POINT('Ctrl Pts',(-0.11747963348345,0.0254217899787136,
-1.33680595668299));
#45212=CARTESIAN_POINT('Ctrl Pts',(-0.117648697715254,-8.46313478923295E-5,
-1.33508671147362));
#45213=CARTESIAN_POINT('Ctrl Pts',(-0.117673475788507,-9.44926190546719E-5,
-1.37521328852639));
#45214=CARTESIAN_POINT('Ctrl Pts',(-0.117769086788655,-0.0128291175224179,
-1.37435446357083));
#45215=CARTESIAN_POINT('Ctrl Pts',(-0.109991446578368,-0.0647308244202197,
-1.37084654151263));
#45216=CARTESIAN_POINT('Ctrl Pts',(-0.0342286474655051,-0.134984122508034,
-1.36468952235177));
#45217=CARTESIAN_POINT('Ctrl Pts',(0.0949576520728147,-0.10185950102666,
-1.35674223104382));
#45218=CARTESIAN_POINT('Ctrl Pts',(0.137050210865036,0.0246891340154153,
-1.34879493973587));
#45219=CARTESIAN_POINT('Ctrl Pts',(0.0534423624365219,0.12859326395183,
-1.34084764842792));
#45220=CARTESIAN_POINT('Ctrl Pts',(-0.0777344908263304,0.114706808671506,
-1.33298709802476));
#45221=CARTESIAN_POINT('Ctrl Pts',(-0.117859184122194,0.0377304344315316,
-1.32777564472425));
#45222=CARTESIAN_POINT('Ctrl Pts',(-0.117963151496065,-2.3757910947049E-5,
-1.32521328852639));
#45223=CARTESIAN_POINT('Origin',(0.,0.,-3.06008671147362));
#45224=CARTESIAN_POINT('',(-0.117946614788854,4.6571822748169E-5,-1.43508671147362));
#45225=CARTESIAN_POINT('',(-0.117622503294115,6.93536635249722E-5,-1.42521328852639));
#45226=CARTESIAN_POINT('',(-0.117775,1.13296574333067E-13,-3.06008671147362));
#45227=CARTESIAN_POINT('Ctrl Pts',(-0.117946614788854,4.65718227481639E-5,
-1.43508671147362));
#45228=CARTESIAN_POINT('Ctrl Pts',(-0.11776338497764,-0.0364196896702833,
-1.43261269147881));
#45229=CARTESIAN_POINT('Ctrl Pts',(-0.0800425056981712,-0.112260027951507,
-1.42748957438135));
#45230=CARTESIAN_POINT('Ctrl Pts',(0.0491311144456285,-0.130301371877472,
-1.41971736018124));
#45231=CARTESIAN_POINT('Ctrl Pts',(0.136152178426768,-0.0292386427432272,
-1.41177006887329));
#45232=CARTESIAN_POINT('Ctrl Pts',(0.0982964971317635,0.0986413329768289,
-1.40382277756534));
#45233=CARTESIAN_POINT('Ctrl Pts',(-0.0297152637478395,0.136048950823653,
-1.39587548625739));
#45234=CARTESIAN_POINT('Ctrl Pts',(-0.108895140667733,0.0673859988607212,
-1.38963013089348));
#45235=CARTESIAN_POINT('Ctrl Pts',(-0.117732985256182,0.014135470639733,
-1.38603387263222));
#45236=CARTESIAN_POINT('Ctrl Pts',(-0.117643137731858,8.18848197859986E-5,
-1.38508671147362));
#45237=CARTESIAN_POINT('Ctrl Pts',(-0.117622503294115,6.9353663524974E-5,
-1.42521328852639));
#45238=CARTESIAN_POINT('Ctrl Pts',(-0.117492881168235,-0.0241400490349439,
-1.42358237952007));
#45239=CARTESIAN_POINT('Ctrl Pts',(-0.0984178786166064,-0.0878603341406336,
-1.4193023734111));
#45240=CARTESIAN_POINT('Ctrl Pts',(0.0059483271787393,-0.139129188312001,
-1.41237327019948));
#45241=CARTESIAN_POINT('Ctrl Pts',(0.120194773022965,-0.0703244635567145,
-1.40442597889153));
#45242=CARTESIAN_POINT('Ctrl Pts',(0.12420036758044,0.0629808092157078,
-1.39647868758358));
#45243=CARTESIAN_POINT('Ctrl Pts',(0.0142912393273046,0.138521024090466,
-1.38853139627563));
#45244=CARTESIAN_POINT('Ctrl Pts',(-0.0954317712490366,0.0925781715067274,
-1.38144292992323));
#45245=CARTESIAN_POINT('Ctrl Pts',(-0.117474168922288,0.0264515970361115,
-1.37700356067348));
#45246=CARTESIAN_POINT('Ctrl Pts',(-0.117673475788507,-9.44926190546719E-5,
-1.37521328852639));
#45247=CARTESIAN_POINT('Origin',(0.,0.,-3.06008671147362));
#45248=CARTESIAN_POINT('',(-0.117783823687606,-0.000107808840122532,-1.48508671147362));
#45249=CARTESIAN_POINT('',(-0.11792699295135,6.31151991691888E-5,-1.47521328852639));
#45250=CARTESIAN_POINT('',(-0.117775,1.13296574333067E-13,-3.06008671147362));
#45251=CARTESIAN_POINT('Ctrl Pts',(-0.117783823687606,-0.000107808840122531,
-1.48508671147362));
#45252=CARTESIAN_POINT('Ctrl Pts',(-0.117865535679874,-0.00893915841207697,
-1.4844897045307));
#45253=CARTESIAN_POINT('Ctrl Pts',(-0.112923229129106,-0.0568672450942766,
-1.48124360048513));
#45254=CARTESIAN_POINT('Ctrl Pts',(-0.0473637742173777,-0.130954140109069,
-1.47534839933691));
#45255=CARTESIAN_POINT('Ctrl Pts',(0.0844579470046824,-0.110721132163533,
-1.46740110802895));
#45256=CARTESIAN_POINT('Ctrl Pts',(0.138816100206623,0.0110636451156712,
-1.459453816721));
#45257=CARTESIAN_POINT('Ctrl Pts',(0.0658541988487744,0.122701012277025,
-1.45150652541305));
#45258=CARTESIAN_POINT('Ctrl Pts',(-0.0675081904779539,0.121798842926412,
-1.4435592341051));
#45259=CARTESIAN_POINT('Ctrl Pts',(-0.116712029120029,0.0442418089731312,
-1.43808596279196));
#45260=CARTESIAN_POINT('Ctrl Pts',(-0.11795958127477,0.00262715225840995,
-1.43526178858146));
#45261=CARTESIAN_POINT('Ctrl Pts',(-0.117946614788854,4.65718227481639E-5,
-1.43508671147362));
#45262=CARTESIAN_POINT('Ctrl Pts',(-0.11792699295135,6.3115199169191E-5,
-1.47521328852638));
#45263=CARTESIAN_POINT('Ctrl Pts',(-0.11769755575331,-0.0353718248083651,
-1.4728102954693));
#45264=CARTESIAN_POINT('Ctrl Pts',(-0.0818437614380234,-0.110273199218807,
-1.46775820530957));
#45265=CARTESIAN_POINT('Ctrl Pts',(0.045624901106524,-0.131570065119699,
-1.46005701804719));
#45266=CARTESIAN_POINT('Ctrl Pts',(0.135320555318067,-0.0328734078700636,
-1.45210972673924));
#45267=CARTESIAN_POINT('Ctrl Pts',(0.100902216552484,0.0959742482720097,
-1.44416243543129));
#45268=CARTESIAN_POINT('Ctrl Pts',(-0.0260621287465163,0.13679575681205,
-1.43621514412334));
#45269=CARTESIAN_POINT('Ctrl Pts',(-0.107973035031269,0.0695208292702655,
-1.4298987618217));
#45270=CARTESIAN_POINT('Ctrl Pts',(-0.117703427309545,0.0151834560147021,
-1.42623147662272));
#45271=CARTESIAN_POINT('Ctrl Pts',(-0.117622503294115,6.9353663524974E-5,
-1.42521328852639));
#45272=CARTESIAN_POINT('Origin',(0.,0.,-3.06008671147362));
#45273=CARTESIAN_POINT('',(-0.117581619011794,1.08966417829141E-5,-1.53508671147362));
#45274=CARTESIAN_POINT('',(-0.117815844487591,-0.000104481014402413,-1.52521328852638));
#45275=CARTESIAN_POINT('',(-0.117775,1.13296574333067E-13,-3.06008671147362));
#45276=CARTESIAN_POINT('Ctrl Pts',(-0.117581619011794,1.089664178292E-5,
-1.53508671147362));
#45277=CARTESIAN_POINT('Ctrl Pts',(-0.117564862655435,-0.0203297153006686,
-1.53371762047993));
#45278=CARTESIAN_POINT('Ctrl Pts',(-0.102863457479005,-0.0800507033264646,
-1.5296994323836));
#45279=CARTESIAN_POINT('Ctrl Pts',(-0.00779081513336725,-0.139038185831728,
-1.52303214718461));
#45280=CARTESIAN_POINT('Ctrl Pts',(0.112679787534581,-0.0818265201568669,
-1.51508485587666));
#45281=CARTESIAN_POINT('Ctrl Pts',(0.129802171405619,0.0504352081209822,
-1.50713756456871));
#45282=CARTESIAN_POINT('Ctrl Pts',(0.0278719416335478,0.136438516517136,
-1.49919027326076));
#45283=CARTESIAN_POINT('Ctrl Pts',(-0.0900445677183776,0.100242387200107,
-1.49183998889573));
#45284=CARTESIAN_POINT('Ctrl Pts',(-0.117502955303656,0.0302481623401825,
-1.48713880163335));
#45285=CARTESIAN_POINT('Ctrl Pts',(-0.117783823687606,-0.000107808840122531,
-1.48508671147362));
#45286=CARTESIAN_POINT('Ctrl Pts',(-0.117815844487591,-0.000104481014402428,
-1.52521328852638));
#45287=CARTESIAN_POINT('Ctrl Pts',(-0.117887561503818,-0.00787972330702221,
-1.52468730852119));
#45288=CARTESIAN_POINT('Ctrl Pts',(-0.113639577894226,-0.054736975302814,
-1.52151223141335));
#45289=CARTESIAN_POINT('Ctrl Pts',(-0.0508528731324187,-0.129639110343907,
-1.51568805720286));
#45290=CARTESIAN_POINT('Ctrl Pts',(0.0814632979273637,-0.112942661237371,
-1.5077407658949));
#45291=CARTESIAN_POINT('Ctrl Pts',(0.139062548390083,0.0073431105015257,
-1.49979347458695));
#45292=CARTESIAN_POINT('Ctrl Pts',(0.0691157056986611,0.120893890922402,
-1.491846183279));
#45293=CARTESIAN_POINT('Ctrl Pts',(-0.0642230303494631,0.123562599557122,
-1.48389889197105));
#45294=CARTESIAN_POINT('Ctrl Pts',(-0.116150928522588,0.0463617126739875,
-1.47835459372018));
#45295=CARTESIAN_POINT('Ctrl Pts',(-0.117950490906318,0.00369220687078259,
-1.47545939257196));
#45296=CARTESIAN_POINT('Ctrl Pts',(-0.11792699295135,6.3115199169191E-5,
-1.47521328852638));
#45297=CARTESIAN_POINT('Origin',(0.,0.,-3.06008671147362));
#45298=CARTESIAN_POINT('',(-0.117823920457094,0.000103148469539977,-1.58508671147362));
#45299=CARTESIAN_POINT('',(-0.117581030135854,-6.48590087786588E-6,-1.57521328852638));
#45300=CARTESIAN_POINT('',(-0.117775,1.13296574333067E-13,-3.06008671147362));
#45301=CARTESIAN_POINT('Ctrl Pts',(-0.117823920457094,0.00010314846953997,
-1.58508671147362));
#45302=CARTESIAN_POINT('Ctrl Pts',(-0.117533506753675,-0.0315429534362953,
-1.58294553642917));
#45303=CARTESIAN_POINT('Ctrl Pts',(-0.0880709269273121,-0.102818908660365,
-1.57815526428207));
#45304=CARTESIAN_POINT('Ctrl Pts',(0.0324375432515528,-0.135425698106468,
-1.57071589503233));
#45305=CARTESIAN_POINT('Ctrl Pts',(0.131422484648456,-0.0460482838838423,
-1.56276860372437));
#45306=CARTESIAN_POINT('Ctrl Pts',(0.109868685287492,0.0855639288077546,
-1.55482131241642));
#45307=CARTESIAN_POINT('Ctrl Pts',(-0.0124550318596216,0.138698183481963,
-1.54687402110847));
#45308=CARTESIAN_POINT('Ctrl Pts',(-0.104250256091004,0.0773819952015474,
-1.5402958207942));
#45309=CARTESIAN_POINT('Ctrl Pts',(-0.117597285054886,0.0190279726919229,
-1.53636671758259));
#45310=CARTESIAN_POINT('Ctrl Pts',(-0.117581619011794,1.089664178292E-5,
-1.53508671147362));
#45311=CARTESIAN_POINT('Ctrl Pts',(-0.117581030135854,-6.48590087786935E-6,
-1.57521328852638));
#45312=CARTESIAN_POINT('Ctrl Pts',(-0.117590483811689,-0.0192920895595535,
-1.57391522447043));
#45313=CARTESIAN_POINT('Ctrl Pts',(-0.103974180293752,-0.0779232980843118,
-1.56996806331182));
#45314=CARTESIAN_POINT('Ctrl Pts',(-0.0115105368274101,-0.138779757812609,
-1.56337180505056));
#45315=CARTESIAN_POINT('Ctrl Pts',(0.110448626411003,-0.0848139997907445,
-1.55542451374261));
#45316=CARTESIAN_POINT('Ctrl Pts',(0.131105958523409,0.0469418925506857,
-1.54747722243466));
#45317=CARTESIAN_POINT('Ctrl Pts',(0.0315148629140466,0.135643381895656,
-1.53952993112671));
#45318=CARTESIAN_POINT('Ctrl Pts',(-0.0884768683350901,0.102298108392725,
-1.53210861982395));
#45319=CARTESIAN_POINT('Ctrl Pts',(-0.117526358914326,0.0312802668568986,
-1.52733640562384));
#45320=CARTESIAN_POINT('Ctrl Pts',(-0.117815844487591,-0.000104481014402428,
-1.52521328852638));
#45321=CARTESIAN_POINT('Origin',(0.,0.,-3.06008671147362));
#45322=CARTESIAN_POINT('',(-0.117921249980265,-6.69982741048494E-5,-1.63508671147362));
#45323=CARTESIAN_POINT('',(-0.117791976321323,0.000107252653627231,-1.62521328852638));
#45324=CARTESIAN_POINT('',(-0.117775,1.13296574333067E-13,-3.06008671147362));
#45325=CARTESIAN_POINT('Ctrl Pts',(-0.117921249980265,-6.69982741048542E-5,
-1.63508671147362));
#45326=CARTESIAN_POINT('Ctrl Pts',(-0.117947710639304,-0.00396287537901269,
-1.63482254948106));
#45327=CARTESIAN_POINT('Ctrl Pts',(-0.116003462933909,-0.0469010631975345,
-1.63190929038585));
#45328=CARTESIAN_POINT('Ctrl Pts',(-0.0633803737869685,-0.123996944068975,
-1.62634693418799));
#45329=CARTESIAN_POINT('Ctrl Pts',(0.0699371058934867,-0.120420576061834,
-1.61839964288003));
#45330=CARTESIAN_POINT('Ctrl Pts',(0.139109316222199,-0.00639625359196896,
-1.61045235157208));
#45331=CARTESIAN_POINT('Ctrl Pts',(0.0806925386394054,0.113494617175214,
-1.60250506026413));
#45332=CARTESIAN_POINT('Ctrl Pts',(-0.051734230629111,0.129289919564653,
-1.59455776895618));
#45333=CARTESIAN_POINT('Ctrl Pts',(-0.113816488971119,0.0541956459344663,
-1.58875165269268));
#45334=CARTESIAN_POINT('Ctrl Pts',(-0.117892811380493,0.00761012612454138,
-1.58559463353182));
#45335=CARTESIAN_POINT('Ctrl Pts',(-0.117823920457094,0.00010314846953997,
-1.58508671147362));
#45336=CARTESIAN_POINT('Ctrl Pts',(-0.117791976321323,0.000107252653627225,
-1.62521328852638));
#45337=CARTESIAN_POINT('Ctrl Pts',(-0.117508209392984,-0.0305104146554398,
-1.62314314041966));
#45338=CARTESIAN_POINT('Ctrl Pts',(-0.0896503593683097,-0.100766102680647,
-1.61842389521029));
#45339=CARTESIAN_POINT('Ctrl Pts',(0.0288001189230785,-0.136245611990252,
-1.61105555289827));
#45340=CARTESIAN_POINT('Ctrl Pts',(0.130142507042637,-0.0495503935124521,
-1.60310826159032));
#45341=CARTESIAN_POINT('Ctrl Pts',(0.112120130754087,0.0825917060985434,
-1.59516097028237));
#45342=CARTESIAN_POINT('Ctrl Pts',(-0.00873715548808248,0.138981925985211,
-1.58721367897442));
#45343=CARTESIAN_POINT('Ctrl Pts',(-0.103149623928905,0.0795101044780683,
-1.58056445172242));
#45344=CARTESIAN_POINT('Ctrl Pts',(-0.117571190691948,0.0200660889067739,
-1.57656432157308));
#45345=CARTESIAN_POINT('Ctrl Pts',(-0.117581030135854,-6.48590087786935E-6,
-1.57521328852638));
#45346=CARTESIAN_POINT('Origin',(0.,0.,-3.06008671147362));
#45347=CARTESIAN_POINT('',(-0.117617850646942,-6.5871718804936E-5,-1.68508671147362));
#45348=CARTESIAN_POINT('',(-0.117942108415767,-5.09551612454251E-5,-1.67521328852638));
#45349=CARTESIAN_POINT('',(-0.117775,1.13296574333067E-13,-3.06008671147362));
#45350=CARTESIAN_POINT('Ctrl Pts',(-0.117617850646942,-6.58717188049326E-5,
-1.68508671147362));
#45351=CARTESIAN_POINT('Ctrl Pts',(-0.117695889536837,-0.0154495527158428,
-1.68405046543029));
#45352=CARTESIAN_POINT('Ctrl Pts',(-0.107732741084233,-0.0700635255376361,
-1.68036512228432));
#45353=CARTESIAN_POINT('Ctrl Pts',(-0.0251302696981556,-0.136970009362336,
-1.6740306820357));
#45354=CARTESIAN_POINT('Ctrl Pts',(0.101553236631872,-0.0952851197690979,
-1.66608339072774));
#45355=CARTESIAN_POINT('Ctrl Pts',(0.135093630531518,0.0337938590521173,
-1.65813609941979));
#45356=CARTESIAN_POINT('Ctrl Pts',(0.0447281634802288,0.131877614899218,
-1.65018880811184));
#45357=CARTESIAN_POINT('Ctrl Pts',(-0.0822940200144428,0.109765453494247,
-1.64250567879645));
#45358=CARTESIAN_POINT('Ctrl Pts',(-0.117682355072768,0.0351061695311471,
-1.63747164658371));
#45359=CARTESIAN_POINT('Ctrl Pts',(-0.117921249980265,-6.69982741048542E-5,
-1.63508671147362));
#45360=CARTESIAN_POINT('Ctrl Pts',(-0.117942108415767,-5.09551612454281E-5,
-1.67521328852638));
#45361=CARTESIAN_POINT('Ctrl Pts',(-0.117957552138955,-0.00289799243842009,
-1.67502015347155));
#45362=CARTESIAN_POINT('Ctrl Pts',(-0.116572218065069,-0.0447805435194828,
-1.67217792131407));
#45363=CARTESIAN_POINT('Ctrl Pts',(-0.0666774638491984,-0.122255590674703,
-1.66668659205393));
#45364=CARTESIAN_POINT('Ctrl Pts',(0.0666879758411977,-0.122249856911105,
-1.65873930074598));
#45365=CARTESIAN_POINT('Ctrl Pts',(0.138888199753706,-0.0101183796013297,
-1.65079200943803));
#45366=CARTESIAN_POINT('Ctrl Pts',(0.0837022404783003,0.111293524409529,
-1.64284471813008));
#45367=CARTESIAN_POINT('Ctrl Pts',(-0.0482541640740641,0.130628669464612,
-1.63489742682213));
#45368=CARTESIAN_POINT('Ctrl Pts',(-0.113108473408961,0.056325488927834,
-1.6290202836209));
#45369=CARTESIAN_POINT('Ctrl Pts',(-0.117871336139931,0.00866995775128773,
-1.62579223752231));
#45370=CARTESIAN_POINT('Ctrl Pts',(-0.117791976321323,0.000107252653627225,
-1.62521328852638));
#45371=CARTESIAN_POINT('Origin',(0.,0.,-3.06008671147362));
#45372=CARTESIAN_POINT('',(-0.11768023886796,9.66154492266578E-5,-1.73508671147362));
#45373=CARTESIAN_POINT('',(-0.117637551566029,-7.88858851605845E-5,-1.72521328852638));
#45374=CARTESIAN_POINT('',(-0.117775,1.13296574333067E-13,-3.06008671147362));
#45375=CARTESIAN_POINT('Ctrl Pts',(-0.11768023886796,9.66154492266658E-5,
-1.73508671147362));
#45376=CARTESIAN_POINT('Ctrl Pts',(-0.117473587897162,-0.026713351369385,
-1.73327838137953));
#45377=CARTESIAN_POINT('Ctrl Pts',(-0.0950796332385711,-0.0931105570833916,
-1.72882095418279));
#45378=CARTESIAN_POINT('Ctrl Pts',(0.0152339085805741,-0.138420525750985,
-1.72171442988341));
#45379=CARTESIAN_POINT('Ctrl Pts',(0.124626240732756,-0.062133839738435,
-1.71376713857545));
#45380=CARTESIAN_POINT('Ctrl Pts',(0.11971324557739,0.0711410764126323,
-1.7058198472675));
#45381=CARTESIAN_POINT('Ctrl Pts',(0.00500104891906081,0.139166459427298,
-1.69787255595955));
#45382=CARTESIAN_POINT('Ctrl Pts',(-0.0987426466397743,0.087323766405728,
-1.69096151069492));
#45383=CARTESIAN_POINT('Ctrl Pts',(-0.117496388078233,0.0238778493233859,
-1.68669956253294));
#45384=CARTESIAN_POINT('Ctrl Pts',(-0.117617850646942,-6.58717188049326E-5,
-1.68508671147362));
#45385=CARTESIAN_POINT('Ctrl Pts',(-0.117637551566029,-7.88858851605862E-5,
-1.72521328852638));
#45386=CARTESIAN_POINT('Ctrl Pts',(-0.117725496492675,-0.0144021151159734,
-1.72424806942079));
#45387=CARTESIAN_POINT('Ctrl Pts',(-0.108664165918674,-0.06792878474672,
-1.72063375321254));
#45388=CARTESIAN_POINT('Ctrl Pts',(-0.0287884036356622,-0.136248087886369,
-1.71437033990164));
#45389=CARTESIAN_POINT('Ctrl Pts',(0.0989657326610272,-0.0979698800420198,
-1.70642304859369));
#45390=CARTESIAN_POINT('Ctrl Pts',(0.135949976537486,0.0301648390686699,
-1.69847575728574));
#45391=CARTESIAN_POINT('Ctrl Pts',(0.0482429316917392,0.130632818152132,
-1.69052846597779));
#45392=CARTESIAN_POINT('Ctrl Pts',(-0.0805050460052469,0.111756485186054,
-1.68277430972467));
#45393=CARTESIAN_POINT('Ctrl Pts',(-0.117745721498532,0.0361528065407269,
-1.6776692505742));
#45394=CARTESIAN_POINT('Ctrl Pts',(-0.117942108415767,-5.09551612454281E-5,
-1.67521328852638));
#45395=CARTESIAN_POINT('Origin',(0.,0.,-3.06008671147362));
#45396=CARTESIAN_POINT('',(-0.117965285605798,1.88808896691469E-5,-1.78508671147362));
#45397=CARTESIAN_POINT('',(-0.117654705075576,8.73580116268896E-5,-1.77521328852638));
#45398=CARTESIAN_POINT('',(-0.117775,1.13296574333067E-13,-3.06008671147362));
#45399=CARTESIAN_POINT('Ctrl Pts',(-0.117965285605798,1.88808896691539E-5,
-1.78508671147362));
#45400=CARTESIAN_POINT('Ctrl Pts',(-0.117880735353708,-0.0379995363499562,
-1.78250629732877));
#45401=CARTESIAN_POINT('Ctrl Pts',(-0.0772533694302627,-0.1152034904333,
-1.77727678608127));
#45402=CARTESIAN_POINT('Ctrl Pts',(0.054316540209444,-0.128226469106407,
-1.76939817773111));
#45403=CARTESIAN_POINT('Ctrl Pts',(0.137215110676543,-0.0237555745425038,
-1.76145088642316));
#45404=CARTESIAN_POINT('Ctrl Pts',(0.0942620302777797,0.102503578316717,
-1.75350359511521));
#45405=CARTESIAN_POINT('Ctrl Pts',(-0.0351467769424353,0.13474797954099,
-1.74555630380726));
#45406=CARTESIAN_POINT('Ctrl Pts',(-0.110208765147338,0.0641880976310302,
-1.7394173425934));
#45407=CARTESIAN_POINT('Ctrl Pts',(-0.117776319400548,0.0125616712902332,
-1.73592747848218));
#45408=CARTESIAN_POINT('Ctrl Pts',(-0.11768023886796,9.66154492266658E-5,
-1.73508671147362));
#45409=CARTESIAN_POINT('Ctrl Pts',(-0.117654705075576,8.73580116268809E-5,
-1.77521328852638));
#45410=CARTESIAN_POINT('Ctrl Pts',(-0.117477780202669,-0.0256836588302884,
-1.77347598537002));
#45411=CARTESIAN_POINT('Ctrl Pts',(-0.0964484074419039,-0.0910137929807851,
-1.76908958511102));
#45412=CARTESIAN_POINT('Ctrl Pts',(0.0115224698662327,-0.138778767557446,
-1.76205408774935));
#45413=CARTESIAN_POINT('Ctrl Pts',(0.122918035611167,-0.0654482250185099,
-1.7541067964414));
#45414=CARTESIAN_POINT('Ctrl Pts',(0.121575014282259,0.06791045235345,-1.74615950513345));
#45415=CARTESIAN_POINT('Ctrl Pts',(0.00872520499083007,0.138982676742282,
-1.7382122138255));
#45416=CARTESIAN_POINT('Ctrl Pts',(-0.0974493906730333,0.0894320653748823,
-1.73123014162315));
#45417=CARTESIAN_POINT('Ctrl Pts',(-0.117484126788099,0.0249087779610027,
-1.72689716652344));
#45418=CARTESIAN_POINT('Ctrl Pts',(-0.117637551566029,-7.88858851605862E-5,
-1.72521328852638));
#45419=CARTESIAN_POINT('Origin',(0.,0.,-3.06008671147362));
#45420=CARTESIAN_POINT('',(-0.117736502923752,-0.000107109896749501,-1.83508671147362));
#45421=CARTESIAN_POINT('',(-0.117954382942583,3.76844323675355E-5,-1.82521328852638));
#45422=CARTESIAN_POINT('',(-0.117775,1.13296574333067E-13,-3.06008671147362));
#45423=CARTESIAN_POINT('Ctrl Pts',(-0.117736502923752,-0.000107109896749515,
-1.83508671147362));
#45424=CARTESIAN_POINT('Ctrl Pts',(-0.117828850108629,-0.0105229883610132,
-1.83438331038065));
#45425=CARTESIAN_POINT('Ctrl Pts',(-0.11178794712638,-0.0600610348697975,
-1.83103081218504));
#45426=CARTESIAN_POINT('Ctrl Pts',(-0.0420745638576578,-0.132748050818114,
-1.82502921688678));
#45427=CARTESIAN_POINT('Ctrl Pts',(0.0888298139634637,-0.107245410489387,
-1.81708192557882));
#45428=CARTESIAN_POINT('Ctrl Pts',(0.13826081266264,0.0166211191466418,
-1.80913463427087));
#45429=CARTESIAN_POINT('Ctrl Pts',(0.0608810582468267,0.125243006457714,
-1.80118734296292));
#45430=CARTESIAN_POINT('Ctrl Pts',(-0.072337893827657,0.118993878146731,
-1.79324005165497));
#45431=CARTESIAN_POINT('Ctrl Pts',(-0.117496963864637,0.0410709634385956,
-1.78787317449187));
#45432=CARTESIAN_POINT('Ctrl Pts',(-0.117967536082299,0.00103081819907492,
-1.78515539443142));
#45433=CARTESIAN_POINT('Ctrl Pts',(-0.117965285605798,1.88808896691539E-5,
-1.78508671147362));
#45434=CARTESIAN_POINT('Ctrl Pts',(-0.117954382942583,3.76844323675288E-5,
-1.82521328852638));
#45435=CARTESIAN_POINT('Ctrl Pts',(-0.117799847059692,-0.0369433981909912,
-1.82270390131926));
#45436=CARTESIAN_POINT('Ctrl Pts',(-0.0791275006836936,-0.113242981745652,
-1.81754541700949));
#45437=CARTESIAN_POINT('Ctrl Pts',(0.0508640200603842,-0.129634737242294,
-1.80973783559706));
#45438=CARTESIAN_POINT('Ctrl Pts',(0.136529906497424,-0.0274207634537505,
-1.80179054428911));
#45439=CARTESIAN_POINT('Ctrl Pts',(0.0969726011114629,0.0999431251775667,
-1.79384325298116));
#45440=CARTESIAN_POINT('Ctrl Pts',(-0.0315265261952861,0.13564067156513,
-1.78589596167321));
#45441=CARTESIAN_POINT('Ctrl Pts',(-0.109340731502731,0.0663229187380152,
-1.77968597352162));
#45442=CARTESIAN_POINT('Ctrl Pts',(-0.117747561079132,0.0136128368897407,
-1.77612508247267));
#45443=CARTESIAN_POINT('Ctrl Pts',(-0.117654705075576,8.73580116268809E-5,
-1.77521328852638));
#45444=CARTESIAN_POINT('Origin',(0.,0.,-3.06008671147362));
#45445=CARTESIAN_POINT('',(-0.117591087501129,3.6292447154734E-5,-1.88508671147362));
#45446=CARTESIAN_POINT('',(-0.11776790710648,-0.000108326905674527,-1.87521328852638));
#45447=CARTESIAN_POINT('',(-0.117775,1.13296574333067E-13,-3.06008671147362));
#45448=CARTESIAN_POINT('Ctrl Pts',(-0.117591087501129,3.62924471547406E-5,
-1.88508671147362));
#45449=CARTESIAN_POINT('Ctrl Pts',(-0.117530670031507,-0.0218806161763991,
-1.88361122632989));
#45450=CARTESIAN_POINT('Ctrl Pts',(-0.101124441328067,-0.0832313222762371,
-1.87948664408351));
#45451=CARTESIAN_POINT('Ctrl Pts',(-0.00220927137030462,-0.139238762705767,
-1.87271296473448));
#45452=CARTESIAN_POINT('Ctrl Pts',(0.115870314076337,-0.077242373317187,
-1.86476567342653));
#45453=CARTESIAN_POINT('Ctrl Pts',(0.127675377417112,0.0555995676351779,
-1.85681838211858));
#45454=CARTESIAN_POINT('Ctrl Pts',(0.0223784908076123,0.137446415264255,
-1.84887109081063));
#45455=CARTESIAN_POINT('Ctrl Pts',(-0.0923073152845968,0.0971430293605453,
-1.84162720059564));
#45456=CARTESIAN_POINT('Ctrl Pts',(-0.117481058980149,0.0287045217143467,
-1.83703240748331));
#45457=CARTESIAN_POINT('Ctrl Pts',(-0.117736502923752,-0.000107109896749515,
-1.83508671147362));
#45458=CARTESIAN_POINT('Ctrl Pts',(-0.11776790710648,-0.000108326905674527,
-1.87521328852638));
#45459=CARTESIAN_POINT('Ctrl Pts',(-0.117853798527441,-0.00946608599639612,
-1.87458091437115));
#45460=CARTESIAN_POINT('Ctrl Pts',(-0.112554198892079,-0.0579285772143487,
-1.87129944311326));
#45461=CARTESIAN_POINT('Ctrl Pts',(-0.0456135877873082,-0.131573987724592,
-1.86536887475272));
#45462=CARTESIAN_POINT('Ctrl Pts',(0.085926654297937,-0.109585234944059,
-1.85742158344477));
#45463=CARTESIAN_POINT('Ctrl Pts',(0.138656251961757,0.0129134591995952,
-1.84947429213682));
#45464=CARTESIAN_POINT('Ctrl Pts',(0.0642124054894162,0.123568121365685,
-1.84152700082887));
#45465=CARTESIAN_POINT('Ctrl Pts',(-0.0691261005948764,0.120887947509786,
-1.83357970952092));
#45466=CARTESIAN_POINT('Ctrl Pts',(-0.116980282886529,0.0431871392476156,
-1.82814180542009));
#45467=CARTESIAN_POINT('Ctrl Pts',(-0.117962986713253,0.00209660271135738,
-1.82535299842191));
#45468=CARTESIAN_POINT('Ctrl Pts',(-0.117954382942583,3.76844323675288E-5,
-1.82521328852638));
#45469=CARTESIAN_POINT('Origin',(0.,0.,-3.06008671147362));
#45470=CARTESIAN_POINT('',(-0.117869880861692,9.13799831027575E-5,-1.93508671147362));
#45471=CARTESIAN_POINT('',(-0.117583632441682,1.94776852104478E-5,-1.92521328852638));
#45472=CARTESIAN_POINT('',(-0.117775,1.13296574333067E-13,-3.06008671147362));
#45473=CARTESIAN_POINT('Ctrl Pts',(-0.117869880861692,9.13799831027641E-5,
-1.93508671147362));
#45474=CARTESIAN_POINT('Ctrl Pts',(-0.117586069037807,-0.0330936947020148,
-1.93283914227913));
#45475=CARTESIAN_POINT('Ctrl Pts',(-0.0856179332394516,-0.10587091750467,
-1.92794247598199));
#45476=CARTESIAN_POINT('Ctrl Pts',(0.037841875214064,-0.134016067693779,
-1.92039671258219));
#45477=CARTESIAN_POINT('Ctrl Pts',(0.133163268965518,-0.0407413514532521,
-1.91244942127425));
#45478=CARTESIAN_POINT('Ctrl Pts',(0.106349300573725,0.0899007240643813,
-1.90450212996629));
#45479=CARTESIAN_POINT('Ctrl Pts',(-0.0180066584898106,0.138087197704393,
-1.89655483865834));
#45480=CARTESIAN_POINT('Ctrl Pts',(-0.105825629738042,0.0741898865853727,
-1.89008303249411));
#45481=CARTESIAN_POINT('Ctrl Pts',(-0.117639144009984,0.0174691660837329,
-1.88626032343254));
#45482=CARTESIAN_POINT('Ctrl Pts',(-0.117591087501129,3.62924471547406E-5,
-1.88508671147362));
#45483=CARTESIAN_POINT('Ctrl Pts',(-0.117583632441682,1.94776852104391E-5,
-1.92521328852638));
#45484=CARTESIAN_POINT('Ctrl Pts',(-0.117552877563387,-0.0208456941039662,
-1.92380883032038));
#45485=CARTESIAN_POINT('Ctrl Pts',(-0.102295467731519,-0.0811088855391901,
-1.91975527501173));
#45486=CARTESIAN_POINT('Ctrl Pts',(-0.00593636402933215,-0.139129699269039,
-1.91305262260043));
#45487=CARTESIAN_POINT('Ctrl Pts',(0.113760742075024,-0.0803169172660493,
-1.90510533129248));
#45488=CARTESIAN_POINT('Ctrl Pts',(0.129118194016824,0.052161342107116,
-1.89715803998453));
#45489=CARTESIAN_POINT('Ctrl Pts',(0.0260503661646103,0.136797997277999,
-1.88921074867658));
#45490=CARTESIAN_POINT('Ctrl Pts',(-0.0908080642029844,0.0992146499208666,
-1.88189583152386));
#45491=CARTESIAN_POINT('Ctrl Pts',(-0.117493988259224,0.0297347767986486,
-1.8772300114738));
#45492=CARTESIAN_POINT('Ctrl Pts',(-0.11776790710648,-0.000108326905674527,
-1.87521328852638));
#45493=CARTESIAN_POINT('Origin',(0.,0.,-3.06008671147362));
#45494=CARTESIAN_POINT('',(-0.117882453427845,-8.67389818698854E-5,-1.98508671147362));
#45495=CARTESIAN_POINT('',(-0.117839561452888,9.99727772240215E-5,-1.97521328852638));
#45496=CARTESIAN_POINT('',(-0.117775,1.13296574333067E-13,-3.06008671147362));
#45497=CARTESIAN_POINT('Ctrl Pts',(-0.117882453427845,-8.67389818699172E-5,
-1.98508671147362));
#45498=CARTESIAN_POINT('Ctrl Pts',(-0.117927594753219,-0.00555643476035982,
-1.98471615533101));
#45499=CARTESIAN_POINT('Ctrl Pts',(-0.115094354639881,-0.0500818457912055,
-1.98169650208576));
#45500=CARTESIAN_POINT('Ctrl Pts',(-0.058357257409372,-0.126438698298729,
-1.97602775173786));
#45501=CARTESIAN_POINT('Ctrl Pts',(0.0747095887255279,-0.117519322974067,
-1.9680804604299));
#45502=CARTESIAN_POINT('Ctrl Pts',(0.139253915509176,-0.000812979202544665,
-1.96013316912196));
#45503=CARTESIAN_POINT('Ctrl Pts',(0.0760766300741984,0.116639016955623,
-1.952185877814));
#45504=CARTESIAN_POINT('Ctrl Pts',(-0.0568770046268523,0.127111448203918,
-1.94423858650605));
#45505=CARTESIAN_POINT('Ctrl Pts',(-0.114816601332513,0.0510087171606275,
-1.93853886439259));
#45506=CARTESIAN_POINT('Ctrl Pts',(-0.117920583802556,0.00601988872629186,
-1.93548823938178));
#45507=CARTESIAN_POINT('Ctrl Pts',(-0.117869880861692,9.13799831027641E-5,
-1.93508671147362));
#45508=CARTESIAN_POINT('Ctrl Pts',(-0.117839561452888,9.9972777224025E-5,
-1.97521328852638));
#45509=CARTESIAN_POINT('Ctrl Pts',(-0.117548964242824,-0.0320578308581577,
-1.97303674626962));
#45510=CARTESIAN_POINT('Ctrl Pts',(-0.0872671618046854,-0.103836632251253,
-1.96821110691021));
#45511=CARTESIAN_POINT('Ctrl Pts',(0.0342402540498007,-0.13498117883315,
-1.96073637044814));
#45512=CARTESIAN_POINT('Ctrl Pts',(0.132024751554693,-0.0442919700792729,
-1.95278907914019));
#45513=CARTESIAN_POINT('Ctrl Pts',(0.108718118087273,0.0870211723441102,
-1.94484178783224));
#45514=CARTESIAN_POINT('Ctrl Pts',(-0.0143031501084346,0.138519794735472,
-1.93689449652429));
#45515=CARTESIAN_POINT('Ctrl Pts',(-0.104783611163582,0.0763213888572104,
-1.93035166342234));
#45516=CARTESIAN_POINT('Ctrl Pts',(-0.117610887590767,0.0185103122883274,
-1.92645792742304));
#45517=CARTESIAN_POINT('Ctrl Pts',(-0.117583632441682,1.94776852104391E-5,
-1.92521328852638));
#45518=CARTESIAN_POINT('Origin',(0.,0.,-3.06008671147362));
#45519=CARTESIAN_POINT('',(-0.117595734395081,-4.33641902384193E-5,-2.03508671147362));
#45520=CARTESIAN_POINT('',(-0.117909228031939,-7.4177712346371E-5,-2.02521328852638));
#45521=CARTESIAN_POINT('',(-0.117775,1.13296574333067E-13,-3.06008671147362));
#45522=CARTESIAN_POINT('Ctrl Pts',(-0.117595734395081,-4.33641902384211E-5,
-2.03508671147362));
#45523=CARTESIAN_POINT('Ctrl Pts',(-0.117651765097342,-0.0170145075963943,
-2.03394407128025));
#45524=CARTESIAN_POINT('Ctrl Pts',(-0.106267972168461,-0.073259904947786,
-2.03015233398423));
#45525=CARTESIAN_POINT('Ctrl Pts',(-0.0196177116792869,-0.137867542620766,
-2.02371149958557));
#45526=CARTESIAN_POINT('Ctrl Pts',(0.105292387066522,-0.0911363107968193,
-2.01576420827761));
#45527=CARTESIAN_POINT('Ctrl Pts',(0.133629880429484,0.039183784608208,
-2.00781691696966));
#45528=CARTESIAN_POINT('Ctrl Pts',(0.0394040425810417,0.133565097791645,
-1.99986962566171));
#45529=CARTESIAN_POINT('Ctrl Pts',(-0.0848840258511211,0.106753762101256,
-1.99229289049636));
#45530=CARTESIAN_POINT('Ctrl Pts',(-0.117604880485369,0.0335462910435847,
-1.98736525243366));
#45531=CARTESIAN_POINT('Ctrl Pts',(-0.117882453427845,-8.67389818699172E-5,
-1.98508671147362));
#45532=CARTESIAN_POINT('Ctrl Pts',(-0.117909228031939,-7.41777123463737E-5,
-2.02521328852638));
#45533=CARTESIAN_POINT('Ctrl Pts',(-0.117941722441543,-0.00449283611884619,
-2.02491375932151));
#45534=CARTESIAN_POINT('Ctrl Pts',(-0.115708932072434,-0.0479578416298998,
-2.02196513301398));
#45535=CARTESIAN_POINT('Ctrl Pts',(-0.0617215220226959,-0.124830955118446,
-2.0163674096038));
#45536=CARTESIAN_POINT('Ctrl Pts',(0.0715364240393441,-0.11947741908932,
-2.00842011829585));
#45537=CARTESIAN_POINT('Ctrl Pts',(0.139182230024373,-0.00454097809115471,
-2.0004728269879));
#45538=CARTESIAN_POINT('Ctrl Pts',(0.0791721726471583,0.114560380214585,
-1.99252553567995));
#45539=CARTESIAN_POINT('Ctrl Pts',(-0.0534534194270322,0.128588668194905,
-1.984578244372));
#45540=CARTESIAN_POINT('Ctrl Pts',(-0.114156913744517,0.0531357723352751,
-1.97880749532081));
#45541=CARTESIAN_POINT('Ctrl Pts',(-0.117902653781737,0.00708183857550709,
-1.97568584337227));
#45542=CARTESIAN_POINT('Ctrl Pts',(-0.117839561452888,9.9972777224025E-5,
-1.97521328852638));
#45543=CARTESIAN_POINT('Origin',(0.,0.,-3.06008671147362));
#45544=CARTESIAN_POINT('',(-0.117723193797192,0.000105656000806925,-2.08508671147362));
#45545=CARTESIAN_POINT('',(-0.117609472469646,-5.87439815582097E-5,-2.07521328852638));
#45546=CARTESIAN_POINT('',(-0.117775,1.13296574333067E-13,-3.06008671147362));
#45547=CARTESIAN_POINT('Ctrl Pts',(-0.117723193797192,0.00010565600080692,
-2.08508671147362));
#45548=CARTESIAN_POINT('Ctrl Pts',(-0.117477437827794,-0.028255491134646,
-2.08317198722949));
#45549=CARTESIAN_POINT('Ctrl Pts',(-0.0929469453665676,-0.0962366779196943,
-2.07860816588271));
#45550=CARTESIAN_POINT('Ctrl Pts',(0.0207721664357911,-0.137698333400896,
-2.07139524743328));
#45551=CARTESIAN_POINT('Ctrl Pts',(0.127017504190175,-0.0570864918270448,
-2.06344795612532));
#45552=CARTESIAN_POINT('Ctrl Pts',(0.116764283495866,0.0758842277388233,
-2.05550066481737));
#45553=CARTESIAN_POINT('Ctrl Pts',(-0.000583394708775192,0.139255066588021,
-2.04755337350942));
#45554=CARTESIAN_POINT('Ctrl Pts',(-0.100600990582941,0.0841555705722101,
-2.04074872239483));
#45555=CARTESIAN_POINT('Ctrl Pts',(-0.117521863513378,0.022331392440132,
-2.0365931683829));
#45556=CARTESIAN_POINT('Ctrl Pts',(-0.117595734395081,-4.33641902384211E-5,
-2.03508671147362));
#45557=CARTESIAN_POINT('Ctrl Pts',(-0.117609472469646,-5.87439815582062E-5,
-2.07521328852638));
#45558=CARTESIAN_POINT('Ctrl Pts',(-0.11768113966839,-0.0159703079548739,
-2.07414167527074));
#45559=CARTESIAN_POINT('Ctrl Pts',(-0.107255162124516,-0.0711262908138071,
-2.07042096491246));
#45560=CARTESIAN_POINT('Ctrl Pts',(-0.0233018516916921,-0.1372928889066,
-2.06405115745151));
#45561=CARTESIAN_POINT('Ctrl Pts',(0.102814620106721,-0.0939226678118359,
-2.05610386614357));
#45562=CARTESIAN_POINT('Ctrl Pts',(0.134631057384304,0.035592021917362,
-2.04815657483561));
#45563=CARTESIAN_POINT('Ctrl Pts',(0.0429658988952774,0.132462240539342,
-2.04020928352766));
#45564=CARTESIAN_POINT('Ctrl Pts',(-0.0831668745964641,0.108768066411958,
-2.03256152142458));
#45565=CARTESIAN_POINT('Ctrl Pts',(-0.117654335285522,0.0345866759678852,
-2.02756285642416));
#45566=CARTESIAN_POINT('Ctrl Pts',(-0.117909228031939,-7.41777123463737E-5,
-2.02521328852638));
#45567=CARTESIAN_POINT('Origin',(0.,0.,-3.06008671147362));
#45568=CARTESIAN_POINT('',(-0.117967850519022,-1.0412081018357E-5,-2.13508671147362));
#45569=CARTESIAN_POINT('',(-0.117693964354226,0.000100292661075557,-2.12521328852638));
#45570=CARTESIAN_POINT('',(-0.117775,1.13296574333067E-13,-3.06008671147362));
#45571=CARTESIAN_POINT('Ctrl Pts',(-0.117967850519022,-1.04120810183751E-5,
-2.13508671147362));
#45572=CARTESIAN_POINT('Ctrl Pts',(-0.117968551785685,-0.000565995771811528,
-2.13504900028137));
#45573=CARTESIAN_POINT('Ctrl Pts',(-0.117713150989245,-0.0401489893130429,
-2.13236219198648));
#45574=CARTESIAN_POINT('Ctrl Pts',(-0.0737223134758439,-0.118141163087173,
-2.12702628658893));
#45575=CARTESIAN_POINT('Ctrl Pts',(0.0594145941073171,-0.125945305299099,
-2.11907899528099));
#45576=CARTESIAN_POINT('Ctrl Pts',(0.138057323045987,-0.0182342938771007,
-2.11113170397303));
#45577=CARTESIAN_POINT('Ctrl Pts',(0.0900759365079238,0.106200939647636,
-2.10318441266508));
#45578=CARTESIAN_POINT('Ctrl Pts',(-0.0405217541450246,0.133230256926986,
-2.09523712135713));
#45579=CARTESIAN_POINT('Ctrl Pts',(-0.111443182865655,0.060991274530224,
-2.08920455429331));
#45580=CARTESIAN_POINT('Ctrl Pts',(-0.117817450980334,0.010983283291857,
-2.08582108433214));
#45581=CARTESIAN_POINT('Ctrl Pts',(-0.117723193797192,0.00010565600080692,
-2.08508671147362));
#45582=CARTESIAN_POINT('Ctrl Pts',(-0.117693964354226,0.000100292661075554,
-2.12521328852638));
#45583=CARTESIAN_POINT('Ctrl Pts',(-0.117473453135155,-0.0272259720969255,
-2.12336959121998));
#45584=CARTESIAN_POINT('Ctrl Pts',(-0.0943817212641257,-0.0941517958408477,
-2.11887679681093));
#45585=CARTESIAN_POINT('Ctrl Pts',(0.0170780778737081,-0.138205111673633,
-2.11173490529922));
#45586=CARTESIAN_POINT('Ctrl Pts',(0.125443576141085,-0.0604667085388119,
-2.10378761399128));
#45587=CARTESIAN_POINT('Ctrl Pts',(0.118754099267359,0.0727308568888059,
-2.09584032268332));
#45588=CARTESIAN_POINT('Ctrl Pts',(0.00314513556600165,0.139220766262987,
-2.08789303137537));
#45589=CARTESIAN_POINT('Ctrl Pts',(-0.0993708103736951,0.0862718543664017,
-2.08101735332306));
#45590=CARTESIAN_POINT('Ctrl Pts',(-0.117503973729512,0.0233641047155024,
-2.07679077237339));
#45591=CARTESIAN_POINT('Ctrl Pts',(-0.117609472469646,-5.87439815582062E-5,
-2.07521328852638));
#45592=CARTESIAN_POINT('Origin',(0.,0.,-3.06008671147362));
#45593=CARTESIAN_POINT('',(-0.117692226381986,-9.98710273162283E-5,-2.18508671147362));
#45594=CARTESIAN_POINT('',(-0.11796809735242,9.20234616148905E-6,-2.17521328852638));
#45595=CARTESIAN_POINT('',(-0.117775,1.13296574333067E-13,-3.06008671147362));
#45596=CARTESIAN_POINT('Ctrl Pts',(-0.117692226381986,-9.98710273162218E-5,
-2.18508671147362));
#45597=CARTESIAN_POINT('Ctrl Pts',(-0.117788571289341,-0.0121026577886401,
-2.18427691623061));
#45598=CARTESIAN_POINT('Ctrl Pts',(-0.110576187009896,-0.063257325136989,
-2.18081802388496));
#45599=CARTESIAN_POINT('Ctrl Pts',(-0.0367176736873534,-0.134328427217807,
-2.17471003443665));
#45600=CARTESIAN_POINT('Ctrl Pts',(0.093058792097453,-0.103597177245249,
-2.16676274312869));
#45601=CARTESIAN_POINT('Ctrl Pts',(0.137483123155237,0.022151856971875,
-2.15881545182074));
#45602=CARTESIAN_POINT('Ctrl Pts',(0.0558099863031745,0.127583538705665,
-2.1508681605128));
#45603=CARTESIAN_POINT('Ctrl Pts',(-0.0764207885802381,0.116052481208713,
-2.14295858039708));
#45604=CARTESIAN_POINT('Ctrl Pts',(-0.117919289925354,0.0384620767452394,
-2.13769809738402));
#45605=CARTESIAN_POINT('Ctrl Pts',(-0.117967850519022,-1.04120810183751E-5,
-2.13508671147362));
#45606=CARTESIAN_POINT('Ctrl Pts',(-0.11796809735242,9.20234616149382E-6,
-2.17521328852638));
#45607=CARTESIAN_POINT('Ctrl Pts',(-0.117924925187486,-0.0385278244848899,
-2.17259750716922));
#45608=CARTESIAN_POINT('Ctrl Pts',(-0.0763018717954651,-0.116172667440745,
-2.1673326287094));
#45609=CARTESIAN_POINT('Ctrl Pts',(0.0560213207628474,-0.127490883033133,
-2.15941865314694));
#45610=CARTESIAN_POINT('Ctrl Pts',(0.137519639994184,-0.0219240108659811,
-2.15147136183898));
#45611=CARTESIAN_POINT('Ctrl Pts',(0.0928869986161953,0.103751236737962,
-2.14352407053103));
#45612=CARTESIAN_POINT('Ctrl Pts',(-0.0369402110727147,0.134267399030759,
-2.13557677922308));
#45613=CARTESIAN_POINT('Ctrl Pts',(-0.110627789111854,0.0631252406314027,
-2.12947318522153));
#45614=CARTESIAN_POINT('Ctrl Pts',(-0.117790292363326,0.01203748429871,
-2.12601868832263));
#45615=CARTESIAN_POINT('Ctrl Pts',(-0.117693964354226,0.000100292661075554,
-2.12521328852638));
#45616=CARTESIAN_POINT('Origin',(0.,0.,-3.06008671147362));
#45617=CARTESIAN_POINT('',(-0.117610460329433,5.96508612474619E-5,-2.23508671147362));
#45618=CARTESIAN_POINT('',(-0.117721328622872,-0.000105405280874327,-2.22521328852638));
#45619=CARTESIAN_POINT('',(-0.117775,1.13296574333067E-13,-3.06008671147362));
#45620=CARTESIAN_POINT('Ctrl Pts',(-0.117610460329433,5.96508612474792E-5,
-2.23508671147362));
#45621=CARTESIAN_POINT('Ctrl Pts',(-0.117502981482352,-0.0234279695405327,
-2.23350483217985));
#45622=CARTESIAN_POINT('Ctrl Pts',(-0.0992933102918214,-0.0864026580678686,
-2.22927385578343));
#45623=CARTESIAN_POINT('Ctrl Pts',(0.00337582615670157,-0.139215364516925,
-2.22239378228436));
#45624=CARTESIAN_POINT('Ctrl Pts',(0.118874455301411,-0.0725339768426726,
-2.21444649097641));
#45625=CARTESIAN_POINT('Ctrl Pts',(0.125343208860993,0.0606744914461575,
-2.20649919966845));
#45626=CARTESIAN_POINT('Ctrl Pts',(0.0168490426502724,0.138233222061811,
-2.19855190836051));
#45627=CARTESIAN_POINT('Ctrl Pts',(-0.0944690535724636,0.0940224986942619,
-2.19141441229555));
#45628=CARTESIAN_POINT('Ctrl Pts',(-0.117473396537287,0.0271622649282534,
-2.18692601333326));
#45629=CARTESIAN_POINT('Ctrl Pts',(-0.117692226381986,-9.98710273162218E-5,
-2.18508671147362));
#45630=CARTESIAN_POINT('Ctrl Pts',(-0.117721328622872,-0.00010540528087433,
-2.22521328852638));
#45631=CARTESIAN_POINT('Ctrl Pts',(-0.117815809071607,-0.0110485780997072,
-2.2244745202211));
#45632=CARTESIAN_POINT('Ctrl Pts',(-0.111393725741073,-0.0611233075246441,
-2.22108665481318));
#45633=CARTESIAN_POINT('Ctrl Pts',(-0.0403009298698327,-0.133297219356626,
-2.2150496923026));
#45634=CARTESIAN_POINT('Ctrl Pts',(0.0902517917743938,-0.106051533313259,
-2.20710240099464));
#45635=CARTESIAN_POINT('Ctrl Pts',(0.13802691747888,0.0184630357162695,
-2.19915510968669));
#45636=CARTESIAN_POINT('Ctrl Pts',(0.059205815238823,0.12604358404333,-2.19120781837874));
#45637=CARTESIAN_POINT('Ctrl Pts',(-0.0739179767846482,0.118018838939578,
-2.18326052707079));
#45638=CARTESIAN_POINT('Ctrl Pts',(-0.117743386247816,0.0400181840074988,
-2.17792901712));
#45639=CARTESIAN_POINT('Ctrl Pts',(-0.11796864721216,0.00050002692296339,
-2.17524660427187));
#45640=CARTESIAN_POINT('Ctrl Pts',(-0.11796809735242,9.20234616149382E-6,
-2.17521328852638));
#45641=CARTESIAN_POINT('Origin',(0.,0.,-3.06008671147362));
#45642=CARTESIAN_POINT('',(-0.117910775228005,7.33173023513087E-5,-2.28508671147362));
#45643=CARTESIAN_POINT('',(-0.117596460302673,4.43517738773561E-5,-2.27521328852638));
#45644=CARTESIAN_POINT('',(-0.117775,1.13296574333067E-13,-3.06008671147362));
#45645=CARTESIAN_POINT('Ctrl Pts',(-0.117910775228005,7.33173023513014E-5,
-2.28508671147362));
#45646=CARTESIAN_POINT('Ctrl Pts',(-0.117657693388436,-0.0346511833667682,
-2.28273274812909));
#45647=CARTESIAN_POINT('Ctrl Pts',(-0.0830590431455795,-0.108892231259704,
-2.2777296876819));
#45648=CARTESIAN_POINT('Ctrl Pts',(0.0431853359348615,-0.132390863279962,
-2.27007753013206));
#45649=CARTESIAN_POINT('Ctrl Pts',(0.134689851066473,-0.0353688837753169,
-2.26213023882412));
#45650=CARTESIAN_POINT('Ctrl Pts',(0.102658845743989,0.0940929078641549,
-2.25418294751616));
#45651=CARTESIAN_POINT('Ctrl Pts',(-0.0235293201795658,0.137254089234922,
-2.24623565620821));
#45652=CARTESIAN_POINT('Ctrl Pts',(-0.107315019292188,0.0709942209893211,
-2.23987024419403));
#45653=CARTESIAN_POINT('Ctrl Pts',(-0.117682971133598,0.015905617667775,
-2.2361539292825));
#45654=CARTESIAN_POINT('Ctrl Pts',(-0.117610460329433,5.96508612474792E-5,
-2.23508671147362));
#45655=CARTESIAN_POINT('Ctrl Pts',(-0.117596460302673,4.43517738773439E-5,
-2.27521328852638));
#45656=CARTESIAN_POINT('Ctrl Pts',(-0.117520659904767,-0.0223953420072019,
-2.27370243617034));
#45657=CARTESIAN_POINT('Ctrl Pts',(-0.100526067276438,-0.0842866703776684,
-2.26954248671165));
#45658=CARTESIAN_POINT('Ctrl Pts',(-0.00035264218412894,-0.139255841098576,
-2.2627334401503));
#45659=CARTESIAN_POINT('Ctrl Pts',(0.116889865813058,-0.0756906394925223,
-2.25478614884235));
#45660=CARTESIAN_POINT('Ctrl Pts',(0.126922734073552,0.0572968865810018,
-2.2468388575344));
#45661=CARTESIAN_POINT('Ctrl Pts',(0.020543965621383,0.137732563735411,
-2.23889156622645));
#45662=CARTESIAN_POINT('Ctrl Pts',(-0.09303702865732,0.0961079088722858,
-2.23168304322378));
#45663=CARTESIAN_POINT('Ctrl Pts',(-0.117477018301604,0.028191772631412,
-2.22712361732375));
#45664=CARTESIAN_POINT('Ctrl Pts',(-0.117721328622872,-0.00010540528087433,
-2.22521328852638));
#45665=CARTESIAN_POINT('Origin',(0.,0.,-3.06008671147362));
#45666=CARTESIAN_POINT('',(-0.117837633641763,-0.000100407954100913,-2.33508671147362));
#45667=CARTESIAN_POINT('',(-0.117884197500364,8.6037916559329E-5,-2.32521328852638));
#45668=CARTESIAN_POINT('',(-0.117775,1.13296574333067E-13,-3.06008671147362));
#45669=CARTESIAN_POINT('Ctrl Pts',(-0.117837633641763,-0.000100407954100916,
-2.33508671147362));
#45670=CARTESIAN_POINT('Ctrl Pts',(-0.117901463481007,-0.00714751330050535,
-2.33460976118097));
#45671=CARTESIAN_POINT('Ctrl Pts',(-0.114115041181782,-0.0532674687213532,
-2.33148371378567));
#45672=CARTESIAN_POINT('Ctrl Pts',(-0.0532402693961469,-0.128677067243725,
-2.32570856928773));
#45673=CARTESIAN_POINT('Ctrl Pts',(0.0793618960797965,-0.114429032026143,
-2.31776127797978));
#45674=CARTESIAN_POINT('Ctrl Pts',(0.139174515358953,0.00477160291947143,
-2.30981398667182));
#45675=CARTESIAN_POINT('Ctrl Pts',(0.0713383470518088,0.11959579490825,
-2.30186669536388));
#45676=CARTESIAN_POINT('Ctrl Pts',(-0.0619282880767048,0.124728509394241,
-2.29391940405591));
#45677=CARTESIAN_POINT('Ctrl Pts',(-0.115745950361329,0.0478264738904903,
-2.2883260760925));
#45678=CARTESIAN_POINT('Ctrl Pts',(-0.117942505966122,0.00442698423816777,
-2.28538184523174));
#45679=CARTESIAN_POINT('Ctrl Pts',(-0.117910775228005,7.33173023513014E-5,
-2.28508671147362));
#45680=CARTESIAN_POINT('Ctrl Pts',(-0.117884197500364,8.60379165593343E-5,
-2.32521328852638));
#45681=CARTESIAN_POINT('Ctrl Pts',(-0.117607682544816,-0.0336105716919928,
-2.32293035211958));
#45682=CARTESIAN_POINT('Ctrl Pts',(-0.0847791412331816,-0.106878836889164,
-2.31799831861012));
#45683=CARTESIAN_POINT('Ctrl Pts',(0.0396253113885193,-0.133499619227714,
-2.31041718799801));
#45684=CARTESIAN_POINT('Ctrl Pts',(0.13369462523368,-0.0389622999861087,
-2.30246989669006));
#45685=CARTESIAN_POINT('Ctrl Pts',(0.105141224899681,0.0913106590885011,
-2.29452260538211));
#45686=CARTESIAN_POINT('Ctrl Pts',(-0.0198461371346163,0.137834844931954,
-2.28657531407416));
#45687=CARTESIAN_POINT('Ctrl Pts',(-0.106330160380951,0.0731279015670244,
-2.28013887512225));
#45688=CARTESIAN_POINT('Ctrl Pts',(-0.117653566746173,0.0169499504312584,
-2.27635153327299));
#45689=CARTESIAN_POINT('Ctrl Pts',(-0.117596460302673,4.43517738773439E-5,
-2.27521328852638));
#45690=CARTESIAN_POINT('Origin',(0.,0.,-3.06008671147362));
#45691=CARTESIAN_POINT('',(-0.117583321031667,-1.84167202121336E-5,-2.38508671147362));
#45692=CARTESIAN_POINT('',(-0.117868059206978,-9.19955489654817E-5,-2.37521328852638));
#45693=CARTESIAN_POINT('',(-0.117775,1.13296574333067E-13,-3.06008671147362));
#45694=CARTESIAN_POINT('Ctrl Pts',(-0.117583321031667,-1.84167202121367E-5,
-2.38508671147362));
#45695=CARTESIAN_POINT('Ctrl Pts',(-0.117609178758956,-0.0185746748110054,
-2.38383767713021));
#45696=CARTESIAN_POINT('Ctrl Pts',(-0.104717853734675,-0.0764532318113364,
-2.37993954568415));
#45697=CARTESIAN_POINT('Ctrl Pts',(-0.0140735972308577,-0.138543306517508,
-2.37339231713544));
#45698=CARTESIAN_POINT('Ctrl Pts',(0.10886216750279,-0.086840902842008,
-2.36544502582749));
#45699=CARTESIAN_POINT('Ctrl Pts',(0.13195117753492,0.044510680369643,-2.35749773451953));
#45700=CARTESIAN_POINT('Ctrl Pts',(0.0340165375872002,0.135037732098843,
-2.34955044321158));
#45701=CARTESIAN_POINT('Ctrl Pts',(-0.0873676836443551,0.103710317580185,
-2.34208010219627));
#45702=CARTESIAN_POINT('Ctrl Pts',(-0.11754693713977,0.0319938115777102,
-2.33725885828362));
#45703=CARTESIAN_POINT('Ctrl Pts',(-0.117837633641763,-0.000100407954100916,
-2.33508671147362));
#45704=CARTESIAN_POINT('Ctrl Pts',(-0.117868059206978,-9.19955489654947E-5,
-2.37521328852638));
#45705=CARTESIAN_POINT('Ctrl Pts',(-0.117919547374431,-0.00608564309425205,
-2.37480736517147));
#45706=CARTESIAN_POINT('Ctrl Pts',(-0.114776697578318,-0.0511402889575705,
-2.3717523447139));
#45707=CARTESIAN_POINT('Ctrl Pts',(-0.0566662969110845,-0.127205520442183,
-2.36604822715368));
#45708=CARTESIAN_POINT('Ctrl Pts',(0.0762698010119113,-0.116512793675996,
-2.35810093584572));
#45709=CARTESIAN_POINT('Ctrl Pts',(0.13925237616884,0.00104372789252618,
-2.35015364453777));
#45710=CARTESIAN_POINT('Ctrl Pts',(0.0745147509671164,0.117642957821071,
-2.34220635322982));
#45711=CARTESIAN_POINT('Ctrl Pts',(-0.0585666913028059,0.126341823266975,
-2.33425906192187));
#45712=CARTESIAN_POINT('Ctrl Pts',(-0.115133288835063,0.0499503388447956,
-2.32859470702072));
#45713=CARTESIAN_POINT('Ctrl Pts',(-0.117928547797741,0.00549064488900448,
-2.32557944922223));
#45714=CARTESIAN_POINT('Ctrl Pts',(-0.117884197500364,8.60379165593343E-5,
-2.32521328852638));
#45715=CARTESIAN_POINT('Origin',(0.,0.,-3.06008671147362));
#45716=CARTESIAN_POINT('',(-0.117769879638916,0.000108303546025554,-2.43508671147362));
#45717=CARTESIAN_POINT('',(-0.117590495046852,-3.52740045776734E-5,-2.42521328852638));
#45718=CARTESIAN_POINT('',(-0.117775,1.13296574333067E-13,-3.06008671147362));
#45719=CARTESIAN_POINT('Ctrl Pts',(-0.117769879638916,0.000108303546025553,
-2.43508671147362));
#45720=CARTESIAN_POINT('Ctrl Pts',(-0.117495009512743,-0.0297985645403461,
-2.43306559307944));
#45721=CARTESIAN_POINT('Ctrl Pts',(-0.0907137933584123,-0.0993425203592325,
-2.42839537758262));
#45722=CARTESIAN_POINT('Ctrl Pts',(0.0262770108420999,-0.136754643873708,
-2.42107606498315));
#45723=CARTESIAN_POINT('Ctrl Pts',(0.129204451314017,-0.0519473163932888,
-2.41312877367519));
#45724=CARTESIAN_POINT('Ctrl Pts',(0.113627498086771,0.0805053141001346,
-2.40518148236725));
#45725=CARTESIAN_POINT('Ctrl Pts',(-0.00616689990636303,0.139119672459956,
-2.39723419105929));
#45726=CARTESIAN_POINT('Ctrl Pts',(-0.102366602030147,0.0809774201074958,
-2.39053593409475));
#45727=CARTESIAN_POINT('Ctrl Pts',(-0.117554336687715,0.0207815925356226,
-2.38648677423286));
#45728=CARTESIAN_POINT('Ctrl Pts',(-0.117583321031667,-1.84167202121367E-5,
-2.38508671147362));
#45729=CARTESIAN_POINT('Ctrl Pts',(-0.117590495046852,-3.52740045776734E-5,
-2.42521328852638));
#45730=CARTESIAN_POINT('Ctrl Pts',(-0.117637364608106,-0.0175336573692995,
-2.4240352811207));
#45731=CARTESIAN_POINT('Ctrl Pts',(-0.105762263505043,-0.0743218437255907,
-2.42020817661237));
#45732=CARTESIAN_POINT('Ctrl Pts',(-0.0177778171272468,-0.138116844934903,
-2.41373197500138));
#45733=CARTESIAN_POINT('Ctrl Pts',(0.106498123211473,-0.0897243745534934,
-2.40578468369343));
#45734=CARTESIAN_POINT('Ctrl Pts',(0.133095574977059,0.0409619525670818,
-2.39783739238548));
#45735=CARTESIAN_POINT('Ctrl Pts',(0.0376197525149271,0.134078588362562,
-2.38989010107753));
#45736=CARTESIAN_POINT('Ctrl Pts',(-0.08572135907778,0.105745412574563,
-2.3823487331245));
#45737=CARTESIAN_POINT('Ctrl Pts',(-0.117583530356522,0.0330295104295094,
-2.37745646227412));
#45738=CARTESIAN_POINT('Ctrl Pts',(-0.117868059206978,-9.19955489654947E-5,
-2.37521328852638));
#45739=CARTESIAN_POINT('Origin',(0.,0.,-3.06008671147362));
#45740=CARTESIAN_POINT('',(-0.117953497684312,-3.88090381494036E-5,-2.48508671147362));
#45741=CARTESIAN_POINT('',(-0.11773841333479,0.000107271409016091,-2.47521328852638));
#45742=CARTESIAN_POINT('',(-0.117775,1.13296574333067E-13,-3.06008671147362));
#45743=CARTESIAN_POINT('Ctrl Pts',(-0.117953497684312,-3.88090381494167E-5,
-2.48508671147362));
#45744=CARTESIAN_POINT('Ctrl Pts',(-0.117962605253777,-0.00216254596668706,
-2.48494260613133));
#45745=CARTESIAN_POINT('Ctrl Pts',(-0.116947344620421,-0.0433181804821695,
-2.4821494036864));
#45746=CARTESIAN_POINT('Ctrl Pts',(-0.0689256895917136,-0.121002327391366,
-2.47670710413881));
#45747=CARTESIAN_POINT('Ctrl Pts',(0.0644170755712456,-0.123461549863384,
-2.46875981283085));
#45748=CARTESIAN_POINT('Ctrl Pts',(0.138677460778961,-0.0126836821041933,
-2.46081252152291));
#45749=CARTESIAN_POINT('Ctrl Pts',(0.0857449494400285,0.109727469511273,
-2.45286523021495));
#45750=CARTESIAN_POINT('Ctrl Pts',(-0.0458315493375432,0.131498224342159,
-2.444917938907));
#45751=CARTESIAN_POINT('Ctrl Pts',(-0.112600512780524,0.0577966553949038,
-2.43899176599322));
#45752=CARTESIAN_POINT('Ctrl Pts',(-0.117855284129485,0.00940062231845771,
-2.43571469018209));
#45753=CARTESIAN_POINT('Ctrl Pts',(-0.117769879638916,0.000108303546025553,
-2.43508671147362));
#45754=CARTESIAN_POINT('Ctrl Pts',(-0.11773841333479,0.00010727140901609,
-2.47521328852638));
#45755=CARTESIAN_POINT('Ctrl Pts',(-0.117481668772501,-0.0287682554493046,
-2.47326319706994));
#45756=CARTESIAN_POINT('Ctrl Pts',(-0.0922158471109609,-0.0972715125940092,
-2.46866400851084));
#45757=CARTESIAN_POINT('Ctrl Pts',(0.0226062146261162,-0.137409143425246,
-2.46141572284909));
#45758=CARTESIAN_POINT('Ctrl Pts',(0.127767332108225,-0.0553879272272235,
-2.45346843154115));
#45759=CARTESIAN_POINT('Ctrl Pts',(0.115742160170272,0.0774342688717387,
-2.44552114023319));
#45760=CARTESIAN_POINT('Ctrl Pts',(-0.00243999302426519,0.139234909669319,
-2.43757384892524));
#45761=CARTESIAN_POINT('Ctrl Pts',(-0.101198093853741,0.0831000893788111,
-2.43080456502297));
#45762=CARTESIAN_POINT('Ctrl Pts',(-0.117531964575542,0.0218166187401381,
-2.42668437822335));
#45763=CARTESIAN_POINT('Ctrl Pts',(-0.117590495046852,-3.52740045776734E-5,
-2.42521328852638));
#45764=CARTESIAN_POINT('Origin',(0.,0.,-3.06008671147362));
#45765=CARTESIAN_POINT('',(-0.117653224368514,-8.67076276465346E-5,-2.53508671147362));
#45766=CARTESIAN_POINT('',(-0.117964807649162,-2.00728089981839E-5,-2.52521328852639));
#45767=CARTESIAN_POINT('',(-0.117775,1.13296574333067E-13,-3.06008671147362));
#45768=CARTESIAN_POINT('Ctrl Pts',(-0.117653224368514,-8.67076276465321E-5,
-2.53508671147362));
#45769=CARTESIAN_POINT('Ctrl Pts',(-0.117745757901207,-0.0136778186926029,
-2.53417052208057));
#45770=CARTESIAN_POINT('Ctrl Pts',(-0.109285840550885,-0.0664550385671571,
-2.53060523558487));
#45771=CARTESIAN_POINT('Ctrl Pts',(-0.0313017206303005,-0.135692727164734,
-2.52439085198651));
#45772=CARTESIAN_POINT('Ctrl Pts',(0.0971380788063926,-0.0997823008635477,
-2.51644356067857));
#45773=CARTESIAN_POINT('Ctrl Pts',(0.136484282651119,0.0276469620217102,
-2.50849626937061));
#45774=CARTESIAN_POINT('Ctrl Pts',(0.0506491401835047,0.129718844114848,
-2.50054897806267));
#45775=CARTESIAN_POINT('Ctrl Pts',(-0.0792418750448042,0.113121058725188,
-2.49274579209699));
#45776=CARTESIAN_POINT('Ctrl Pts',(-0.117795180261066,0.0368782366644444,
-2.48759170323398));
#45777=CARTESIAN_POINT('Ctrl Pts',(-0.117953497684312,-3.88090381494167E-5,
-2.48508671147362));
#45778=CARTESIAN_POINT('Ctrl Pts',(-0.117964807649162,-2.00728089981873E-5,
-2.52521328852638));
#45779=CARTESIAN_POINT('Ctrl Pts',(-0.117967343283893,-0.00109678191988592,
-2.52514021012183));
#45780=CARTESIAN_POINT('Ctrl Pts',(-0.117465836079,-0.0412018472256403,
-2.52241803461462));
#45781=CARTESIAN_POINT('Ctrl Pts',(-0.0721406159404224,-0.119113580956658,
-2.51704676200475));
#45782=CARTESIAN_POINT('Ctrl Pts',(0.0610885073433754,-0.125141951028183,
-2.50909947069681));
#45783=CARTESIAN_POINT('Ctrl Pts',(0.1382881637544,-0.0163919920088414,
-2.50115217938885));
#45784=CARTESIAN_POINT('Ctrl Pts',(0.0886519810374287,0.107392457345575,
-2.4932048880809));
#45785=CARTESIAN_POINT('Ctrl Pts',(-0.0422944750968055,0.132678148211631,
-2.48525759677295));
#45786=CARTESIAN_POINT('Ctrl Pts',(-0.111836348204514,0.0599290334960457,
-2.47926039692144));
#45787=CARTESIAN_POINT('Ctrl Pts',(-0.11783044281273,0.0104576353595844,
-2.47591229417259));
#45788=CARTESIAN_POINT('Ctrl Pts',(-0.11773841333479,0.00010727140901609,
-2.47521328852638));
#45789=CARTESIAN_POINT('Origin',(0.,0.,-3.06008671147362));
#45790=CARTESIAN_POINT('',(-0.117638891309021,7.96281316254408E-5,-2.58508671147362));
#45791=CARTESIAN_POINT('',(-0.117678576059632,-9.61137264129941E-5,-2.57521328852638));
#45792=CARTESIAN_POINT('',(-0.117775,1.13296574333067E-13,-3.06008671147362));
#45793=CARTESIAN_POINT('Ctrl Pts',(-0.117638891309021,7.96281316254328E-5,
-2.58508671147362));
#45794=CARTESIAN_POINT('Ctrl Pts',(-0.117483508336674,-0.0249725458388271,
-2.58339843802981));
#45795=CARTESIAN_POINT('Ctrl Pts',(-0.0973679568000036,-0.0895623381818424,
-2.57906106748334));
#45796=CARTESIAN_POINT('Ctrl Pts',(0.00895549343668939,-0.138968028902788,
-2.57207459983422));
#45797=CARTESIAN_POINT('Ctrl Pts',(0.121687378843393,-0.0677089045107432,
-2.56412730852628));
#45798=CARTESIAN_POINT('Ctrl Pts',(0.122809417189726,0.0656518161922446,
-2.55618001721832));
#45799=CARTESIAN_POINT('Ctrl Pts',(0.011292491656669,0.138797671277311,
-2.54823272591037));
#45800=CARTESIAN_POINT('Ctrl Pts',(-0.096531683990788,0.0908838025098833,
-2.54120162399547));
#45801=CARTESIAN_POINT('Ctrl Pts',(-0.117478203708577,0.0256199217277792,
-2.53681961918322));
#45802=CARTESIAN_POINT('Ctrl Pts',(-0.117653224368514,-8.67076276465321E-5,
-2.53508671147362));
#45803=CARTESIAN_POINT('Ctrl Pts',(-0.117678576059632,-9.61137264130253E-5,
-2.57521328852638));
#45804=CARTESIAN_POINT('Ctrl Pts',(-0.117774563927174,-0.0126267819892236,
-2.57436812607106));
#45805=CARTESIAN_POINT('Ctrl Pts',(-0.110156077978415,-0.0643201985882453,
-2.57087386651309));
#45806=CARTESIAN_POINT('Ctrl Pts',(-0.0349234451532213,-0.134806033304195,
-2.56473050985246));
#45807=CARTESIAN_POINT('Ctrl Pts',(0.0944317530776,-0.102347240545473,-2.55678321854452));
#45808=CARTESIAN_POINT('Ctrl Pts',(0.137175557268965,0.0239829131785638,
-2.54883592723656));
#45809=CARTESIAN_POINT('Ctrl Pts',(0.0541039883893578,0.128316297004496,
-2.54088863592861));
#45810=CARTESIAN_POINT('Ctrl Pts',(-0.077370769783318,0.11508270631958,
-2.53301442302521));
#45811=CARTESIAN_POINT('Ctrl Pts',(-0.117875426353606,0.0379339960955099,
-2.52778930722448));
#45812=CARTESIAN_POINT('Ctrl Pts',(-0.117964807649162,-2.00728089981873E-5,
-2.52521328852638));
#45813=CARTESIAN_POINT('Origin',(0.,0.,-3.06008671147362));
#45814=CARTESIAN_POINT('',(-0.117943238001422,4.98985662682079E-5,-2.63508671147362));
#45815=CARTESIAN_POINT('',(-0.117618959460295,6.6729458887721E-5,-2.62521328852638));
#45816=CARTESIAN_POINT('',(-0.117775,1.13296574333067E-13,-3.06008671147362));
#45817=CARTESIAN_POINT('Ctrl Pts',(-0.117943238001422,4.98985662681943E-5,
-2.63508671147362));
#45818=CARTESIAN_POINT('Ctrl Pts',(-0.117749962726917,-0.0362177372561391,
-2.63262635397904));
#45819=CARTESIAN_POINT('Ctrl Pts',(-0.0803927491711805,-0.111879153836378,
-2.62751689938181));
#45820=CARTESIAN_POINT('Ctrl Pts',(0.0484593300923006,-0.130552699117355,
-2.61975834768194));
#45821=CARTESIAN_POINT('Ctrl Pts',(0.135999775339708,-0.0299395228313577,
-2.61181105637398));
#45822=CARTESIAN_POINT('Ctrl Pts',(0.0988032571470193,0.0981337367930133,
-2.60386376506603));
#45823=CARTESIAN_POINT('Ctrl Pts',(-0.0290141333502425,0.136200198185447,
-2.59591647375808));
#45824=CARTESIAN_POINT('Ctrl Pts',(-0.108720603964012,0.0677966676599294,
-2.58965745589394));
#45825=CARTESIAN_POINT('Ctrl Pts',(-0.117727322265842,0.0143372245798384,
-2.58604753513246));
#45826=CARTESIAN_POINT('Ctrl Pts',(-0.117638891309021,7.96281316254328E-5,
-2.58508671147362));
#45827=CARTESIAN_POINT('Ctrl Pts',(-0.117618959460295,6.6729458887714E-5,
-2.62521328852638));
#45828=CARTESIAN_POINT('Ctrl Pts',(-0.117495510368196,-0.0239416772140386,
-2.6235960420203));
#45829=CARTESIAN_POINT('Ctrl Pts',(-0.0986638469305919,-0.0874544040157706,
-2.61932969841156));
#45830=CARTESIAN_POINT('Ctrl Pts',(0.00523164691012173,-0.139157980393471,
-2.61241425770018));
#45831=CARTESIAN_POINT('Ctrl Pts',(0.119830964215785,-0.0709426081540357,
-2.60446696639222));
#45832=CARTESIAN_POINT('Ctrl Pts',(0.12452311024091,0.0623402650981849,
-2.59651967508427));
#45833=CARTESIAN_POINT('Ctrl Pts',(0.0150045187058493,0.138445577953893,
-2.58857238377632));
#45834=CARTESIAN_POINT('Ctrl Pts',(-0.0951656069162575,0.0929810151014424,
-2.58147025492369));
#45835=CARTESIAN_POINT('Ctrl Pts',(-0.117473697294737,0.0266496396978196,
-2.57701722317371));
#45836=CARTESIAN_POINT('Ctrl Pts',(-0.117678576059632,-9.61137264130253E-5,
-2.57521328852638));
#45837=CARTESIAN_POINT('Origin',(0.,0.,-3.06008671147362));
#45838=CARTESIAN_POINT('',(-0.117789991982999,-0.00010740623187117,-2.68508671147362));
#45839=CARTESIAN_POINT('',(-0.11792267289879,6.60661965921575E-5,-2.67521328852638));
#45840=CARTESIAN_POINT('',(-0.117775,1.13296574333067E-13,-3.06008671147362));
#45841=CARTESIAN_POINT('Ctrl Pts',(-0.117789991982999,-0.000107406231871198,
-2.68508671147362));
#45842=CARTESIAN_POINT('Ctrl Pts',(-0.11786993715536,-0.0087354930933903,
-2.68450336703093));
#45843=CARTESIAN_POINT('Ctrl Pts',(-0.113063580952104,-0.0564573476549392,
-2.68127092548559));
#45844=CARTESIAN_POINT('Ctrl Pts',(-0.0480376407722225,-0.130708450334381,
-2.67538938683759));
#45845=CARTESIAN_POINT('Ctrl Pts',(0.0838865444021125,-0.111154674162296,
-2.66744209552965));
#45846=CARTESIAN_POINT('Ctrl Pts',(0.138871243492067,0.0103485095922432,
-2.65949480422169));
#45847=CARTESIAN_POINT('Ctrl Pts',(0.0664853114242254,0.122360194853714,
-2.65154751291374));
#45848=CARTESIAN_POINT('Ctrl Pts',(-0.0668799556441275,0.12214493625552,
-2.64360022160579));
#45849=CARTESIAN_POINT('Ctrl Pts',(-0.116606427544758,0.0446493968714564,
-2.63811328779242));
#45850=CARTESIAN_POINT('Ctrl Pts',(-0.117958064586437,0.00283207123262861,
-2.63527545108169));
#45851=CARTESIAN_POINT('Ctrl Pts',(-0.117943238001422,4.98985662681943E-5,
-2.63508671147362));
#45852=CARTESIAN_POINT('Ctrl Pts',(-0.11792267289879,6.60661965921502E-5,
-2.67521328852638));
#45853=CARTESIAN_POINT('Ctrl Pts',(-0.117685998143791,-0.0351708055618756,
-2.67282395796953));
#45854=CARTESIAN_POINT('Ctrl Pts',(-0.0821847093582401,-0.109889137046738,
-2.66778553031004));
#45855=CARTESIAN_POINT('Ctrl Pts',(0.0449466287065965,-0.131803316363808,
-2.66009800554788));
#45856=CARTESIAN_POINT('Ctrl Pts',(0.135149441973695,-0.0335699563714237,
-2.65215071423994));
#45857=CARTESIAN_POINT('Ctrl Pts',(0.10139520486838,0.0954532663992196,
-2.64420342293198));
#45858=CARTESIAN_POINT('Ctrl Pts',(-0.0253572002932921,0.136928178363215,
-2.63625613162403));
#45859=CARTESIAN_POINT('Ctrl Pts',(-0.107791450141899,0.0699314320822719,
-2.62992608682216));
#45860=CARTESIAN_POINT('Ctrl Pts',(-0.11769772359356,0.0153847954771589,
-2.62624513912295));
#45861=CARTESIAN_POINT('Ctrl Pts',(-0.117618959460295,6.6729458887714E-5,
-2.62521328852638));
#45862=CARTESIAN_POINT('Origin',(0.,0.,-3.06008671147362));
#45863=CARTESIAN_POINT('',(-0.117581146632055,7.56075370698167E-6,-2.73508671147362));
#45864=CARTESIAN_POINT('',(-0.117821958574713,-0.000103490888977639,-2.72521328852638));
#45865=CARTESIAN_POINT('',(-0.117775,1.13296574333067E-13,-3.06008671147362));
#45866=CARTESIAN_POINT('Ctrl Pts',(-0.117581146632055,7.56075370697551E-6,
-2.73508671147362));
#45867=CARTESIAN_POINT('Ctrl Pts',(-0.117569638646798,-0.0201302688798466,
-2.73373128298016));
#45868=CARTESIAN_POINT('Ctrl Pts',(-0.103080207415897,-0.0796417091885475,
-2.72972675738406));
#45869=CARTESIAN_POINT('Ctrl Pts',(-0.00850684444458044,-0.138996214030495,
-2.72307313468531));
#45870=CARTESIAN_POINT('Ctrl Pts',(0.112256835707494,-0.0824058053669272,
-2.71512584337735));
#45871=CARTESIAN_POINT('Ctrl Pts',(0.130060222154785,0.0497659776633264,
-2.70717855206941));
#45872=CARTESIAN_POINT('Ctrl Pts',(0.02857431466928,0.136293148986501,-2.69923126076145));
#45873=CARTESIAN_POINT('Ctrl Pts',(-0.0897465865227608,0.100638692211853,
-2.69186731389619));
#45874=CARTESIAN_POINT('Ctrl Pts',(-0.117506888313243,0.0304465719673242,
-2.68715246413358));
#45875=CARTESIAN_POINT('Ctrl Pts',(-0.117789991982999,-0.000107406231871198,
-2.68508671147362));
#45876=CARTESIAN_POINT('Ctrl Pts',(-0.117821958574713,-0.000103490888977657,
-2.72521328852638));
#45877=CARTESIAN_POINT('Ctrl Pts',(-0.117891546518806,-0.00767575694883443,
-2.72470097102142));
#45878=CARTESIAN_POINT('Ctrl Pts',(-0.113773620055613,-0.0543273988107319,
-2.72153955641381));
#45879=CARTESIAN_POINT('Ctrl Pts',(-0.0515199201897912,-0.12937546699384,
-2.71572904470355));
#45880=CARTESIAN_POINT('Ctrl Pts',(0.0808804927988873,-0.113360749474457,
-2.7077817533956));
#45881=CARTESIAN_POINT('Ctrl Pts',(0.139098525352115,0.0066267549690055,
-2.69983446208764));
#45882=CARTESIAN_POINT('Ctrl Pts',(0.0697374672192116,0.120536298692083,
-2.69188717077969));
#45883=CARTESIAN_POINT('Ctrl Pts',(-0.0635857546542645,0.123891748884511,
-2.68393987947174));
#45884=CARTESIAN_POINT('Ctrl Pts',(-0.116039537486793,0.0467697666635364,
-2.67838191872063));
#45885=CARTESIAN_POINT('Ctrl Pts',(-0.117948404032311,0.00389699718071681,
-2.67547305507218));
#45886=CARTESIAN_POINT('Ctrl Pts',(-0.11792267289879,6.60661965921502E-5,
-2.67521328852638));
#45887=CARTESIAN_POINT('Origin',(0.,0.,-3.06008671147362));
#45888=CARTESIAN_POINT('',(-0.117817815448454,0.000104175268542342,-2.78508671147362));
#45889=CARTESIAN_POINT('',(-0.117581447556463,-9.82433484120193E-6,-2.77521328852638));
#45890=CARTESIAN_POINT('',(-0.117775,1.13296574333067E-13,-3.06008671147362));
#45891=CARTESIAN_POINT('Ctrl Pts',(-0.117817815448454,0.00010417526854233,
-2.78508671147362));
#45892=CARTESIAN_POINT('Ctrl Pts',(-0.117528053916134,-0.0313441947429135,
-2.7829591989294));
#45893=CARTESIAN_POINT('Ctrl Pts',(-0.088378335258817,-0.102424947763681,
-2.77818258928254));
#45894=CARTESIAN_POINT('Ctrl Pts',(0.0317395866552255,-0.135590974706457,
-2.77075688253302));
#45895=CARTESIAN_POINT('Ctrl Pts',(0.131183564369451,-0.0467245803901248,
-2.76280959122507));
#45896=CARTESIAN_POINT('Ctrl Pts',(0.110307935021035,0.0849969022889005,
-2.75486229991711));
#45897=CARTESIAN_POINT('Ctrl Pts',(-0.0117404851910752,0.138760494767705,
-2.74691500860916));
#45898=CARTESIAN_POINT('Ctrl Pts',(-0.104041614331916,0.0777915559561233,
-2.74032314579466));
#45899=CARTESIAN_POINT('Ctrl Pts',(-0.11759213025779,0.01922781337502,-2.73638038008281));
#45900=CARTESIAN_POINT('Ctrl Pts',(-0.117581146632055,7.56075370697551E-6,
-2.73508671147362));
#45901=CARTESIAN_POINT('Ctrl Pts',(-0.117581447556463,-9.82433484119326E-6,
-2.77521328852638));
#45902=CARTESIAN_POINT('Ctrl Pts',(-0.117595619370663,-0.0190922725530593,
-2.77392888697066));
#45903=CARTESIAN_POINT('Ctrl Pts',(-0.104183290718898,-0.077513766930232,
-2.76999538831228));
#45904=CARTESIAN_POINT('Ctrl Pts',(-0.0122251857505716,-0.138718630510878,
-2.76341279255126));
#45905=CARTESIAN_POINT('Ctrl Pts',(0.110010316820066,-0.0853817535458526,
-2.7554655012433));
#45906=CARTESIAN_POINT('Ctrl Pts',(0.131345999238215,0.0462659931371576,
-2.74751820993535));
#45907=CARTESIAN_POINT('Ctrl Pts',(0.0322130921955051,0.135479261605527,
-2.7395709186274));
#45908=CARTESIAN_POINT('Ctrl Pts',(-0.0881700120753839,0.102692212606021,
-2.73213594482441));
#45909=CARTESIAN_POINT('Ctrl Pts',(-0.117531720396742,0.031479001351202,
-2.72735006812407));
#45910=CARTESIAN_POINT('Ctrl Pts',(-0.117821958574713,-0.000103490888977657,
-2.72521328852638));
#45911=CARTESIAN_POINT('Origin',(0.,0.,-3.06008671147362));
#45912=CARTESIAN_POINT('',(-0.117925628517856,-6.40596713930419E-5,-2.83508671147362));
#45913=CARTESIAN_POINT('',(-0.117785807801612,0.00010769544346639,-2.82521328852638));
#45914=CARTESIAN_POINT('',(-0.117775,1.13296574333067E-13,-3.06008671147362));
#45915=CARTESIAN_POINT('Ctrl Pts',(-0.117925628517856,-6.40596713930531E-5,
-2.83508671147362));
#45916=CARTESIAN_POINT('Ctrl Pts',(-0.117949840251135,-0.00375807816172122,
-2.83483621198129));
#45917=CARTESIAN_POINT('Ctrl Pts',(-0.116115236168781,-0.0464929399061779,
-2.83193661538631));
#45918=CARTESIAN_POINT('Ctrl Pts',(-0.064018173970134,-0.123668891311378,
-2.82638792168868));
#45919=CARTESIAN_POINT('Ctrl Pts',(0.0693159272014078,-0.120779176949328,
-2.81844063038073));
#45920=CARTESIAN_POINT('Ctrl Pts',(0.139074531908459,-0.00711267889956292,
-2.81049333907277));
#45921=CARTESIAN_POINT('Ctrl Pts',(0.0812760328298283,0.113077501111085,
-2.80254604776482));
#45922=CARTESIAN_POINT('Ctrl Pts',(-0.0510676198065011,0.129554664787932,
-2.79459875645687));
#45923=CARTESIAN_POINT('Ctrl Pts',(-0.113682833675918,0.0546052015218531,
-2.78877897769313));
#45924=CARTESIAN_POINT('Ctrl Pts',(-0.117888853873725,0.00781411062496882,
-2.78560829603205));
#45925=CARTESIAN_POINT('Ctrl Pts',(-0.117817815448454,0.00010417526854233,
-2.78508671147362));
#45926=CARTESIAN_POINT('Ctrl Pts',(-0.117785807801612,0.000107695443466389,
-2.82521328852638));
#45927=CARTESIAN_POINT('Ctrl Pts',(-0.117504191843327,-0.0303119846466792,
-2.82315680291989));
#45928=CARTESIAN_POINT('Ctrl Pts',(-0.0899488852292908,-0.100369933896061,
-2.81845122021076));
#45929=CARTESIAN_POINT('Ctrl Pts',(0.0280979867448407,-0.136392139869556,
-2.81109654039897));
#45930=CARTESIAN_POINT('Ctrl Pts',(0.129885566115495,-0.0502200523954337,
-2.80314924909101));
#45931=CARTESIAN_POINT('Ctrl Pts',(0.112544041625198,0.082013123462066,
-2.79520195778306));
#45932=CARTESIAN_POINT('Ctrl Pts',(-0.00802119657383768,0.139025083726287,
-2.78725466647511));
#45933=CARTESIAN_POINT('Ctrl Pts',(-0.10293335038447,0.0799191353882865,
-2.78059177672288));
#45934=CARTESIAN_POINT('Ctrl Pts',(-0.117566389795404,0.0202655576060691,
-2.77657798407331));
#45935=CARTESIAN_POINT('Ctrl Pts',(-0.117581447556463,-9.82433484119326E-6,
-2.77521328852638));
#45936=CARTESIAN_POINT('Origin',(0.,0.,-3.06008671147362));
#45937=CARTESIAN_POINT('',(-0.117620976551725,-6.92605765801207E-5,-2.88508671147362));
#45938=CARTESIAN_POINT('',(-0.117945584131744,-4.75337169963674E-5,-2.87521328852638));
#45939=CARTESIAN_POINT('',(-0.117775,1.13296574333067E-13,-3.06008671147362));
#45940=CARTESIAN_POINT('Ctrl Pts',(-0.117620976551725,-6.92605765801272E-5,
-2.88508671147362));
#45941=CARTESIAN_POINT('Ctrl Pts',(-0.117701550786951,-0.0152483239620161,
-2.88406412793052));
#45942=CARTESIAN_POINT('Ctrl Pts',(-0.10791599027619,-0.0696504806793931,
-2.88039244728478));
#45943=CARTESIAN_POINT('Ctrl Pts',(-0.0258344786463291,-0.136840632652599,
-2.87407166953639));
#45944=CARTESIAN_POINT('Ctrl Pts',(0.101060618120367,-0.0958059291879449,
-2.86612437822844));
#45945=CARTESIAN_POINT('Ctrl Pts',(0.13526615819552,0.0330970741869585,
-2.85817708692048));
#45946=CARTESIAN_POINT('Ctrl Pts',(0.0454066843029653,0.131645762308753,
-2.85022979561253));
#45947=CARTESIAN_POINT('Ctrl Pts',(-0.081953579115799,0.11014957429056,
-2.84253300379691));
#45948=CARTESIAN_POINT('Ctrl Pts',(-0.117693794891987,0.035307125479465,
-2.83748530908394));
#45949=CARTESIAN_POINT('Ctrl Pts',(-0.117925628517856,-6.40596713930531E-5,
-2.83508671147362));
#45950=CARTESIAN_POINT('Ctrl Pts',(-0.117945584131744,-4.75337169963657E-5,
-2.87521328852638));
#45951=CARTESIAN_POINT('Ctrl Pts',(-0.117959142789025,-0.00269295294045094,
-2.87503381597178));
#45952=CARTESIAN_POINT('Ctrl Pts',(-0.116678262851619,-0.0443726330815549,
-2.87220524631453));
#45953=CARTESIAN_POINT('Ctrl Pts',(-0.0673061831817785,-0.121910832782649,
-2.86672757955463));
#45954=CARTESIAN_POINT('Ctrl Pts',(0.0660573824567498,-0.12259156477827,
-2.85878028824667));
#45955=CARTESIAN_POINT('Ctrl Pts',(0.138834266016569,-0.0108336871046625,
-2.85083299693873));
#45956=CARTESIAN_POINT('Ctrl Pts',(0.0842743478026822,0.110860972835297,
-2.84288570563077));
#45957=CARTESIAN_POINT('Ctrl Pts',(-0.0475806987781872,0.130875452878429,
-2.83493841432283));
#45958=CARTESIAN_POINT('Ctrl Pts',(-0.112968516313132,0.0567353707931715,
-2.82904760862136));
#45959=CARTESIAN_POINT('Ctrl Pts',(-0.117866960256001,0.00887364647862188,
-2.82580590002254));
#45960=CARTESIAN_POINT('Ctrl Pts',(-0.117785807801612,0.000107695443466389,
-2.82521328852638));
#45961=CARTESIAN_POINT('Origin',(0.,0.,-3.06008671147362));
#45962=CARTESIAN_POINT('',(-0.117558445841294,-3.12605290917906E-5,-2.93508671147362));
#45963=CARTESIAN_POINT('',(-0.117640397146581,-8.56657636452568E-5,-2.92521328852638));
#45964=CARTESIAN_POINT('',(-0.117775,1.13296574333067E-13,-3.06008671147362));
#45965=CARTESIAN_POINT('Ctrl Pts',(-0.117558445841294,-3.12605290917947E-5,
-2.93508671147362));
#45966=CARTESIAN_POINT('Ctrl Pts',(-0.117410007759293,-0.0266293090558454,
-2.93329204387976));
#45967=CARTESIAN_POINT('Ctrl Pts',(-0.095425295455791,-0.0925554651998461,
-2.92884827918326));
#45968=CARTESIAN_POINT('Ctrl Pts',(0.0145658909989512,-0.138586676302172,
-2.92175541738409));
#45969=CARTESIAN_POINT('Ctrl Pts',(0.12428129992797,-0.0627284744858215,
-2.91380812607615));
#45970=CARTESIAN_POINT('Ctrl Pts',(0.120090271076318,0.0704991524890691,
-2.9058608347682));
#45971=CARTESIAN_POINT('Ctrl Pts',(0.00571135947086689,0.139151690834859,
-2.89791354346024));
#45972=CARTESIAN_POINT('Ctrl Pts',(-0.0984950632345573,0.0877255235924107,
-2.89098883569539));
#45973=CARTESIAN_POINT('Ctrl Pts',(-0.117492815789671,0.0240744415048385,
-2.88671322503318));
#45974=CARTESIAN_POINT('Ctrl Pts',(-0.117620976551725,-6.92605765801272E-5,
-2.88508671147362));
#45975=CARTESIAN_POINT('Ctrl Pts',(-0.117640397146581,-8.56657636452533E-5,
-2.92521328852638));
#45976=CARTESIAN_POINT('Ctrl Pts',(-0.117731162646286,-0.0142003580566992,
-2.92426173192102));
#45977=CARTESIAN_POINT('Ctrl Pts',(-0.108844415761643,-0.0675005170391406,
-2.920661078213));
#45978=CARTESIAN_POINT('Ctrl Pts',(-0.0294856614640362,-0.136111750350814,
-2.91441132740234));
#45979=CARTESIAN_POINT('Ctrl Pts',(0.0984576432878249,-0.0984710734890703,
-2.90646403609439));
#45980=CARTESIAN_POINT('Ctrl Pts',(0.136104684613073,0.0294603972989506,
-2.89851674478643));
#45981=CARTESIAN_POINT('Ctrl Pts',(0.0489145289672211,0.130384614459911,
-2.89056945347848));
#45982=CARTESIAN_POINT('Ctrl Pts',(-0.0801550832889095,0.112136573427275,
-2.88280163472513));
#45983=CARTESIAN_POINT('Ctrl Pts',(-0.117759010797814,0.0363546463746542,
-2.87768291307443));
#45984=CARTESIAN_POINT('Ctrl Pts',(-0.117945584131744,-4.75337169963657E-5,
-2.87521328852638));
#45985=CARTESIAN_POINT('Origin',(3.28582941601228E-18,0.,-0.0136500000000002));
#45986=CARTESIAN_POINT('',(-0.00798678478681935,0.146131905375825,-0.0136500000000002));
#45987=CARTESIAN_POINT('Ctrl Pts',(0.106356886625425,-0.0510349087439493,
-0.0136500000000001));
#45988=CARTESIAN_POINT('Ctrl Pts',(0.10797749373506,-0.048506909295007,
-0.0136500000000001));
#45989=CARTESIAN_POINT('Ctrl Pts',(0.109491831180351,-0.0459180783966364,
-0.01365));
#45990=CARTESIAN_POINT('Ctrl Pts',(0.110894447333282,-0.0432730197048374,
-0.0136500000000002));
#45991=CARTESIAN_POINT('Ctrl Pts',(0.114260347727643,-0.036925592381097,
-0.0136500000000004));
#45992=CARTESIAN_POINT('Ctrl Pts',(0.116984348240791,-0.0302554581673266,
-0.0136499999999999));
#45993=CARTESIAN_POINT('Ctrl Pts',(0.119089796519242,-0.0233578112726241,
-0.0136499999999997));
#45994=CARTESIAN_POINT('Ctrl Pts',(0.120241782982297,-0.0195837951018374,
-0.0136499999999996));
#45995=CARTESIAN_POINT('Ctrl Pts',(0.121205726309446,-0.0157487895062339,
-0.0136500000000004));
#45996=CARTESIAN_POINT('Ctrl Pts',(0.121984207803306,-0.0118757879252627,
-0.0136500000000002));
#45997=CARTESIAN_POINT('Ctrl Pts',(0.123386384522449,-0.00489985761365873,
-0.0136499999999998));
#45998=CARTESIAN_POINT('Ctrl Pts',(0.124190160703931,0.00220615526225158,
-0.0136499999999999));
#45999=CARTESIAN_POINT('Ctrl Pts',(0.124410018311042,0.00935781521445493,
-0.0136499999999999));
#46000=CARTESIAN_POINT('Ctrl Pts',(0.124518362026204,0.012882084485723,
-0.0136499999999999));
#46001=CARTESIAN_POINT('Ctrl Pts',(0.124484221856685,0.0164097982231168,
-0.0136500000000001));
#46002=CARTESIAN_POINT('Ctrl Pts',(0.124310440415547,0.0199246610494899,
-0.0136500000000001));
#46003=CARTESIAN_POINT('Ctrl Pts',(0.123841403627022,0.0294112895489918,
-0.01365));
#46004=CARTESIAN_POINT('Ctrl Pts',(0.122359308962272,0.0388174407805119,
-0.0136499999999999));
#46005=CARTESIAN_POINT('Ctrl Pts',(0.119889589499077,0.0479553918623724,
-0.0136500000000002));
#46006=CARTESIAN_POINT('Ctrl Pts',(0.118986999919028,0.0512949693133307,
-0.0136500000000003));
#46007=CARTESIAN_POINT('Ctrl Pts',(0.117952005112996,0.0545988186576902,
-0.0136500000000003));
#46008=CARTESIAN_POINT('Ctrl Pts',(0.116784106418537,0.0578577665921829,
-0.0136500000000002));
#46009=CARTESIAN_POINT('Ctrl Pts',(0.115748002753435,0.0607489487771823,
-0.01365));
#46010=CARTESIAN_POINT('Ctrl Pts',(0.114608972805582,0.0635995076652492,
-0.0136500000000001));
#46011=CARTESIAN_POINT('Ctrl Pts',(0.113370868331345,0.0663963390231016,
-0.0136500000000001));
#46012=CARTESIAN_POINT('Ctrl Pts',(0.111623408852175,0.0703437841455626,
-0.01365));
#46013=CARTESIAN_POINT('Ctrl Pts',(0.109677163187892,0.074188513161514,
-0.0136500000000003));
#46014=CARTESIAN_POINT('Ctrl Pts',(0.107534292680181,0.0779135678957582,
-0.0136500000000004));
#46015=CARTESIAN_POINT('Ctrl Pts',(0.104293166260343,0.0835477736356994,
-0.0136500000000005));
#46016=CARTESIAN_POINT('Ctrl Pts',(0.100602795829931,0.0889085421797832,
-0.0136500000000002));
#46017=CARTESIAN_POINT('Ctrl Pts',(0.0965158424099242,0.0939776949692943,
-0.0136500000000003));
#46018=CARTESIAN_POINT('Ctrl Pts',(0.0944562159089865,0.0965323023625348,
-0.0136500000000003));
#46019=CARTESIAN_POINT('Ctrl Pts',(0.0922956872886706,0.0990127808204909,
-0.0136500000000004));
#46020=CARTESIAN_POINT('Ctrl Pts',(0.090040009153852,0.101416277916268,
-0.0136500000000003));
#46021=CARTESIAN_POINT('Ctrl Pts',(0.087748564367495,0.103857885521595,
-0.0136500000000002));
#46022=CARTESIAN_POINT('Ctrl Pts',(0.0853639556028889,0.10621444018175,
-0.0136500000000006));
#46023=CARTESIAN_POINT('Ctrl Pts',(0.0828986900609891,0.108478986224309,
-0.0136500000000005));
#46024=CARTESIAN_POINT('Ctrl Pts',(0.0767583099038693,0.114119422659364,
-0.0136500000000003));
#46025=CARTESIAN_POINT('Ctrl Pts',(0.0701100271741426,0.119199823308631,
-0.0136500000000007));
#46026=CARTESIAN_POINT('Ctrl Pts',(0.0630566235181073,0.123682391417081,
-0.0136500000000005));
#46027=CARTESIAN_POINT('Ctrl Pts',(0.0583782755736549,0.126655567817966,
-0.0136500000000003));
#46028=CARTESIAN_POINT('Ctrl Pts',(0.0535211481662564,0.129365518098269,
-0.0136500000000002));
#46029=CARTESIAN_POINT('Ctrl Pts',(0.0485105898935787,0.131797135777499,
-0.0136500000000002));
#46030=CARTESIAN_POINT('Ctrl Pts',(0.0456575463118391,0.133181714268642,
-0.0136500000000002));
#46031=CARTESIAN_POINT('Ctrl Pts',(0.0427550251642698,0.134475492007146,
-0.0136500000000003));
#46032=CARTESIAN_POINT('Ctrl Pts',(0.0398205425663953,0.135670768783895,
-0.0136500000000003));
#46033=CARTESIAN_POINT('Ctrl Pts',(0.0302520139346001,0.139568232708038,
-0.0136500000000002));
#46034=CARTESIAN_POINT('Ctrl Pts',(0.0203132057297043,0.142438162792591,
-0.0136500000000004));
#46035=CARTESIAN_POINT('Ctrl Pts',(0.0101716141419635,0.144199039300689,
-0.0136500000000002));
#46036=CARTESIAN_POINT('Ctrl Pts',(0.00417993901636529,0.145239369103121,
-0.01365));
#46037=CARTESIAN_POINT('Ctrl Pts',(-0.00188321839195679,0.14589189591373,
-0.0136500000000001));
#46038=CARTESIAN_POINT('Ctrl Pts',(-0.00798678478681931,0.146131905375825,
-0.0136500000000002));
#46039=CARTESIAN_POINT('',(-0.14635,-1.79227059055215E-17,-0.0136500000000001));
#46040=CARTESIAN_POINT('Origin',(0.,0.,-0.0136500000000002));
#46041=CARTESIAN_POINT('',(-0.119330942213657,0.085138415363241,-0.013650000000002));
#46042=CARTESIAN_POINT('Origin',(0.,0.,-0.0136500000000002));
#46043=CARTESIAN_POINT('Ctrl Pts',(-0.119330942213682,0.0851384153632074,
-0.0136499999999997));
#46044=CARTESIAN_POINT('Ctrl Pts',(-0.121198726066873,0.0819569309101861,
-0.0136499999999997));
#46045=CARTESIAN_POINT('Ctrl Pts',(-0.122934816712479,0.0787053437274808,
-0.0136499999999999));
#46046=CARTESIAN_POINT('Ctrl Pts',(-0.124531604043384,0.0753872965898214,
-0.0136499999999998));
#46047=CARTESIAN_POINT('Ctrl Pts',(-0.127644196141878,0.0689194801791971,
-0.0136499999999995));
#46048=CARTESIAN_POINT('Ctrl Pts',(-0.130228216974403,0.0621991413433847,
-0.0136499999999996));
#46049=CARTESIAN_POINT('Ctrl Pts',(-0.132285959409066,0.0552930525211129,
-0.0136499999999993));
#46050=CARTESIAN_POINT('Ctrl Pts',(-0.133637403415453,0.0507574059847852,
-0.0136499999999992));
#46051=CARTESIAN_POINT('Ctrl Pts',(-0.134761526400422,0.0461391411278747,
-0.0136499999999996));
#46052=CARTESIAN_POINT('Ctrl Pts',(-0.135653414685908,0.0414802748139204,
-0.0136499999999996));
#46053=CARTESIAN_POINT('Ctrl Pts',(-0.13686902110764,0.0351304349276935,
-0.0136499999999997));
#46054=CARTESIAN_POINT('Ctrl Pts',(-0.137656705017299,0.0286962406659602,
-0.0136499999999995));
#46055=CARTESIAN_POINT('Ctrl Pts',(-0.13801608155741,0.0222270992451787,
-0.0136499999999991));
#46056=CARTESIAN_POINT('Ctrl Pts',(-0.138199023739623,0.0189339548228916,
-0.0136499999999989));
#46057=CARTESIAN_POINT('Ctrl Pts',(-0.138270844463559,0.0156317713083359,
-0.0136499999999985));
#46058=CARTESIAN_POINT('Ctrl Pts',(-0.138230698014712,0.0123273216632419,
-0.0136499999999984));
#46059=CARTESIAN_POINT('Ctrl Pts',(-0.138188662178769,0.00886735678074606,
-0.0136499999999982));
#46060=CARTESIAN_POINT('Ctrl Pts',(-0.138023945600157,0.00541434562535705,
-0.0136499999999993));
#46061=CARTESIAN_POINT('Ctrl Pts',(-0.137737265449259,0.0019780480046521,
-0.0136499999999993));
#46062=CARTESIAN_POINT('Ctrl Pts',(-0.136918974928002,-0.0078304084316795,
-0.0136499999999994));
#46063=CARTESIAN_POINT('Ctrl Pts',(-0.135110265356286,-0.0175107005685719,
-0.0136499999999995));
#46064=CARTESIAN_POINT('Ctrl Pts',(-0.132295379661141,-0.0268797270541801,
-0.0136499999999994));
#46065=CARTESIAN_POINT('Ctrl Pts',(-0.131155623417163,-0.0306732759202626,
-0.0136499999999994));
#46066=CARTESIAN_POINT('Ctrl Pts',(-0.129850387617751,-0.0344155153559583,
-0.0136500000000002));
#46067=CARTESIAN_POINT('Ctrl Pts',(-0.128376581127422,-0.0380927221985045,
-0.0136500000000004));
#46068=CARTESIAN_POINT('Ctrl Pts',(-0.127294239500948,-0.0407932083620289,
-0.0136500000000005));
#46069=CARTESIAN_POINT('Ctrl Pts',(-0.126122089187759,-0.0434552743016918,
-0.0136500000000001));
#46070=CARTESIAN_POINT('Ctrl Pts',(-0.124863185252744,-0.0460663274824253,
-0.01365));
#46071=CARTESIAN_POINT('Ctrl Pts',(-0.122907807025548,-0.0501219161557532,
-0.0136499999999999));
#46072=CARTESIAN_POINT('Ctrl Pts',(-0.120741025491108,-0.0540601902277737,
-0.0136499999999991));
#46073=CARTESIAN_POINT('Ctrl Pts',(-0.118360761739933,-0.0578624096065901,
-0.0136499999999992));
#46074=CARTESIAN_POINT('Ctrl Pts',(-0.114440131085056,-0.0641252020579709,
-0.0136499999999994));
#46075=CARTESIAN_POINT('Ctrl Pts',(-0.109940665047455,-0.0700197682606754,
-0.0136499999999996));
#46076=CARTESIAN_POINT('Ctrl Pts',(-0.10493387405501,-0.075499387422339,
-0.0136499999999995));
#46077=CARTESIAN_POINT('Ctrl Pts',(-0.102913339621813,-0.077710735811688,
-0.0136499999999994));
#46078=CARTESIAN_POINT('Ctrl Pts',(-0.100808353999335,-0.0798559352178832,
-0.0136499999999995));
#46079=CARTESIAN_POINT('Ctrl Pts',(-0.0986289428089273,-0.0819258236072475,
-0.0136499999999996));
#46080=CARTESIAN_POINT('Ctrl Pts',(-0.0918665361750953,-0.088348396381554,
-0.01365));
#46081=CARTESIAN_POINT('Ctrl Pts',(-0.0844256807446546,-0.0940174328437391,
-0.0136499999999999));
#46082=CARTESIAN_POINT('Ctrl Pts',(-0.0764567779821786,-0.0988447114068085,
-0.01365));
#46083=CARTESIAN_POINT('Ctrl Pts',(-0.071808772676882,-0.101660308113164,
-0.01365));
#46084=CARTESIAN_POINT('Ctrl Pts',(-0.0669805865634173,-0.104188713709908,
-0.0136499999999998));
#46085=CARTESIAN_POINT('Ctrl Pts',(-0.0620003236069234,-0.106404393078832,
-0.0136499999999997));
#46086=CARTESIAN_POINT('Ctrl Pts',(-0.0592527274166011,-0.107626776765439,
-0.0136499999999996));
#46087=CARTESIAN_POINT('Ctrl Pts',(-0.0564585789255776,-0.108753606517434,
-0.0136499999999994));
#46088=CARTESIAN_POINT('Ctrl Pts',(-0.0536364829015093,-0.109775780828203,
-0.0136499999999995));
#46089=CARTESIAN_POINT('Ctrl Pts',(-0.0454122711661217,-0.112754622756523,
-0.0136499999999999));
#46090=CARTESIAN_POINT('Ctrl Pts',(-0.0369224943427728,-0.114861623947457,
-0.0136500000000008));
#46091=CARTESIAN_POINT('Ctrl Pts',(-0.0282900439033421,-0.115996210102783,
-0.0136500000000007));
#46092=CARTESIAN_POINT('Ctrl Pts',(-0.023506892932931,-0.116624872486418,
-0.0136500000000006));
#46093=CARTESIAN_POINT('Ctrl Pts',(-0.0186799033642427,-0.116954139727108,
-0.0136500000000002));
#46094=CARTESIAN_POINT('Ctrl Pts',(-0.0138313775859597,-0.116960008631475,
-0.0136500000000002));
#46095=CARTESIAN_POINT('Ctrl Pts',(0.103670563470606,-0.0558870726974231,
-2.95414778394209));
#46096=CARTESIAN_POINT('Ctrl Pts',(0.122275110647363,-0.0213756231646796,
-2.95149868683944));
#46097=CARTESIAN_POINT('Ctrl Pts',(0.121984618190939,0.0670884644041237,
-2.94620049263415));
#46098=CARTESIAN_POINT('Ctrl Pts',(0.00941180899824742,0.139031834987488,
-2.93825320132619));
#46099=CARTESIAN_POINT('Ctrl Pts',(-0.111685438487879,0.0831087463150725,
-2.93030591001824));
#46100=CARTESIAN_POINT('Ctrl Pts',(-0.13039962705173,-0.0488645184779689,
-2.92235861871029));
#46101=CARTESIAN_POINT('Ctrl Pts',(-0.0294856614640362,-0.136111750350814,
-2.91441132740234));
#46102=CARTESIAN_POINT('Ctrl Pts',(0.0984576432878249,-0.0984710734890703,
-2.90646403609439));
#46103=CARTESIAN_POINT('Ctrl Pts',(0.136104684613073,0.0294603972989506,
-2.89851674478643));
#46104=CARTESIAN_POINT('Ctrl Pts',(0.0489145289672211,0.130384614459911,
-2.89056945347848));
#46105=CARTESIAN_POINT('Ctrl Pts',(-0.0831371885321713,0.111714959246436,
-2.88262216217053));
#46106=CARTESIAN_POINT('Ctrl Pts',(-0.138937831621556,-0.0094142740234505,
-2.87467487086258));
#46107=CARTESIAN_POINT('Ctrl Pts',(-0.0673061831817785,-0.121910832782649,
-2.86672757955463));
#46108=CARTESIAN_POINT('Ctrl Pts',(0.0660573824567498,-0.12259156477827,
-2.85878028824667));
#46109=CARTESIAN_POINT('Ctrl Pts',(0.138834266016569,-0.0108336871046625,
-2.85083299693873));
#46110=CARTESIAN_POINT('Ctrl Pts',(0.0842743478026822,0.110860972835297,
-2.84288570563077));
#46111=CARTESIAN_POINT('Ctrl Pts',(-0.0475806987781872,0.130875452878429,
-2.83493841432283));
#46112=CARTESIAN_POINT('Ctrl Pts',(-0.135795462645268,0.030853000978399,
-2.82699112301486));
#46113=CARTESIAN_POINT('Ctrl Pts',(-0.0994606430770848,-0.0974674046326144,
-2.81904383170692));
#46114=CARTESIAN_POINT('Ctrl Pts',(0.0280979867448407,-0.136392139869556,
-2.81109654039897));
#46115=CARTESIAN_POINT('Ctrl Pts',(0.129885566115495,-0.0502200523954337,
-2.80314924909101));
#46116=CARTESIAN_POINT('Ctrl Pts',(0.112544041625198,0.082013123462066,
-2.79520195778306));
#46117=CARTESIAN_POINT('Ctrl Pts',(-0.00802119657383768,0.139025083726287,
-2.78725466647511));
#46118=CARTESIAN_POINT('Ctrl Pts',(-0.121229513542639,0.0685253145656341,
-2.77930737516716));
#46119=CARTESIAN_POINT('Ctrl Pts',(-0.123247930400552,-0.0648248509142736,
-2.77136008385921));
#46120=CARTESIAN_POINT('Ctrl Pts',(-0.0122251857505716,-0.138718630510878,
-2.76341279255126));
#46121=CARTESIAN_POINT('Ctrl Pts',(0.110010316820066,-0.0853817535458526,
-2.7554655012433));
#46122=CARTESIAN_POINT('Ctrl Pts',(0.131345999238215,0.0462659931371576,
-2.74751820993535));
#46123=CARTESIAN_POINT('Ctrl Pts',(0.0322130921955051,0.135479261605527,
-2.7395709186274));
#46124=CARTESIAN_POINT('Ctrl Pts',(-0.0964651820724651,0.100432974095761,
-2.73162362731945));
#46125=CARTESIAN_POINT('Ctrl Pts',(-0.136667031580617,-0.0267289377911359,
-2.7236763360115));
#46126=CARTESIAN_POINT('Ctrl Pts',(-0.0515199201897912,-0.12937546699384,
-2.71572904470355));
#46127=CARTESIAN_POINT('Ctrl Pts',(0.0808804927988873,-0.113360749474457,
-2.7077817533956));
#46128=CARTESIAN_POINT('Ctrl Pts',(0.139098525352115,0.0066267549690055,
-2.69983446208764));
#46129=CARTESIAN_POINT('Ctrl Pts',(0.0697374672192116,0.120536298692083,
-2.69188717077969));
#46130=CARTESIAN_POINT('Ctrl Pts',(-0.0635857546542645,0.123891748884511,
-2.68393987947174));
#46131=CARTESIAN_POINT('Ctrl Pts',(-0.138589071705656,0.0136155367260933,
-2.67599258816378));
#46132=CARTESIAN_POINT('Ctrl Pts',(-0.0864805613488348,-0.109148642434832,
-2.66804529685584));
#46133=CARTESIAN_POINT('Ctrl Pts',(0.0449466287065965,-0.131803316363808,
-2.66009800554788));
#46134=CARTESIAN_POINT('Ctrl Pts',(0.135149441973695,-0.0335699563714237,
-2.65215071423994));
#46135=CARTESIAN_POINT('Ctrl Pts',(0.10139520486838,0.0954532663992196,
-2.64420342293198));
#46136=CARTESIAN_POINT('Ctrl Pts',(-0.0253572002932921,0.136928178363215,
-2.63625613162403));
#46137=CARTESIAN_POINT('Ctrl Pts',(-0.128852359933585,0.05281460949517,
-2.62830884031608));
#46138=CARTESIAN_POINT('Ctrl Pts',(-0.114166058832061,-0.0797397306700743,
-2.62036154900813));
#46139=CARTESIAN_POINT('Ctrl Pts',(0.00523164691012173,-0.139157980393471,
-2.61241425770018));
#46140=CARTESIAN_POINT('Ctrl Pts',(0.119830964215785,-0.0709426081540357,
-2.60446696639222));
#46141=CARTESIAN_POINT('Ctrl Pts',(0.12452311024091,0.0623402650981849,
-2.59651967508427));
#46142=CARTESIAN_POINT('Ctrl Pts',(0.0150045187058493,0.138445577953893,
-2.58857238377632));
#46143=CARTESIAN_POINT('Ctrl Pts',(-0.108275993366011,0.0875706737280534,
-2.58062509246837));
#46144=CARTESIAN_POINT('Ctrl Pts',(-0.132247380902922,-0.0436227449950054,
-2.57267780116042));
#46145=CARTESIAN_POINT('Ctrl Pts',(-0.0349234451532213,-0.134806033304195,
-2.56473050985246));
#46146=CARTESIAN_POINT('Ctrl Pts',(0.0944317530776,-0.102347240545473,-2.55678321854452));
#46147=CARTESIAN_POINT('Ctrl Pts',(0.137175557268965,0.0239829131785638,
-2.54883592723656));
#46148=CARTESIAN_POINT('Ctrl Pts',(0.0541039883893578,0.128316297004496,
-2.54088863592861));
#46149=CARTESIAN_POINT('Ctrl Pts',(-0.0785909508585415,0.114959889003652,
-2.53294134462066));
#46150=CARTESIAN_POINT('Ctrl Pts',(-0.139203443356235,-0.00383601281920323,
-2.52499405331271));
#46151=CARTESIAN_POINT('Ctrl Pts',(-0.0721406159404224,-0.119113580956658,
-2.51704676200475));
#46152=CARTESIAN_POINT('Ctrl Pts',(0.0610885073433754,-0.125141951028183,
-2.50909947069681));
#46153=CARTESIAN_POINT('Ctrl Pts',(0.1382881637544,-0.0163919920088414,
-2.50115217938885));
#46154=CARTESIAN_POINT('Ctrl Pts',(0.0886519810374287,0.107392457345575,
-2.4932048880809));
#46155=CARTESIAN_POINT('Ctrl Pts',(-0.0422944750968055,0.132678148211631,
-2.48525759677295));
#46156=CARTESIAN_POINT('Ctrl Pts',(-0.134449070136487,0.0362734224469619,
-2.477310305465));
#46157=CARTESIAN_POINT('Ctrl Pts',(-0.103288985396153,-0.0934007448172382,
-2.46936301415705));
#46158=CARTESIAN_POINT('Ctrl Pts',(0.0226062146261162,-0.137409143425246,
-2.46141572284909));
#46159=CARTESIAN_POINT('Ctrl Pts',(0.127767332108225,-0.0553879272272235,
-2.45346843154115));
#46160=CARTESIAN_POINT('Ctrl Pts',(0.115742160170272,0.0774342688717387,
-2.44552114023319));
#46161=CARTESIAN_POINT('Ctrl Pts',(-0.00243999302426519,0.139234909669319,
-2.43757384892524));
#46162=CARTESIAN_POINT('Ctrl Pts',(-0.118384221046488,0.0733313701208286,
-2.42962655761729));
#46163=CARTESIAN_POINT('Ctrl Pts',(-0.125748209022913,-0.0598306072517374,
-2.42167926630934));
#46164=CARTESIAN_POINT('Ctrl Pts',(-0.0177778171272468,-0.138116844934903,
-2.41373197500138));
#46165=CARTESIAN_POINT('Ctrl Pts',(0.106498123211473,-0.0897243745534934,
-2.40578468369343));
#46166=CARTESIAN_POINT('Ctrl Pts',(0.133095574977059,0.0409619525670818,
-2.39783739238548));
#46167=CARTESIAN_POINT('Ctrl Pts',(0.0376197525149271,0.134078588362562,
-2.38989010107753));
#46168=CARTESIAN_POINT('Ctrl Pts',(-0.09236034528412,0.104220344729711,
-2.38194280976958));
#46169=CARTESIAN_POINT('Ctrl Pts',(-0.137628913345395,-0.0212272430604503,
-2.37399551846163));
#46170=CARTESIAN_POINT('Ctrl Pts',(-0.0566662969110845,-0.127205520442183,
-2.36604822715368));
#46171=CARTESIAN_POINT('Ctrl Pts',(0.0762698010119113,-0.116512793675996,
-2.35810093584572));
#46172=CARTESIAN_POINT('Ctrl Pts',(0.13925237616884,0.00104372789252618,
-2.35015364453777));
#46173=CARTESIAN_POINT('Ctrl Pts',(0.0745147509671164,0.117642957821071,
-2.34220635322982));
#46174=CARTESIAN_POINT('Ctrl Pts',(-0.0585666913028059,0.126341823266975,
-2.33425906192187));
#46175=CARTESIAN_POINT('Ctrl Pts',(-0.137931638721192,0.0191618547189039,
-2.32631177061392));
#46176=CARTESIAN_POINT('Ctrl Pts',(-0.0907877464490561,-0.105593080887356,
-2.31836447930597));
#46177=CARTESIAN_POINT('Ctrl Pts',(0.0396253113885193,-0.133499619227714,
-2.31041718799801));
#46178=CARTESIAN_POINT('Ctrl Pts',(0.13369462523368,-0.0389622999861087,
-2.30246989669006));
#46179=CARTESIAN_POINT('Ctrl Pts',(0.105141224899681,0.0913106590885011,
-2.29452260538211));
#46180=CARTESIAN_POINT('Ctrl Pts',(-0.0198461371346163,0.137834844931954,
-2.28657531407416));
#46181=CARTESIAN_POINT('Ctrl Pts',(-0.126630918495495,0.0579389689032257,
-2.27862802276621));
#46182=CARTESIAN_POINT('Ctrl Pts',(-0.117271712035045,-0.0750976643641544,
-2.27068073145826));
#46183=CARTESIAN_POINT('Ctrl Pts',(-0.00035264218412894,-0.139255841098576,
-2.2627334401503));
#46184=CARTESIAN_POINT('Ctrl Pts',(0.116889865813058,-0.0756906394925223,
-2.25478614884235));
#46185=CARTESIAN_POINT('Ctrl Pts',(0.126922734073552,0.0572968865810018,
-2.2468388575344));
#46186=CARTESIAN_POINT('Ctrl Pts',(0.020543965621383,0.137732563735411,
-2.23889156622645));
#46187=CARTESIAN_POINT('Ctrl Pts',(-0.10467742137356,0.0918419898040323,
-2.2309442749185));
#46188=CARTESIAN_POINT('Ctrl Pts',(-0.133890240337692,-0.0382846859579246,
-2.22299698361055));
#46189=CARTESIAN_POINT('Ctrl Pts',(-0.0403009298698327,-0.133297219356626,
-2.2150496923026));
#46190=CARTESIAN_POINT('Ctrl Pts',(0.0902517917743938,-0.106051533313259,
-2.20710240099464));
#46191=CARTESIAN_POINT('Ctrl Pts',(0.13802691747888,0.0184630357162695,
-2.19915510968669));
#46192=CARTESIAN_POINT('Ctrl Pts',(0.059205815238823,0.12604358404333,-2.19120781837874));
#46193=CARTESIAN_POINT('Ctrl Pts',(-0.0739179767846482,0.118018838939578,
-2.18326052707079));
#46194=CARTESIAN_POINT('Ctrl Pts',(-0.139245304110133,0.00174897680326264,
-2.17531323576284));
#46195=CARTESIAN_POINT('Ctrl Pts',(-0.0768589174636237,-0.116125020744462,
-2.16736594445488));
#46196=CARTESIAN_POINT('Ctrl Pts',(0.0560213207628474,-0.127490883033133,
-2.15941865314694));
#46197=CARTESIAN_POINT('Ctrl Pts',(0.137519639994184,-0.0219240108659811,
-2.15147136183898));
#46198=CARTESIAN_POINT('Ctrl Pts',(0.0928869986161953,0.103751236737962,
-2.14352407053103));
#46199=CARTESIAN_POINT('Ctrl Pts',(-0.0369402110727147,0.134267399030759,
-2.13557677922308));
#46200=CARTESIAN_POINT('Ctrl Pts',(-0.132886410689829,0.0416355075693321,
-2.12762948791513));
#46201=CARTESIAN_POINT('Ctrl Pts',(-0.106951178440612,-0.0891838498089545,
-2.11968219660718));
#46202=CARTESIAN_POINT('Ctrl Pts',(0.0170780778737081,-0.138205111673633,
-2.11173490529922));
#46203=CARTESIAN_POINT('Ctrl Pts',(0.125443576141085,-0.0604667085388119,
-2.10378761399128));
#46204=CARTESIAN_POINT('Ctrl Pts',(0.118754099267359,0.0727308568888059,
-2.09584032268332));
#46205=CARTESIAN_POINT('Ctrl Pts',(0.00314513556600165,0.139220766262987,
-2.08789303137537));
#46206=CARTESIAN_POINT('Ctrl Pts',(-0.115348499519044,0.0780194674122224,
-2.07994574006742));
#46207=CARTESIAN_POINT('Ctrl Pts',(-0.128046213019386,-0.0547401221041357,
-2.07199844875947));
#46208=CARTESIAN_POINT('Ctrl Pts',(-0.0233018516916921,-0.1372928889066,
-2.06405115745151));
#46209=CARTESIAN_POINT('Ctrl Pts',(0.102814620106721,-0.0939226678118359,
-2.05610386614357));
#46210=CARTESIAN_POINT('Ctrl Pts',(0.134631057384304,0.035592021917362,
-2.04815657483561));
#46211=CARTESIAN_POINT('Ctrl Pts',(0.0429658988952774,0.132462240539342,
-2.04020928352766));
#46212=CARTESIAN_POINT('Ctrl Pts',(-0.0881069405717808,0.10784006982408,
-2.03226199221971));
#46213=CARTESIAN_POINT('Ctrl Pts',(-0.138369409599115,-0.0156914028618916,
-2.02431470091176));
#46214=CARTESIAN_POINT('Ctrl Pts',(-0.0617215220226959,-0.124830955118446,
-2.0163674096038));
#46215=CARTESIAN_POINT('Ctrl Pts',(0.0715364240393441,-0.11947741908932,
-2.00842011829585));
#46216=CARTESIAN_POINT('Ctrl Pts',(0.139182230024373,-0.00454097809115471,
-2.0004728269879));
#46217=CARTESIAN_POINT('Ctrl Pts',(0.0791721726471583,0.114560380214585,
-1.99252553567995));
#46218=CARTESIAN_POINT('Ctrl Pts',(-0.0534534194270322,0.128588668194905,
-1.984578244372));
#46219=CARTESIAN_POINT('Ctrl Pts',(-0.137052333272063,0.02467734955916,
-1.97663095306404));
#46220=CARTESIAN_POINT('Ctrl Pts',(-0.0949488932563241,-0.101867665654913,
-1.9686836617561));
#46221=CARTESIAN_POINT('Ctrl Pts',(0.0342402540498007,-0.13498117883315,
-1.96073637044814));
#46222=CARTESIAN_POINT('Ctrl Pts',(0.132024751554693,-0.0442919700792729,
-1.95278907914019));
#46223=CARTESIAN_POINT('Ctrl Pts',(0.108718118087273,0.0870211723441102,
-1.94484178783224));
#46224=CARTESIAN_POINT('Ctrl Pts',(-0.0143031501084346,0.138519794735472,
-1.93689449652429));
#46225=CARTESIAN_POINT('Ctrl Pts',(-0.12420578257333,0.0629701295212927,
-1.92894720521634));
#46226=CARTESIAN_POINT('Ctrl Pts',(-0.120188725676985,-0.0703347983342829,
-1.92099991390838));
#46227=CARTESIAN_POINT('Ctrl Pts',(-0.00593636402933215,-0.139129699269039,
-1.91305262260043));
#46228=CARTESIAN_POINT('Ctrl Pts',(0.113760742075024,-0.0803169172660493,
-1.90510533129248));
#46229=CARTESIAN_POINT('Ctrl Pts',(0.129118194016824,0.052161342107116,
-1.89715803998453));
#46230=CARTESIAN_POINT('Ctrl Pts',(0.0260503661646103,0.136797997277999,
-1.88921074867658));
#46231=CARTESIAN_POINT('Ctrl Pts',(-0.10091046859706,0.0959655717645845,
-1.88126345736863));
#46232=CARTESIAN_POINT('Ctrl Pts',(-0.135317728173232,-0.0328850433877962,
-1.87331616606068));
#46233=CARTESIAN_POINT('Ctrl Pts',(-0.0456135877873082,-0.131573987724592,
-1.86536887475272));
#46234=CARTESIAN_POINT('Ctrl Pts',(0.085926654297937,-0.109585234944059,
-1.85742158344477));
#46235=CARTESIAN_POINT('Ctrl Pts',(0.138656251961757,0.0129134591995952,
-1.84947429213682));
#46236=CARTESIAN_POINT('Ctrl Pts',(0.0642124054894162,0.123568121365685,
-1.84152700082887));
#46237=CARTESIAN_POINT('Ctrl Pts',(-0.0691261005948764,0.120887947509786,
-1.83357970952092));
#46238=CARTESIAN_POINT('Ctrl Pts',(-0.139063179278854,0.00733115307704587,
-1.82563241821296));
#46239=CARTESIAN_POINT('Ctrl Pts',(-0.0814535861669311,-0.112949665502506,
-1.81768512690502));
#46240=CARTESIAN_POINT('Ctrl Pts',(0.0508640200603842,-0.129634737242294,
-1.80973783559706));
#46241=CARTESIAN_POINT('Ctrl Pts',(0.136529906497424,-0.0274207634537505,
-1.80179054428911));
#46242=CARTESIAN_POINT('Ctrl Pts',(0.0969726011114629,0.0999431251775667,
-1.79384325298116));
#46243=CARTESIAN_POINT('Ctrl Pts',(-0.0315265261952861,0.13564067156513,
-1.78589596167321));
#46244=CARTESIAN_POINT('Ctrl Pts',(-0.131109994372513,0.0469306191331561,
-1.77794867036525));
#46245=CARTESIAN_POINT('Ctrl Pts',(-0.110441333207432,-0.0848234964850357,
-1.77000137905731));
#46246=CARTESIAN_POINT('Ctrl Pts',(0.0115224698662327,-0.138778767557446,
-1.76205408774935));
#46247=CARTESIAN_POINT('Ctrl Pts',(0.122918035611167,-0.0654482250185099,
-1.7541067964414));
#46248=CARTESIAN_POINT('Ctrl Pts',(0.121575014282259,0.06791045235345,-1.74615950513345));
#46249=CARTESIAN_POINT('Ctrl Pts',(0.00872520499083007,0.138982676742282,
-1.7382122138255));
#46250=CARTESIAN_POINT('Ctrl Pts',(-0.112127232049285,0.0825820650598395,
-1.73026492251755));
#46251=CARTESIAN_POINT('Ctrl Pts',(-0.130138245933848,-0.0495615837301763,
-1.7223176312096));
#46252=CARTESIAN_POINT('Ctrl Pts',(-0.0287884036356622,-0.136248087886369,
-1.71437033990164));
#46253=CARTESIAN_POINT('Ctrl Pts',(0.0989657326610272,-0.0979698800420198,
-1.70642304859369));
#46254=CARTESIAN_POINT('Ctrl Pts',(0.135949976537486,0.0301648390686699,
-1.69847575728574));
#46255=CARTESIAN_POINT('Ctrl Pts',(0.0482429316917392,0.130632818152132,
-1.69052846597779));
#46256=CARTESIAN_POINT('Ctrl Pts',(-0.0837118098258903,0.111286326798289,
-1.68258117466984));
#46257=CARTESIAN_POINT('Ctrl Pts',(-0.138887329203821,-0.0101303219697604,
-1.67463388336189));
#46258=CARTESIAN_POINT('Ctrl Pts',(-0.0666774638491984,-0.122255590674703,
-1.66668659205393));
#46259=CARTESIAN_POINT('Ctrl Pts',(0.0666879758411977,-0.122249856911105,
-1.65873930074598));
#46260=CARTESIAN_POINT('Ctrl Pts',(0.138888199753706,-0.0101183796013297,
-1.65079200943803));
#46261=CARTESIAN_POINT('Ctrl Pts',(0.0837022404783003,0.111293524409529,
-1.64284471813008));
#46262=CARTESIAN_POINT('Ctrl Pts',(-0.0482541640740641,0.130628669464612,
-1.63489742682213));
#46263=CARTESIAN_POINT('Ctrl Pts',(-0.135952569781179,0.030153149196646,
-1.62695013551418));
#46264=CARTESIAN_POINT('Ctrl Pts',(-0.0989573082816934,-0.097978389322461,
-1.61900284420623));
#46265=CARTESIAN_POINT('Ctrl Pts',(0.0288001189230785,-0.136245611990252,
-1.61105555289827));
#46266=CARTESIAN_POINT('Ctrl Pts',(0.130142507042637,-0.0495503935124521,
-1.60310826159032));
#46267=CARTESIAN_POINT('Ctrl Pts',(0.112120130754087,0.0825917060985434,
-1.59516097028237));
#46268=CARTESIAN_POINT('Ctrl Pts',(-0.00873715548808248,0.138981925985211,
-1.58721367897442));
#46269=CARTESIAN_POINT('Ctrl Pts',(-0.121580853163911,0.0678999983837808,
-1.57926638766647));
#46270=CARTESIAN_POINT('Ctrl Pts',(-0.122912407542141,-0.0654587939758788,
-1.57131909635852));
#46271=CARTESIAN_POINT('Ctrl Pts',(-0.0115105368274101,-0.138779757812609,
-1.56337180505056));
#46272=CARTESIAN_POINT('Ctrl Pts',(0.110448626411003,-0.0848139997907445,
-1.55542451374261));
#46273=CARTESIAN_POINT('Ctrl Pts',(0.131105958523409,0.0469418925506857,
-1.54747722243466));
#46274=CARTESIAN_POINT('Ctrl Pts',(0.0315148629140466,0.135643381895656,
-1.53952993112671));
#46275=CARTESIAN_POINT('Ctrl Pts',(-0.0969811944374197,0.0999347865463928,
-1.53158263981876));
#46276=CARTESIAN_POINT('Ctrl Pts',(-0.136527548197828,-0.0274325029786067,
-1.5236353485108));
#46277=CARTESIAN_POINT('Ctrl Pts',(-0.0508528731324187,-0.129639110343907,
-1.51568805720286));
#46278=CARTESIAN_POINT('Ctrl Pts',(0.0814632979273637,-0.112942661237371,
-1.5077407658949));
#46279=CARTESIAN_POINT('Ctrl Pts',(0.139062548390083,0.0073431105015257,
-1.49979347458695));
#46280=CARTESIAN_POINT('Ctrl Pts',(0.0691157056986611,0.120893890922402,
-1.491846183279));
#46281=CARTESIAN_POINT('Ctrl Pts',(-0.0642230303494631,0.123562599557122,
-1.48389889197105));
#46282=CARTESIAN_POINT('Ctrl Pts',(-0.138657361822632,0.0129015366902274,
-1.4759516006631));
#46283=CARTESIAN_POINT('Ctrl Pts',(-0.0859172312118186,-0.109592623006646,
-1.46800430935514));
#46284=CARTESIAN_POINT('Ctrl Pts',(0.045624901106524,-0.131570065119699,
-1.46005701804719));
#46285=CARTESIAN_POINT('Ctrl Pts',(0.135320555318067,-0.0328734078700636,
-1.45210972673924));
#46286=CARTESIAN_POINT('Ctrl Pts',(0.100902216552484,0.0959742482720097,
-1.44416243543129));
#46287=CARTESIAN_POINT('Ctrl Pts',(-0.0260621287465163,0.13679575681205,
-1.43621514412334));
#46288=CARTESIAN_POINT('Ctrl Pts',(-0.129122678671555,0.052150239589711,
-1.42826785281539));
#46289=CARTESIAN_POINT('Ctrl Pts',(-0.113753835544216,-0.0803266987717117,
-1.42032056150743));
#46290=CARTESIAN_POINT('Ctrl Pts',(0.0059483271787393,-0.139129188312001,
-1.41237327019948));
#46291=CARTESIAN_POINT('Ctrl Pts',(0.120194773022965,-0.0703244635567145,
-1.40442597889153));
#46292=CARTESIAN_POINT('Ctrl Pts',(0.12420036758044,0.0629808092157078,
-1.39647868758358));
#46293=CARTESIAN_POINT('Ctrl Pts',(0.0142912393273046,0.138521024090466,
-1.38853139627563));
#46294=CARTESIAN_POINT('Ctrl Pts',(-0.108725600266021,0.0870118238136351,
-1.38058410496768));
#46295=CARTESIAN_POINT('Ctrl Pts',(-0.13202094258842,-0.0443033221626407,
-1.37263681365972));
#46296=CARTESIAN_POINT('Ctrl Pts',(-0.0342286474655051,-0.134984122508034,
-1.36468952235177));
#46297=CARTESIAN_POINT('Ctrl Pts',(0.0949576520728147,-0.10185950102666,
-1.35674223104382));
#46298=CARTESIAN_POINT('Ctrl Pts',(0.137050210865036,0.0246891340154153,
-1.34879493973587));
#46299=CARTESIAN_POINT('Ctrl Pts',(0.0534423624365219,0.12859326395183,
-1.34084764842792));
#46300=CARTESIAN_POINT('Ctrl Pts',(-0.0791820229145371,0.114553572112542,
-1.33290035711997));
#46301=CARTESIAN_POINT('Ctrl Pts',(-0.139181839050446,-0.00455294576261637,
-1.32495306581201));
#46302=CARTESIAN_POINT('Ctrl Pts',(-0.0715261504195623,-0.119483569760616,
-1.31700577450407));
#46303=CARTESIAN_POINT('Ctrl Pts',(0.0617322554776575,-0.124825647485695,
-1.30905848319611));
#46304=CARTESIAN_POINT('Ctrl Pts',(0.138370758324617,-0.0156795050066074,
-1.30111119188816));
#46305=CARTESIAN_POINT('Ctrl Pts',(0.0880976675369301,0.107847645366666,
-1.29316390058021));
#46306=CARTESIAN_POINT('Ctrl Pts',(-0.0429772886013641,0.132458545594676,
-1.28521660927226));
#46307=CARTESIAN_POINT('Ctrl Pts',(-0.134634117293255,0.0355804454335238,
-1.27726931796431));
#46308=CARTESIAN_POINT('Ctrl Pts',(-0.10280654371573,-0.0939315080567081,
-1.26932202665635));
#46309=CARTESIAN_POINT('Ctrl Pts',(0.0233136568373885,-0.137290884771896,
-1.2613747353484));
#46310=CARTESIAN_POINT('Ctrl Pts',(0.128050919416408,-0.0547291117522856,
-1.25342744404045));
#46311=CARTESIAN_POINT('Ctrl Pts',(0.115341790530312,0.0780293854508893,
-1.2454801527325));
#46312=CARTESIAN_POINT('Ctrl Pts',(-0.003157106556191,0.139220495311483,
-1.23753286142455));
#46313=CARTESIAN_POINT('Ctrl Pts',(-0.118760352645532,0.0727206454598038,
-1.2295855701166));
#46314=CARTESIAN_POINT('Ctrl Pts',(-0.125438376402145,-0.0604774946750888,
-1.22163827880865));
#46315=CARTESIAN_POINT('Ctrl Pts',(-0.01706619414058,-0.138206579634031,
-1.21369098750069));
#46316=CARTESIAN_POINT('Ctrl Pts',(0.106958846585331,-0.0891746532021148,
-1.20574369619274));
#46317=CARTESIAN_POINT('Ctrl Pts',(0.132882830138289,0.0416469337529245,
-1.19779640488479));
#46318=CARTESIAN_POINT('Ctrl Pts',(0.036928665853329,0.134270574866107,
-1.18984911357684));
#46319=CARTESIAN_POINT('Ctrl Pts',(-0.0928959194005778,0.103743249396301,
-1.18190182226889));
#46320=CARTESIAN_POINT('Ctrl Pts',(-0.137517754333317,-0.0219358355141317,
-1.17395453096093));
#46321=CARTESIAN_POINT('Ctrl Pts',(-0.0560103581567255,-0.127495699597034,
-1.16600723965299));
#46322=CARTESIAN_POINT('Ctrl Pts',(0.0768689022763401,-0.116118411543615,
-1.15805994834503));
#46323=CARTESIAN_POINT('Ctrl Pts',(0.139245153208294,0.00176094990851802,
-1.15011265703708));
#46324=CARTESIAN_POINT('Ctrl Pts',(0.0739078285731691,0.118025194395861,
-1.14216536572913));
#46325=CARTESIAN_POINT('Ctrl Pts',(-0.0592166529718895,0.126038492721028,
-1.13421807442118));
#46326=CARTESIAN_POINT('Ctrl Pts',(-0.138028504526574,0.0184511673001812,
-1.12627078311322));
#46327=CARTESIAN_POINT('Ctrl Pts',(-0.0902426725202642,-0.106059293289094,
-1.11832349180528));
#46328=CARTESIAN_POINT('Ctrl Pts',(0.0403123913820496,-0.13329375355823,
-1.11037620049732));
#46329=CARTESIAN_POINT('Ctrl Pts',(0.133893531780113,-0.0382731731638424,
-1.10242890918937));
#46330=CARTESIAN_POINT('Ctrl Pts',(0.10466952388434,0.0918509902309573,
-1.09448161788142));
#46331=CARTESIAN_POINT('Ctrl Pts',(-0.0205558085830443,0.137730796737981,
-1.08653432657347));
#46332=CARTESIAN_POINT('Ctrl Pts',(-0.126927660320036,0.0572859728228762,
-1.07858703526552));
#46333=CARTESIAN_POINT('Ctrl Pts',(-0.116883357064639,-0.0757006900753334,
-1.07063974395756));
#46334=CARTESIAN_POINT('Ctrl Pts',(0.00036461620057585,-0.139255810261576,
-1.06269245264961));
#46335=CARTESIAN_POINT('Ctrl Pts',(0.117278168930411,-0.0750875803905805,
-1.05474516134166));
#46336=CARTESIAN_POINT('Ctrl Pts',(0.126625936101752,0.0579498571433683,
-1.04679787003371));
#46337=CARTESIAN_POINT('Ctrl Pts',(0.0198342852289171,0.137836550907369,
-1.03885057872576));
#46338=CARTESIAN_POINT('Ctrl Pts',(-0.105149075926379,0.0913016181040087,
-1.03090328741781));
#46339=CARTESIAN_POINT('Ctrl Pts',(-0.133691274536908,-0.0389737956745147,
-1.02295599610985));
#46340=CARTESIAN_POINT('Ctrl Pts',(-0.0396138321773288,-0.133503025946263,
-1.0150087048019));
#46341=CARTESIAN_POINT('Ctrl Pts',(0.0907968256135503,-0.105585274044654,
-1.00706141349395));
#46342=CARTESIAN_POINT('Ctrl Pts',(0.137929990564865,0.0191737148032896,
-0.999114122186));
#46343=CARTESIAN_POINT('Ctrl Pts',(0.0585558274900352,0.126346858700717,
-0.991166830878047));
#46344=CARTESIAN_POINT('Ctrl Pts',(-0.0745248663094564,0.117636550179523,
-0.983219539570098));
#46345=CARTESIAN_POINT('Ctrl Pts',(-0.139252465399779,0.00103175416884905,
-0.975272248262143));
#46346=CARTESIAN_POINT('Ctrl Pts',(-0.0762597822901658,-0.116519351361215,
-0.967324956954194));
#46347=CARTESIAN_POINT('Ctrl Pts',(0.0566772345635106,-0.127200647477969,
-0.959377665646241));
#46348=CARTESIAN_POINT('Ctrl Pts',(0.137630738076998,-0.0212154088568283,
-0.95143037433829));
#46349=CARTESIAN_POINT('Ctrl Pts',(0.0923513834783183,0.104228286017869,
-0.943483083030339));
#46350=CARTESIAN_POINT('Ctrl Pts',(-0.0376312812236582,0.13407535310432,
-0.935535791722386));
#46351=CARTESIAN_POINT('Ctrl Pts',(-0.133099096629194,0.0409505080929924,
-0.927588500414435));
#46352=CARTESIAN_POINT('Ctrl Pts',(-0.106490407800252,-0.0897335315426603,
-0.919641209106483));
#46353=CARTESIAN_POINT('Ctrl Pts',(0.017789693141843,-0.1381153157854,-0.911693917798532));
#46354=CARTESIAN_POINT('Ctrl Pts',(0.125753353137608,-0.0598197944766599,
-0.90374662649058));
#46355=CARTESIAN_POINT('Ctrl Pts',(0.118377915156088,0.0733415492056153,
-0.895799335182628));
#46356=CARTESIAN_POINT('Ctrl Pts',(0.00242802079729554,0.139235118959227,
-0.887852043874677));
#46357=CARTESIAN_POINT('Ctrl Pts',(-0.115748817985984,0.0774243164091847,
-0.879904752566726));
#46358=CARTESIAN_POINT('Ctrl Pts',(-0.127762569063506,-0.0553989131921782,
-0.871957461258773));
#46359=CARTESIAN_POINT('Ctrl Pts',(-0.0225943993144704,-0.137411086729565,
-0.864010169950823));
#46360=CARTESIAN_POINT('Ctrl Pts',(0.103297016147289,-0.0933918630912153,
-0.856062878642869));
#46361=CARTESIAN_POINT('Ctrl Pts',(0.134445950642072,0.0362849830168238,
-0.848115587334919));
#46362=CARTESIAN_POINT('Ctrl Pts',(0.0422830665105441,0.132681784443256,
-0.840168296026967));
#46363=CARTESIAN_POINT('Ctrl Pts',(-0.0886612149305494,0.107384834141608,
-0.832221004719016));
#46364=CARTESIAN_POINT('Ctrl Pts',(-0.138286753765475,-0.0164038827595369,
-0.824273713411065));
#46365=CARTESIAN_POINT('Ctrl Pts',(-0.0610777466931965,-0.1251472033066,
-0.816326422103112));
#46366=CARTESIAN_POINT('Ctrl Pts',(0.0721508577441712,-0.119107377451451,
-0.808379130795161));
#46367=CARTESIAN_POINT('Ctrl Pts',(0.139203772684067,-0.00382404329272468,
-0.800431839487209));
#46368=CARTESIAN_POINT('Ctrl Pts',(0.0785810656558809,0.114966646280423,
-0.792484548179258));
#46369=CARTESIAN_POINT('Ctrl Pts',(-0.0541150215622158,0.12831164435819,
-0.784537256871306));
#46370=CARTESIAN_POINT('Ctrl Pts',(-0.137177618950604,0.0239711179469101,
-0.776589965563354));
#46371=CARTESIAN_POINT('Ctrl Pts',(-0.0944229523244023,-0.102355359952107,
-0.768642674255403));
#46372=CARTESIAN_POINT('Ctrl Pts',(0.0349350364218175,-0.134803029887269,
-0.760695382947452));
#46373=CARTESIAN_POINT('Ctrl Pts',(0.132251131348421,-0.0436113734436843,
-0.752748091639499));
#46374=CARTESIAN_POINT('Ctrl Pts',(0.108268463135797,0.087579983596677,
-0.744800800331548));
#46375=CARTESIAN_POINT('Ctrl Pts',(-0.0150164229970535,0.138444287267318,
-0.736853509023596));
#46376=CARTESIAN_POINT('Ctrl Pts',(-0.124528470154946,0.0623295576548628,
-0.728906217715645));
#46377=CARTESIAN_POINT('Ctrl Pts',(-0.119824863719519,-0.0709529116469537,
-0.720958926407693));
#46378=CARTESIAN_POINT('Ctrl Pts',(-0.00521968128764912,-0.139158429726111,
-0.713011635099741));
#46379=CARTESIAN_POINT('Ctrl Pts',(0.114172914890457,-0.0797299137212506,
-0.705064343791791));
#46380=CARTESIAN_POINT('Ctrl Pts',(0.128847818153508,0.0528256887665676,
-0.697117052483838));
#46381=CARTESIAN_POINT('Ctrl Pts',(0.0253454263276182,0.136930358214871,
-0.689169761175887));
#46382=CARTESIAN_POINT('Ctrl Pts',(-0.101403412114119,0.0954445475037516,
-0.681222469867934));
#46383=CARTESIAN_POINT('Ctrl Pts',(-0.135146554936249,-0.0335815771732833,
-0.673275178559984));
#46384=CARTESIAN_POINT('Ctrl Pts',(-0.0449352953335994,-0.131807180646063,
-0.665327887252032));
#46385=CARTESIAN_POINT('Ctrl Pts',(0.086489946256864,-0.109141205935553,
-0.657380595944081));
#46386=CARTESIAN_POINT('Ctrl Pts',(0.138587900451223,0.0136274533609135,
-0.649433304636128));
#46387=CARTESIAN_POINT('Ctrl Pts',(0.0635751014943803,0.123897215895116,
-0.641486013328178));
#46388=CARTESIAN_POINT('Ctrl Pts',(-0.0697478313652302,0.120530301818377,
-0.633538722020224));
#46389=CARTESIAN_POINT('Ctrl Pts',(-0.139099094644512,0.00661479445324233,
-0.625591430712274));
#46390=CARTESIAN_POINT('Ctrl Pts',(-0.0808707450907354,-0.113367703624317,
-0.617644139404322));
#46391=CARTESIAN_POINT('Ctrl Pts',(0.0515310444452701,-0.129371036538173,
-0.609696848096371));
#46392=CARTESIAN_POINT('Ctrl Pts',(0.136669329383979,-0.0267171862724199,
-0.601749556788419));
#46393=CARTESIAN_POINT('Ctrl Pts',(0.0964565459097508,0.100441268349926,
-0.593802265480467));
#46394=CARTESIAN_POINT('Ctrl Pts',(-0.0322247413590565,0.135476491248201,
-0.585854974172516));
#46395=CARTESIAN_POINT('Ctrl Pts',(-0.131349976974611,0.0462546990623779,
-0.577907682864563));
#46396=CARTESIAN_POINT('Ctrl Pts',(-0.110002974788192,-0.0853912125123539,
-0.569960391556613));
#46397=CARTESIAN_POINT('Ctrl Pts',(0.0122371135094518,-0.13871757887715,
-0.562013100248661));
#46398=CARTESIAN_POINT('Ctrl Pts',(0.123253503998567,-0.0648142529746122,
-0.554065808940709));
#46399=CARTESIAN_POINT('Ctrl Pts',(0.121223620817521,0.0685357380676061,
-0.546118517632758));
#46400=CARTESIAN_POINT('Ctrl Pts',(0.00800924251344417,0.139025773405302,
-0.538171226324806));
#46401=CARTESIAN_POINT('Ctrl Pts',(-0.112551093444511,0.0820034450558435,
-0.530223935016855));
#46402=CARTESIAN_POINT('Ctrl Pts',(-0.129881246903541,-0.0502312187724236,
-0.522276643708902));
#46403=CARTESIAN_POINT('Ctrl Pts',(-0.0280862598533812,-0.136394558703894,
-0.514329352400952));
#46404=CARTESIAN_POINT('Ctrl Pts',(0.0994690254013135,-0.0974588457878242,
-0.506382061092999));
#46405=CARTESIAN_POINT('Ctrl Pts',(0.135792805648636,0.0308646654064759,
-0.498434769785048));
#46406=CARTESIAN_POINT('Ctrl Pts',(0.0475694519664141,0.130879566305045,
-0.490487478477097));
#46407=CARTESIAN_POINT('Ctrl Pts',(-0.0842838928387955,0.110853683044453,
-0.482540187169144));
#46408=CARTESIAN_POINT('Ctrl Pts',(-0.138833309506175,-0.0108455432387773,
-0.474592895861194));
#46409=CARTESIAN_POINT('Ctrl Pts',(-0.0660468875011581,-0.122597399189343,
-0.466645604553241));
#46410=CARTESIAN_POINT('Ctrl Pts',(0.0673167536278285,-0.121904751005003,
-0.45869831324529));
#46411=CARTESIAN_POINT('Ctrl Pts',(0.138938473380797,-0.00940288525907187,
-0.450751021937338));
#46412=CARTESIAN_POINT('Ctrl Pts',(0.0831278997256812,0.111723166459686,
-0.442803730629387));
#46413=CARTESIAN_POINT('Ctrl Pts',(-0.0489263424431069,0.1303783979489,
-0.434856439321435));
#46414=CARTESIAN_POINT('Ctrl Pts',(-0.136106073802305,0.0294525094126708,
-0.426909148013483));
#46415=CARTESIAN_POINT('Ctrl Pts',(-0.0984513463585633,-0.0984867810255157,
-0.418961856705532));
#46416=CARTESIAN_POINT('Ctrl Pts',(0.0295014860686701,-0.136095466332724,
-0.41101456539758));
#46417=CARTESIAN_POINT('Ctrl Pts',(0.130395995936294,-0.0488794218497269,
-0.403067274089629));
#46418=CARTESIAN_POINT('Ctrl Pts',(0.111693245167184,0.083168098575145,
-0.395119982781677));
#46419=CARTESIAN_POINT('Ctrl Pts',(-0.00945288246871811,0.138935080701795,
-0.387172691473725));
#46420=CARTESIAN_POINT('Ctrl Pts',(-0.121928967437574,0.0672728811348881,
-0.379225400165774));
#46421=CARTESIAN_POINT('Ctrl Pts',(-0.122573623894439,-0.0660910006125364,
-0.371278108857823));
#46422=CARTESIAN_POINT('Ctrl Pts',(-0.0107955825619163,-0.138837203348852,
-0.363330817549871));
#46423=CARTESIAN_POINT('Ctrl Pts',(0.11088400591638,-0.0842439960384028,
-0.35538352624192));
#46424=CARTESIAN_POINT('Ctrl Pts',(0.130862439686628,0.0476165466602282,
-0.347436234933967));
#46425=CARTESIAN_POINT('Ctrl Pts',(0.0308157975764226,0.135803903685831,
-0.339488943626016));
#46426=CARTESIAN_POINT('Ctrl Pts',(-0.0974946339853923,0.099433947827876,
-0.331541652318064));
#46427=CARTESIAN_POINT('Ctrl Pts',(-0.136384442868491,-0.0281353404108124,
-0.323594361010113));
#46428=CARTESIAN_POINT('Ctrl Pts',(-0.0501844769972613,-0.129899314490461,
-0.315647069702161));
#46429=CARTESIAN_POINT('Ctrl Pts',(0.0820439419124697,-0.112521576739974,
-0.30769977839421));
#46430=CARTESIAN_POINT('Ctrl Pts',(0.139022882231082,0.00805927122877484,
-0.299752487086258));
#46431=CARTESIAN_POINT('Ctrl Pts',(0.0684921106044416,0.12124827595279,
-0.291805195778306));
#46432=CARTESIAN_POINT('Ctrl Pts',(-0.0648586022690144,0.123230172231987,
-0.283857904470355));
#46433=CARTESIAN_POINT('Ctrl Pts',(-0.138721973491842,0.0121871943886424,
-0.275910613162403));
#46434=CARTESIAN_POINT('Ctrl Pts',(-0.0853516217728486,-0.110033696190289,
-0.267963321854451));
#46435=CARTESIAN_POINT('Ctrl Pts',(0.0463019631218519,-0.131333323447874,
-0.2600160305465));
#46436=CARTESIAN_POINT('Ctrl Pts',(0.135488078736147,-0.0321759872672793,
-0.252068739238548));
#46437=CARTESIAN_POINT('Ctrl Pts',(0.100406551398842,0.0964926840371405,
-0.244121447930597));
#46438=CARTESIAN_POINT('Ctrl Pts',(-0.0267663657998475,0.136659706204361,
-0.236174156622645));
#46439=CARTESIAN_POINT('Ctrl Pts',(-0.129389571901277,0.051484486179617,
-0.228226865314693));
#46440=CARTESIAN_POINT('Ctrl Pts',(-0.113338594488273,-0.080911535866496,
-0.220279574006742));
#46441=CARTESIAN_POINT('Ctrl Pts',(0.00666484966802229,-0.139096705296418,
-0.21233228269879));
#46442=CARTESIAN_POINT('Ctrl Pts',(0.12055539313165,-0.0697044532603406,
-0.204384991390839));
#46443=CARTESIAN_POINT('Ctrl Pts',(0.123874330089505,0.0636196824021741,
-0.196437700082887));
#46444=CARTESIAN_POINT('Ctrl Pts',(0.0135775806509123,0.138592795605587,
-0.188490408774936));
#46445=CARTESIAN_POINT('Ctrl Pts',(-0.109172322466555,0.0864506651613264,
-0.180543117466983));
#46446=CARTESIAN_POINT('Ctrl Pts',(-0.131791002478216,-0.0449827232515467,
-0.172595826159032));
#46447=CARTESIAN_POINT('Ctrl Pts',(-0.0335329405968919,-0.135158632142634,
-0.16464853485108));
#46448=CARTESIAN_POINT('Ctrl Pts',(0.0954810297919763,-0.101369056556591,
-0.156701243543129));
#46449=CARTESIAN_POINT('Ctrl Pts',(0.136921232711689,0.0253946947183125,
-0.148753952235177));
#46450=CARTESIAN_POINT('Ctrl Pts',(0.0527793109988149,0.128866829226554,
-0.140806660927226));
#46451=CARTESIAN_POINT('Ctrl Pts',(-0.0797709797129985,0.114144197653596,
-0.132859369619274));
#46452=CARTESIAN_POINT('Ctrl Pts',(-0.139156570159351,-0.00526972267221474,
-0.124912078311322));
#46453=CARTESIAN_POINT('Ctrl Pts',(-0.0709097346571945,-0.11985045568327,
-0.116964787003371));
#46454=CARTESIAN_POINT('Ctrl Pts',(0.0623742658464559,-0.124505905450053,
-0.109017495695419));
#46455=CARTESIAN_POINT('Ctrl Pts',(0.138449871985116,-0.0149668430727117,
-0.101070204387468));
#46456=CARTESIAN_POINT('Ctrl Pts',(0.0875406563815945,0.108300429783857,
-0.093122913079516));
#46457=CARTESIAN_POINT('Ctrl Pts',(-0.0436582776930319,0.132234560631268,
-0.0851756217715646));
#46458=CARTESIAN_POINT('Ctrl Pts',(-0.134816891517839,0.0348881726866265,
-0.0772283304636131));
#46459=CARTESIAN_POINT('Ctrl Pts',(-0.102318909486457,-0.0944629077688085,
-0.0692810391556614));
#46460=CARTESIAN_POINT('Ctrl Pts',(0.0240158013170603,-0.137163045762996,
-0.0613337478477098));
#46461=CARTESIAN_POINT('Ctrl Pts',(0.128339992499329,-0.0540801177957914,
-0.0533864565397582));
#46462=CARTESIAN_POINT('Ctrl Pts',(0.114921489370477,0.0786438502502632,
-0.0454391652318065));
#46463=CARTESIAN_POINT('Ctrl Pts',(-0.0038420162804081,0.139161560048721,
-0.0374918739238548));
#46464=CARTESIAN_POINT('Ctrl Pts',(-0.119195118024918,0.0721869595400255,
-0.0295445826159032));
#46465=CARTESIAN_POINT('Ctrl Pts',(-0.125001006615905,-0.0612850510018785,
-0.0215972913079518));
#46466=CARTESIAN_POINT('Ctrl Pts',(-0.0527668217477812,-0.112355607212729,
-0.0162990971026507));
#46467=CARTESIAN_POINT('Ctrl Pts',(-0.0138313775859597,-0.116960008631475,
-0.0136500000000002));
#46468=CARTESIAN_POINT('Ctrl Pts',(0.112054873528411,-0.0604069144927277,
-2.94864852262806));
#46469=CARTESIAN_POINT('Ctrl Pts',(0.132164055066097,-0.0231043670461693,
-2.94599942552541));
#46470=CARTESIAN_POINT('Ctrl Pts',(0.131850069163285,0.0725142137010918,
-2.94070123132011));
#46471=CARTESIAN_POINT('Ctrl Pts',(0.0101729848055668,0.150275971928739,
-2.93275394001216));
#46472=CARTESIAN_POINT('Ctrl Pts',(-0.120717947947423,0.0898301286852705,
-2.92480664870421));
#46473=CARTESIAN_POINT('Ctrl Pts',(-0.14094563806992,-0.0528164143684709,
-2.91685935739625));
#46474=CARTESIAN_POINT('Ctrl Pts',(-0.0318703010347745,-0.147119726764245,
-2.90891206608831));
#46475=CARTESIAN_POINT('Ctrl Pts',(0.106420360777253,-0.106434877139951,
-2.90096477478035));
#46476=CARTESIAN_POINT('Ctrl Pts',(0.147112089588147,0.0318429936417547,
-2.8930174834724));
#46477=CARTESIAN_POINT('Ctrl Pts',(0.0528704694334625,0.140929411341517,
-2.88507019216445));
#46478=CARTESIAN_POINT('Ctrl Pts',(-0.0898608711538647,0.120749856183999,
-2.8771229008565));
#46479=CARTESIAN_POINT('Ctrl Pts',(-0.150174366082989,-0.0101756491885928,
-2.86917560954855));
#46480=CARTESIAN_POINT('Ctrl Pts',(-0.0727495403866633,-0.131770316393393,
-2.8612283182406));
#46481=CARTESIAN_POINT('Ctrl Pts',(0.0713997434663159,-0.13250610228209,
-2.85328102693264));
#46482=CARTESIAN_POINT('Ctrl Pts',(0.150062424656416,-0.0117098566624688,
-2.8453337356247));
#46483=CARTESIAN_POINT('Ctrl Pts',(0.0910899976674201,0.119826804007082,
-2.83738644431673));
#46484=CARTESIAN_POINT('Ctrl Pts',(-0.0514287663295641,0.141459946095722,
-2.82943915300879));
#46485=CARTESIAN_POINT('Ctrl Pts',(-0.146777859433181,0.0333482235155928,
-2.82149186170084));
#46486=CARTESIAN_POINT('Ctrl Pts',(-0.107504477722029,-0.105350037017472,
-2.81354457039289));
#46487=CARTESIAN_POINT('Ctrl Pts',(0.0303703987486264,-0.147422792658834,
-2.80559727908493));
#46488=CARTESIAN_POINT('Ctrl Pts',(0.140390002687352,-0.0542815764800469,
-2.79764998777698));
#46489=CARTESIAN_POINT('Ctrl Pts',(0.121645990226168,0.0886458978282491,
-2.78970269646903));
#46490=CARTESIAN_POINT('Ctrl Pts',(-0.00866990722862085,0.150268674662333,
-2.78175540516108));
#46491=CARTESIAN_POINT('Ctrl Pts',(-0.131033895767171,0.0740672684712725,
-2.77380811385313));
#46492=CARTESIAN_POINT('Ctrl Pts',(-0.133215551178006,-0.0700675314913027,
-2.76586082254518));
#46493=CARTESIAN_POINT('Ctrl Pts',(-0.0132138921336998,-0.149937437181362,
-2.75791353123723));
#46494=CARTESIAN_POINT('Ctrl Pts',(0.118907351570326,-0.0922869643505502,
-2.74996623992927));
#46495=CARTESIAN_POINT('Ctrl Pts',(0.141968547680105,0.0500077344628434,
-2.74201894862132));
#46496=CARTESIAN_POINT('Ctrl Pts',(0.0348183114963835,0.146436085776981,
-2.73407165731337));
#46497=CARTESIAN_POINT('Ctrl Pts',(-0.104266760159845,0.108555445573249,
-2.72612436600542));
#46498=CARTESIAN_POINT('Ctrl Pts',(-0.147719916113032,-0.0288906285783304,
-2.71817707469747));
#46499=CARTESIAN_POINT('Ctrl Pts',(-0.0556865704959391,-0.139838649529325,
-2.71022978338951));
#46500=CARTESIAN_POINT('Ctrl Pts',(0.0874216661710837,-0.122528748954342,
-2.70228249208156));
#46501=CARTESIAN_POINT('Ctrl Pts',(0.150348055846523,0.00716269078799115,
-2.69433520077361));
#46502=CARTESIAN_POINT('Ctrl Pts',(0.0753774534239399,0.130284617478266,
-2.68638790946566));
#46503=CARTESIAN_POINT('Ctrl Pts',(-0.0687282238801868,0.133911438191447,
-2.67844061815771));
#46504=CARTESIAN_POINT('Ctrl Pts',(-0.149797400366207,0.0147166871172186,
-2.67049332684976));
#46505=CARTESIAN_POINT('Ctrl Pts',(-0.0934746377389571,-0.117975989657863,
-2.6625460355418));
#46506=CARTESIAN_POINT('Ctrl Pts',(0.0485816670290888,-0.142462850121947,
-2.65459874423386));
#46507=CARTESIAN_POINT('Ctrl Pts',(0.146079592131197,-0.0362849114504862,
-2.6466514529259));
#46508=CARTESIAN_POINT('Ctrl Pts',(0.109595496325569,0.103173006262973,
-2.63870416161795));
#46509=CARTESIAN_POINT('Ctrl Pts',(-0.0274079524291007,0.148002183023876,
-2.63075687031));
#46510=CARTESIAN_POINT('Ctrl Pts',(-0.139273236421531,0.0570859672148926,
-2.62280957900205));
#46511=CARTESIAN_POINT('Ctrl Pts',(-0.12339918734299,-0.0861886454196691,
-2.61486228769409));
#46512=CARTESIAN_POINT('Ctrl Pts',(0.00565475399413943,-0.15041231928753,
-2.60691499638615));
#46513=CARTESIAN_POINT('Ctrl Pts',(0.129522239394354,-0.076680059588263,
-2.59896770507819));
#46514=CARTESIAN_POINT('Ctrl Pts',(0.134593860612755,0.0673820059180649,
-2.59102041377024));
#46515=CARTESIAN_POINT('Ctrl Pts',(0.0162180023880564,0.149642301621998,
-2.58307312246229));
#46516=CARTESIAN_POINT('Ctrl Pts',(-0.11703276548923,0.0946529124651258,
-2.57512583115434));
#46517=CARTESIAN_POINT('Ctrl Pts',(-0.142942828180357,-0.0471507148194896,
-2.56717853984639));
#46518=CARTESIAN_POINT('Ctrl Pts',(-0.0377478630269907,-0.145708410440453,
-2.55923124853843));
#46519=CARTESIAN_POINT('Ctrl Pts',(0.102068878512243,-0.110624527458611,
-2.55128395723048));
#46520=CARTESIAN_POINT('Ctrl Pts',(0.148269568587044,0.0259225204638712,
-2.54333666592253));
#46521=CARTESIAN_POINT('Ctrl Pts',(0.058479624045545,0.138693819644855,
-2.53538937461458));
#46522=CARTESIAN_POINT('Ctrl Pts',(-0.0849469585590607,0.124257218171634,
-2.52744208330663));
#46523=CARTESIAN_POINT('Ctrl Pts',(-0.1504614590469,-0.00414624862564929,
-2.51949479199867));
#46524=CARTESIAN_POINT('Ctrl Pts',(-0.0779749557139858,-0.128746838087737,
-2.51154750069073));
#46525=CARTESIAN_POINT('Ctrl Pts',(0.0660290128194679,-0.135262749869557,
-2.50360020938277));
#46526=CARTESIAN_POINT('Ctrl Pts',(0.149472156620126,-0.0177176869685779,
-2.49565291807483));
#46527=CARTESIAN_POINT('Ctrl Pts',(0.0958216700153998,0.116077773891679,
-2.48770562676686));
#46528=CARTESIAN_POINT('Ctrl Pts',(-0.0457150216924184,0.143408433600851,
-2.47975833545893));
#46529=CARTESIAN_POINT('Ctrl Pts',(-0.145322578037573,0.0392070191254258,
-2.47181104415096));
#46530=CARTESIAN_POINT('Ctrl Pts',(-0.111642435499295,-0.100954487923884,
-2.46386375284302));
#46531=CARTESIAN_POINT('Ctrl Pts',(0.0244344820369845,-0.148522045918349,
-2.45591646153506));
#46532=CARTESIAN_POINT('Ctrl Pts',(0.138100457460221,-0.0598674008577744,
-2.44796917022712));
#46533=CARTESIAN_POINT('Ctrl Pts',(0.125102755165994,0.0836967304383223,
-2.44002187891916));
#46534=CARTESIAN_POINT('Ctrl Pts',(-0.00263732635950105,0.150495470183861,
-2.43207458761121));
#46535=CARTESIAN_POINT('Ctrl Pts',(-0.127958491523826,0.0792620116016167,
-2.42412729630325));
#46536=CARTESIAN_POINT('Ctrl Pts',(-0.135918038706145,-0.0646693806253223,
-2.41618000499531));
#46537=CARTESIAN_POINT('Ctrl Pts',(-0.0192155900683274,-0.149286982468378,
-2.40823271368735));
#46538=CARTESIAN_POINT('Ctrl Pts',(0.115111110887891,-0.0969807928733496,
-2.4002854223794));
#46539=CARTESIAN_POINT('Ctrl Pts',(0.143859619567644,0.0442747320041667,
-2.39233813107145));
#46540=CARTESIAN_POINT('Ctrl Pts',(0.0406622330303461,0.144922133717295,
-2.3843908397635));
#46541=CARTESIAN_POINT('Ctrl Pts',(-0.0998299465478195,0.112649118098844,
-2.37644354845555));
#46542=CARTESIAN_POINT('Ctrl Pts',(-0.148759589631659,-0.0229439867679609,
-2.3684962571476));
#46543=CARTESIAN_POINT('Ctrl Pts',(-0.0612491581131811,-0.137493209529105,
-2.36054896583964));
#46544=CARTESIAN_POINT('Ctrl Pts',(0.0824380867655902,-0.125935713308882,
-2.35260167453169));
#46545=CARTESIAN_POINT('Ctrl Pts',(0.150514349278652,0.0011281389150487,
-2.34465438322374));
#46546=CARTESIAN_POINT('Ctrl Pts',(0.0805410978400582,0.127157278969417,
-2.33670709191579));
#46547=CARTESIAN_POINT('Ctrl Pts',(-0.063303246044138,0.136559661234433,
-2.32875980060784));
#46548=CARTESIAN_POINT('Ctrl Pts',(-0.149086797785675,0.020711561075909,
-2.32081250929989));
#46549=CARTESIAN_POINT('Ctrl Pts',(-0.0981301644913087,-0.11413287367405,
-2.31286521799193));
#46550=CARTESIAN_POINT('Ctrl Pts',(0.0428299905732093,-0.144296340714818,
-2.30491792668398));
#46551=CARTESIAN_POINT('Ctrl Pts',(0.144507117743561,-0.0421133584226735,
-2.29697063537603));
#46552=CARTESIAN_POINT('Ctrl Pts',(0.113644474037177,0.0986953674546136,
-2.28902334406808));
#46553=CARTESIAN_POINT('Ctrl Pts',(-0.0214511845233532,0.148982175842391,
-2.28107605276013));
#46554=CARTESIAN_POINT('Ctrl Pts',(-0.136872136909167,0.0626247568786199,
-2.27312876145218));
#46555=CARTESIAN_POINT('Ctrl Pts',(-0.126756008847893,-0.0811711540951639,
-2.26518147014422));
#46556=CARTESIAN_POINT('Ctrl Pts',(-0.000381161961692621,-0.150518094433018,
-2.25723417883628));
#46557=CARTESIAN_POINT('Ctrl Pts',(0.126343280984955,-0.081812085819546,
-2.24928688752832));
#46558=CARTESIAN_POINT('Ctrl Pts',(0.13718755294046,0.0619307464382313,
-2.24133959622038));
#46559=CARTESIAN_POINT('Ctrl Pts',(0.0222054495741949,0.148871622700217,
-2.23339230491242));
#46560=CARTESIAN_POINT('Ctrl Pts',(-0.113143160610104,0.0992696693020791,
-2.22544501360447));
#46561=CARTESIAN_POINT('Ctrl Pts',(-0.144718553130867,-0.0413809426656339,
-2.21749772229651));
#46562=CARTESIAN_POINT('Ctrl Pts',(-0.0435602493944256,-0.144077571845459,
-2.20955043098857));
#46563=CARTESIAN_POINT('Ctrl Pts',(0.0975508647241037,-0.114628403233089,
-2.20160313968061));
#46564=CARTESIAN_POINT('Ctrl Pts',(0.14918978216991,0.0199562254016758,
-2.19365584837266));
#46565=CARTESIAN_POINT('Ctrl Pts',(0.0639940588401701,0.136237302048113,
-2.18570855706471));
#46566=CARTESIAN_POINT('Ctrl Pts',(-0.0798960598147894,0.127563559303821,
-2.17776126575676));
#46567=CARTESIAN_POINT('Ctrl Pts',(-0.150506705270388,0.00189042451330132,
-2.1698139744488));
#46568=CARTESIAN_POINT('Ctrl Pts',(-0.0830748477445828,-0.125516579416435,
-2.16186668314085));
#46569=CARTESIAN_POINT('Ctrl Pts',(0.0605520198099057,-0.13780165069087,
-2.1539193918329));
#46570=CARTESIAN_POINT('Ctrl Pts',(0.148641478847462,-0.0236971053554501,
-2.14597210052495));
#46571=CARTESIAN_POINT('Ctrl Pts',(0.100399192730552,0.112142071209878,
-2.138024809217));
#46572=CARTESIAN_POINT('Ctrl Pts',(-0.0399277339805376,0.14512621436311,
-2.13007751790905));
#46573=CARTESIAN_POINT('Ctrl Pts',(-0.143633539213038,0.0450027604633815,
-2.1221302266011));
#46574=CARTESIAN_POINT('Ctrl Pts',(-0.115600806754312,-0.0963965534339281,
-2.11418293529314));
#46575=CARTESIAN_POINT('Ctrl Pts',(0.0184592597183131,-0.149382387739786,
-2.1062356439852));
#46576=CARTESIAN_POINT('Ctrl Pts',(0.13558876877742,-0.0653569263170418,
-2.09828835267724));
#46577=CARTESIAN_POINT('Ctrl Pts',(0.128358283478957,0.0786129321328472,
-2.09034106136929));
#46578=CARTESIAN_POINT('Ctrl Pts',(0.00339949698620866,0.150480182935922,
-2.08239377006134));
#46579=CARTESIAN_POINT('Ctrl Pts',(-0.124677257387179,0.0843292566467827,
-2.07444647875338));
#46580=CARTESIAN_POINT('Ctrl Pts',(-0.138401892739269,-0.0591672047875833,
-2.06649918744544));
#46581=CARTESIAN_POINT('Ctrl Pts',(-0.0251863784364351,-0.148396389367951,
-2.05855189613748));
#46582=CARTESIAN_POINT('Ctrl Pts',(0.111129706131067,-0.101518621205228,
-2.05060460482953));
#46583=CARTESIAN_POINT('Ctrl Pts',(0.145519283421962,0.038470510635376,
-2.04265731352158));
#46584=CARTESIAN_POINT('Ctrl Pts',(0.0464407465877105,0.143175064492962,
-2.03471002221363));
#46585=CARTESIAN_POINT('Ctrl Pts',(-0.0952325496479617,0.116561586827464,
-2.02676273090568));
#46586=CARTESIAN_POINT('Ctrl Pts',(-0.149559973185881,-0.0169604379904061,
-2.01881543959772));
#46587=CARTESIAN_POINT('Ctrl Pts',(-0.066713222275424,-0.134926602305912,
-2.01086814828978));
#46588=CARTESIAN_POINT('Ctrl Pts',(0.0773219000654605,-0.12914010146525,
-2.00292085698182));
#46589=CARTESIAN_POINT('Ctrl Pts',(0.150438530096393,-0.00490822764595809,
-1.99497356567387));
#46590=CARTESIAN_POINT('Ctrl Pts',(0.0855751863976413,0.12382539928947,
-1.98702627436592));
#46591=CARTESIAN_POINT('Ctrl Pts',(-0.0577764406118648,0.138988218732421,
-1.97907898305797));
#46592=CARTESIAN_POINT('Ctrl Pts',(-0.148136378904979,0.0266731190734859,
-1.97113169175001));
#46593=CARTESIAN_POINT('Ctrl Pts',(-0.102627842169638,-0.110106167165113,
-1.96318440044207));
#46594=CARTESIAN_POINT('Ctrl Pts',(0.0370094191512704,-0.145897720785054,
-1.95523710913411));
#46595=CARTESIAN_POINT('Ctrl Pts',(0.142702193784019,-0.0478740631805581,
-1.94728981782616));
#46596=CARTESIAN_POINT('Ctrl Pts',(0.11751064684788,0.094058970404638,-1.93934252651821));
#46597=CARTESIAN_POINT('Ctrl Pts',(-0.0154599109217152,0.149722520652307,
-1.93139523521026));
#46598=CARTESIAN_POINT('Ctrl Pts',(-0.134250869213207,0.0680628103422581,
-1.92344794390231));
#46599=CARTESIAN_POINT('Ctrl Pts',(-0.129908934652342,-0.0760230934235222,
-1.91550065259436));
#46600=CARTESIAN_POINT('Ctrl Pts',(-0.00641646479246623,-0.150381750939916,
-1.9075533612864));
#46601=CARTESIAN_POINT('Ctrl Pts',(0.122961090776067,-0.0868125117212231,
-1.89960606997845));
#46602=CARTESIAN_POINT('Ctrl Pts',(0.139560569716333,0.0563798671215204,
-1.8916587786705));
#46603=CARTESIAN_POINT('Ctrl Pts',(0.0281571777775729,0.147861473602118,
-1.88371148736255));
#46604=CARTESIAN_POINT('Ctrl Pts',(-0.109071557226972,0.103726744093659,
-1.8757641960546));
#46605=CARTESIAN_POINT('Ctrl Pts',(-0.146261488401206,-0.0355446064382738,
-1.86781690474665));
#46606=CARTESIAN_POINT('Ctrl Pts',(-0.0493025661245861,-0.142214974632486,
-1.85986961343869));
#46607=CARTESIAN_POINT('Ctrl Pts',(0.0928759337051868,-0.118447891389326,
-1.85192232213075));
#46608=CARTESIAN_POINT('Ctrl Pts',(0.149870013795216,0.0139578293874739,
-1.84397503082279));
#46609=CARTESIAN_POINT('Ctrl Pts',(0.0694055548189475,0.133561637443025,
-1.83602773951484));
#46610=CARTESIAN_POINT('Ctrl Pts',(-0.0747166427996508,0.130664705735471,
-1.82808044820689));
#46611=CARTESIAN_POINT('Ctrl Pts',(-0.150309851175531,0.00792405677526355,
-1.82013315689893));
#46612=CARTESIAN_POINT('Ctrl Pts',(-0.0880411082067443,-0.122084418751601,
-1.81218586559099));
#46613=CARTESIAN_POINT('Ctrl Pts',(0.0549776247394447,-0.140118888142166,
-1.80423857428303));
#46614=CARTESIAN_POINT('Ctrl Pts',(0.147571701100593,-0.0296384053293244,
-1.79629128297508));
#46615=CARTESIAN_POINT('Ctrl Pts',(0.104815216484724,0.108025980344769,
-1.78834399166713));
#46616=CARTESIAN_POINT('Ctrl Pts',(-0.0340762197806085,0.146610549694254,
-1.78039670035918));
#46617=CARTESIAN_POINT('Ctrl Pts',(-0.141713456027351,0.0507261117864536,
-1.77244940905122));
#46618=CARTESIAN_POINT('Ctrl Pts',(-0.119373226213588,-0.0916835585017708,
-1.76450211774327));
#46619=CARTESIAN_POINT('Ctrl Pts',(0.012454344419212,-0.150002437784443,
-1.75655482643532));
#46620=CARTESIAN_POINT('Ctrl Pts',(0.132858976296346,-0.0707413206950133,
-1.74860753512737));
#46621=CARTESIAN_POINT('Ctrl Pts',(0.131407338723251,0.073402679555044,
-1.74066024381942));
#46622=CARTESIAN_POINT('Ctrl Pts',(0.00943085200875732,0.150222838032626,
-1.73271295251147));
#46623=CARTESIAN_POINT('Ctrl Pts',(-0.121195471363827,0.0892608523210916,
-1.72476566120351));
#46624=CARTESIAN_POINT('Ctrl Pts',(-0.14066311787203,-0.0535698544585239,
-1.71681836989557));
#46625=CARTESIAN_POINT('Ctrl Pts',(-0.0311166527940441,-0.14726709053649,
-1.70887107858761));
#46626=CARTESIAN_POINT('Ctrl Pts',(0.106969541649328,-0.105893149898945,
-1.70092378727966));
#46627=CARTESIAN_POINT('Ctrl Pts',(0.146944869566731,0.0326044068218462,
-1.69297649597171));
#46628=CARTESIAN_POINT('Ctrl Pts',(0.0521445570312648,0.141197688395388,
-1.68502920466376));
#46629=CARTESIAN_POINT('Ctrl Pts',(-0.0904819646855179,0.120286558279953,
-1.67708191335581));
#46630=CARTESIAN_POINT('Ctrl Pts',(-0.150119779305,-0.0109496071895714,
-1.66913462204785));
#46631=CARTESIAN_POINT('Ctrl Pts',(-0.0720699736616587,-0.132142956424456,
-1.6611873307399));
#46632=CARTESIAN_POINT('Ctrl Pts',(0.0720813358062882,-0.132136758945303,
-1.65324003943195));
#46633=CARTESIAN_POINT('Ctrl Pts',(0.150120720260215,-0.0109366989874593,
-1.645292748124));
#46634=CARTESIAN_POINT('Ctrl Pts',(0.0904716214212405,0.120294337994768,
-1.63734545681605));
#46635=CARTESIAN_POINT('Ctrl Pts',(-0.0521566978274638,0.141193204184629,
-1.6293981655081));
#46636=CARTESIAN_POINT('Ctrl Pts',(-0.146947672537843,0.0325917715366741,
-1.62145087420015));
#46637=CARTESIAN_POINT('Ctrl Pts',(-0.106960435952101,-0.105902347363619,
-1.61350358289219));
#46638=CARTESIAN_POINT('Ctrl Pts',(0.031129315550067,-0.147264414403387,
-1.60555629158424));
#46639=CARTESIAN_POINT('Ctrl Pts',(0.140667723596079,-0.0535577592369685,
-1.59760900027629));
#46640=CARTESIAN_POINT('Ctrl Pts',(0.12118779575457,0.0892712730744692,
-1.58966170896834));
#46641=CARTESIAN_POINT('Ctrl Pts',(-0.0094437689971061,0.150222026558415,
-1.58171441766039));
#46642=CARTESIAN_POINT('Ctrl Pts',(-0.131413649821834,0.0733913801252743,
-1.57376712635244));
#46643=CARTESIAN_POINT('Ctrl Pts',(-0.132852893059766,-0.0707527444120611,
-1.56581983504448));
#46644=CARTESIAN_POINT('Ctrl Pts',(-0.0124414463012357,-0.150003508126047,
-1.55787254373653));
#46645=CARTESIAN_POINT('Ctrl Pts',(0.119381109251721,-0.0916732937665955,
-1.54992525242858));
#46646=CARTESIAN_POINT('Ctrl Pts',(0.141709093780764,0.0507382969365613,
-1.54197796112063));
#46647=CARTESIAN_POINT('Ctrl Pts',(0.0340636132367385,0.146613479221543,
-1.53403066981268));
#46648=CARTESIAN_POINT('Ctrl Pts',(-0.104824504792056,0.108016967330545,
-1.52608337850473));
#46649=CARTESIAN_POINT('Ctrl Pts',(-0.147569152074577,-0.0296510942829791,
-1.51813608719677));
#46650=CARTESIAN_POINT('Ctrl Pts',(-0.0549655763086878,-0.140123614916407,
-1.51018879588882));
#46651=CARTESIAN_POINT('Ctrl Pts',(0.0880516054014386,-0.122076848019669,
-1.50224150458087));
#46652=CARTESIAN_POINT('Ctrl Pts',(0.150309169263914,0.00793698125107607,
-1.49429421327292));
#46653=CARTESIAN_POINT('Ctrl Pts',(0.0747054072208741,0.130671129818913,
-1.48634692196497));
#46654=CARTESIAN_POINT('Ctrl Pts',(-0.0694170389597775,0.133555669060675,
-1.47839963065702));
#46655=CARTESIAN_POINT('Ctrl Pts',(-0.149871213415591,0.0139449426505173,
-1.47045233934906));
#46656=CARTESIAN_POINT('Ctrl Pts',(-0.0928657485312122,-0.118455876958156,
-1.46250504804111));
#46657=CARTESIAN_POINT('Ctrl Pts',(0.0493147944034109,-0.142210734788684,
-1.45455775673316));
#46658=CARTESIAN_POINT('Ctrl Pts',(0.14626454419011,-0.0355320299032718,
-1.44661046542521));
#46659=CARTESIAN_POINT('Ctrl Pts',(0.109062637801998,0.103736122309724,
-1.43866317411726));
#46660=CARTESIAN_POINT('Ctrl Pts',(-0.0281698916530059,0.147859051939493,
-1.43071588280931));
#46661=CARTESIAN_POINT('Ctrl Pts',(-0.139565417065501,0.0563678666930081,
-1.42276859150136));
#46662=CARTESIAN_POINT('Ctrl Pts',(-0.122953625682683,-0.0868230843017613,
-1.4148213001934));
#46663=CARTESIAN_POINT('Ctrl Pts',(0.00642939545620693,-0.150381198659458,
-1.40687400888545));
#46664=CARTESIAN_POINT('Ctrl Pts',(0.129915471074711,-0.0760119228254608,
-1.3989267175775));
#46665=CARTESIAN_POINT('Ctrl Pts',(0.1342450162852,0.0680743537521607,-1.39097942626955));
#46666=CARTESIAN_POINT('Ctrl Pts',(0.0154470368615123,0.149723849430834,
-1.38303213496159));
#46667=CARTESIAN_POINT('Ctrl Pts',(-0.117518734144473,0.0940488658159606,
-1.37508484365365));
#46668=CARTESIAN_POINT('Ctrl Pts',(-0.14269807676931,-0.0478863333585683,
-1.36713755234569));
#46669=CARTESIAN_POINT('Ctrl Pts',(-0.0369968738896843,-0.145900902528321,
-1.35919026103774));
#46670=CARTESIAN_POINT('Ctrl Pts',(0.102637309351477,-0.110097342226219,
-1.35124296972979));
#46671=CARTESIAN_POINT('Ctrl Pts',(0.148134084849236,0.0266858565923466,
-1.34329567842184));
#46672=CARTESIAN_POINT('Ctrl Pts',(0.0577644893922145,0.138993186169123,
-1.33534838711389));
#46673=CARTESIAN_POINT('Ctrl Pts',(-0.0855858333009689,0.123818040585234,
-1.32740109580594));
#46674=CARTESIAN_POINT('Ctrl Pts',(-0.150438107502626,-0.00492116319747254,
-1.31945380449798));
#46675=CARTESIAN_POINT('Ctrl Pts',(-0.0773107955712941,-0.129146749569324,
-1.31150651319003));
#46676=CARTESIAN_POINT('Ctrl Pts',(0.0667248237937332,-0.134920865420747,
-1.30355922188208));
#46677=CARTESIAN_POINT('Ctrl Pts',(0.149561430988952,-0.0169475779014209,
-1.29561193057413));
#46678=CARTESIAN_POINT('Ctrl Pts',(0.0952225266605833,0.116569775038653,
-1.28766463926618));
#46679=CARTESIAN_POINT('Ctrl Pts',(-0.0464530574311598,0.143171070721307,
-1.27971734795822));
#46680=CARTESIAN_POINT('Ctrl Pts',(-0.145522590799675,0.0384579979086082,
-1.27177005665028));
#46681=CARTESIAN_POINT('Ctrl Pts',(-0.111120976565583,-0.101528176400933,
-1.26382276534232));
#46682=CARTESIAN_POINT('Ctrl Pts',(0.0251991383179859,-0.148394223149754,
-1.25587547403437));
#46683=CARTESIAN_POINT('Ctrl Pts',(0.138406979764036,-0.0591553039784738,
-1.24792818272642));
#46684=CARTESIAN_POINT('Ctrl Pts',(0.124670005811998,0.0843399768023711,
-1.23998089141847));
#46685=CARTESIAN_POINT('Ctrl Pts',(-0.00341243612485143,0.150479890071337,
-1.23203360011052));
#46686=CARTESIAN_POINT('Ctrl Pts',(-0.12836504259628,0.0786018948591122,
-1.22408630880257));
#46687=CARTESIAN_POINT('Ctrl Pts',(-0.13558314851193,-0.0653685847772444,
-1.21613901749461));
#46688=CARTESIAN_POINT('Ctrl Pts',(-0.018446414893607,-0.149383974420822,
-1.20819172618666));
#46689=CARTESIAN_POINT('Ctrl Pts',(0.11560909505679,-0.096386613055642,
-1.20024443487871));
#46690=CARTESIAN_POINT('Ctrl Pts',(0.143629669086001,0.0450151107344386,
-1.19229714357076));
#46691=CARTESIAN_POINT('Ctrl Pts',(0.0399152550467209,0.145129647042715,
-1.18434985226281));
#46692=CARTESIAN_POINT('Ctrl Pts',(-0.100408834979363,0.112133437895548,
-1.17640256095486));
#46693=CARTESIAN_POINT('Ctrl Pts',(-0.14863944068462,-0.0237098863167076,
-1.1684552696469));
#46694=CARTESIAN_POINT('Ctrl Pts',(-0.0605401706079386,-0.137806856792214,
-1.16050797833895));
#46695=CARTESIAN_POINT('Ctrl Pts',(0.0830856400745417,-0.125509435699439,
-1.152560687031));
#46696=CARTESIAN_POINT('Ctrl Pts',(0.150506542164431,0.00190336593806516,
-1.14461339572305));
#46697=CARTESIAN_POINT('Ctrl Pts',(0.0798850908712658,0.127570428754776,
-1.1366661044151));
#46698=CARTESIAN_POINT('Ctrl Pts',(-0.064005773070029,0.136231798967407,
-1.12871881310715));
#46699=CARTESIAN_POINT('Ctrl Pts',(-0.149191497569375,0.0199433971327684,
-1.12077152179919));
#46700=CARTESIAN_POINT('Ctrl Pts',(-0.0975410079543931,-0.114636790793483,
-1.11282423049124));
#46701=CARTESIAN_POINT('Ctrl Pts',(0.0435726378512938,-0.144073825752174,
-1.10487693918329));
#46702=CARTESIAN_POINT('Ctrl Pts',(0.144722110767215,-0.0413684987795025,
-1.09692964787534));
#46703=CARTESIAN_POINT('Ctrl Pts',(0.113134624414992,0.099279397634488,
-1.08898235656739));
#46704=CARTESIAN_POINT('Ctrl Pts',(-0.0222182503300599,0.148869712797663,
-1.08103506525944));
#46705=CARTESIAN_POINT('Ctrl Pts',(-0.137192877594915,0.0619189500348204,
-1.07308777395148));
#46706=CARTESIAN_POINT('Ctrl Pts',(-0.126336245844431,-0.0818229492387265,
-1.06514048264353));
#46707=CARTESIAN_POINT('Ctrl Pts',(0.000394104371340178,-0.150518061102089,
-1.05719319133558));
#46708=CARTESIAN_POINT('Ctrl Pts',(0.12676298794177,-0.0811602545847577,
-1.04924590002763));
#46709=CARTESIAN_POINT('Ctrl Pts',(0.136866751566568,0.0626365257002925,
-1.04129860871968));
#46710=CARTESIAN_POINT('Ctrl Pts',(0.0214383741001049,0.1489840197878,-1.03335131741173));
#46711=CARTESIAN_POINT('Ctrl Pts',(-0.113652960012132,0.0986855952845626,
-1.02540402610377));
#46712=CARTESIAN_POINT('Ctrl Pts',(-0.144503496060692,-0.0421257838197151,
-1.01745673479582));
#46713=CARTESIAN_POINT('Ctrl Pts',(-0.0428175829859707,-0.144300022950198,
-1.00950944348787));
#46714=CARTESIAN_POINT('Ctrl Pts',(0.0981399779291522,-0.114124435456451,
-1.00156215217992));
#46715=CARTESIAN_POINT('Ctrl Pts',(0.149085016335446,0.0207243803392913,
-0.993614860871969));
#46716=CARTESIAN_POINT('Ctrl Pts',(0.06329150362539,0.136565103906617,-0.985667569564016));
#46717=CARTESIAN_POINT('Ctrl Pts',(-0.0805520312561653,0.127150353112736,
-0.977720278256066));
#46718=CARTESIAN_POINT('Ctrl Pts',(-0.150514445726104,0.00111519682184853,
-0.969772986948113));
#46719=CARTESIAN_POINT('Ctrl Pts',(-0.0824272577842244,-0.125942801343947,
-0.961825695640163));
#46720=CARTESIAN_POINT('Ctrl Pts',(0.0612609803433331,-0.1374879424661,
-0.953878404332209));
#46721=CARTESIAN_POINT('Ctrl Pts',(0.14876156193761,-0.0229311954784377,
-0.94593111302426));
#46722=CARTESIAN_POINT('Ctrl Pts',(0.0998202599599995,0.112657701635114,
-0.937983821716306));
#46723=CARTESIAN_POINT('Ctrl Pts',(-0.0406746941182161,0.144918636808996,
-0.930036530408357));
#46724=CARTESIAN_POINT('Ctrl Pts',(-0.143863426031812,0.044262361963377,
-0.922089239100402));
#46725=CARTESIAN_POINT('Ctrl Pts',(-0.115102771496254,-0.0969906904299014,
-0.914141947792454));
#46726=CARTESIAN_POINT('Ctrl Pts',(0.0192284265502686,-0.149285329649597,
-0.906194656484499));
#46727=CARTESIAN_POINT('Ctrl Pts',(0.135923598848805,-0.0646576933719181,
-0.89824736517655));
#46728=CARTESIAN_POINT('Ctrl Pts',(0.127951675647373,0.0792730139153126,
-0.890300073868596));
#46729=CARTESIAN_POINT('Ctrl Pts',(0.00262438588405391,0.150495696399996,
-0.882352782560647));
#46730=CARTESIAN_POINT('Ctrl Pts',(-0.12510995142956,0.0836859730748307,
-0.874405491252693));
#46731=CARTESIAN_POINT('Ctrl Pts',(-0.1380953092064,-0.0598792753077094,
-0.866458199944743));
#46732=CARTESIAN_POINT('Ctrl Pts',(-0.0244217111673174,-0.148524146386532,
-0.858510908636791));
#46733=CARTESIAN_POINT('Ctrl Pts',(0.111651115733821,-0.100944887892259,
-0.850563617328839));
#46734=CARTESIAN_POINT('Ctrl Pts',(0.145319206255449,0.0392195146511816,
-0.842616326020887));
#46735=CARTESIAN_POINT('Ctrl Pts',(0.0457026904418683,0.143412363911075,
-0.834669034712937));
#46736=CARTESIAN_POINT('Ctrl Pts',(-0.095831650695478,0.116069534164516,
-0.826721743404984));
#46737=CARTESIAN_POINT('Ctrl Pts',(-0.149470632598979,-0.0177305393783937,
-0.818774452097033));
#46738=CARTESIAN_POINT('Ctrl Pts',(-0.0660173819065402,-0.135268426923631,
-0.810827160789081));
#46739=CARTESIAN_POINT('Ctrl Pts',(0.0779860258190115,-0.128740132876833,
-0.802879869481131));
#46740=CARTESIAN_POINT('Ctrl Pts',(0.150461815008973,-0.00413331106909414,
-0.794932578173178));
#46741=CARTESIAN_POINT('Ctrl Pts',(0.0849362738950762,0.124264521940127,
-0.786985286865226));
#46742=CARTESIAN_POINT('Ctrl Pts',(-0.0584915495213012,0.138688790717869,
-0.779037995557275));
#46743=CARTESIAN_POINT('Ctrl Pts',(-0.148271797006258,0.0259097712981566,
-0.771090704249323));
#46744=CARTESIAN_POINT('Ctrl Pts',(-0.102059366002084,-0.110633303518608,
-0.763143412941372));
#46745=CARTESIAN_POINT('Ctrl Pts',(0.0377603917342272,-0.145705164123532,
-0.75519612163342));
#46746=CARTESIAN_POINT('Ctrl Pts',(0.14294688194145,-0.0471384235990644,
-0.747248830325468));
#46747=CARTESIAN_POINT('Ctrl Pts',(0.11702462625503,0.0946629752651919,
-0.739301539017517));
#46748=CARTESIAN_POINT('Ctrl Pts',(-0.0162308694334636,0.149640906551725,
-0.731354247709565));
#46749=CARTESIAN_POINT('Ctrl Pts',(-0.134599654007431,0.0673704325150745,
-0.723406956401614));
#46750=CARTESIAN_POINT('Ctrl Pts',(-0.129515645523193,-0.0766911963715416,
-0.715459665093661));
#46751=CARTESIAN_POINT('Ctrl Pts',(-0.00564182065732522,-0.150412804959745,
-0.707512373785711));
#46752=CARTESIAN_POINT('Ctrl Pts',(0.123406597882029,-0.0861780345295194,
-0.699565082477759));
#46753=CARTESIAN_POINT('Ctrl Pts',(0.139268327327031,0.0570979425173868,
-0.691617791169807));
#46754=CARTESIAN_POINT('Ctrl Pts',(0.0273952262492426,0.148004539170056,
-0.683670499861856));
#46755=CARTESIAN_POINT('Ctrl Pts',(-0.10960436732862,0.10316358223075,-0.675723208553903));
#46756=CARTESIAN_POINT('Ctrl Pts',(-0.146076471605894,-0.0362974720794752,
-0.667775917245953));
#46757=CARTESIAN_POINT('Ctrl Pts',(-0.0485694170746423,-0.142467026926293,
-0.659828625938001));
#46758=CARTESIAN_POINT('Ctrl Pts',(0.0934847816472068,-0.117967951735047,
-0.651881334630049));
#46759=CARTESIAN_POINT('Ctrl Pts',(0.149796134387099,0.0147295675045261,
-0.643934043322098));
#46760=CARTESIAN_POINT('Ctrl Pts',(0.0687167091507831,0.133917347344078,
-0.635986752014146));
#46761=CARTESIAN_POINT('Ctrl Pts',(-0.0753886557656117,0.130278135610093,
-0.628039460706194));
#46762=CARTESIAN_POINT('Ctrl Pts',(-0.150348671180187,0.00714976297088918,
-0.620092169398244));
#46763=CARTESIAN_POINT('Ctrl Pts',(-0.0874111301214144,-0.122536265517948,
-0.61214487809029));
#46764=CARTESIAN_POINT('Ctrl Pts',(0.0556985944205823,-0.139833860762547,
-0.60419758678234));
#46765=CARTESIAN_POINT('Ctrl Pts',(0.147722399750208,-0.0288779266608177,
-0.596250295474387));
#46766=CARTESIAN_POINT('Ctrl Pts',(0.104257425551351,0.108564410621494,
-0.588303004166437));
#46767=CARTESIAN_POINT('Ctrl Pts',(-0.0348309027808034,0.146433091368251,
-0.580355712858484));
#46768=CARTESIAN_POINT('Ctrl Pts',(-0.141972847114145,0.0499955269848398,
-0.572408421550534));
#46769=CARTESIAN_POINT('Ctrl Pts',(-0.118899415754923,-0.0922971883067176,
-0.564461130242581));
#46770=CARTESIAN_POINT('Ctrl Pts',(0.0132267845447208,-0.149936300497229,
-0.55651383893463));
#46771=CARTESIAN_POINT('Ctrl Pts',(0.133221575538256,-0.0700560764480323,
-0.548566547626678));
#46772=CARTESIAN_POINT('Ctrl Pts',(0.131027526470557,0.0740785349692836,
-0.540619256318727));
#46773=CARTESIAN_POINT('Ctrl Pts',(0.00865698638896329,0.150269420118829,
-0.532671965010775));
#46774=CARTESIAN_POINT('Ctrl Pts',(-0.121653612358199,0.0886354366852716,
-0.524724673702824));
#46775=CARTESIAN_POINT('Ctrl Pts',(-0.140385334161072,-0.0542936459327594,
-0.516777382394872));
#46776=CARTESIAN_POINT('Ctrl Pts',(-0.0303577234500885,-0.147425407115313,
-0.50883009108692));
#46777=CARTESIAN_POINT('Ctrl Pts',(0.107513537962964,-0.105340785979954,
-0.500882799778969));
#46778=CARTESIAN_POINT('Ctrl Pts',(0.146774987553141,0.0333608312990502,
-0.492935508471017));
#46779=CARTESIAN_POINT('Ctrl Pts',(0.0514166099369417,0.141464392193867,
-0.484988217163065));
#46780=CARTESIAN_POINT('Ctrl Pts',(-0.091100314654041,0.119818924657679,
-0.477040925855113));
#46781=CARTESIAN_POINT('Ctrl Pts',(-0.150061390788673,-0.0117226716561039,
-0.469093634547163));
#46782=CARTESIAN_POINT('Ctrl Pts',(-0.0713883997359057,-0.132512408548537,
-0.46114634323921));
#46783=CARTESIAN_POINT('Ctrl Pts',(0.0727609657127887,-0.131763742754713,
-0.45319905193126));
#46784=CARTESIAN_POINT('Ctrl Pts',(0.15017505974422,-0.0101633393630106,
-0.445251760623307));
#46785=CARTESIAN_POINT('Ctrl Pts',(0.0898508311193224,0.120758727151932,
-0.437304469315356));
#46786=CARTESIAN_POINT('Ctrl Pts',(-0.0528832383189022,0.140922692072975,
-0.429357178007404));
#46787=CARTESIAN_POINT('Ctrl Pts',(-0.147113591127436,0.0318344678262087,
-0.421409886699453));
#46788=CARTESIAN_POINT('Ctrl Pts',(-0.106413554586663,-0.106451855016336,
-0.413462595391501));
#46789=CARTESIAN_POINT('Ctrl Pts',(0.0318874054471912,-0.147102125783533,
-0.405515304083549));
#46790=CARTESIAN_POINT('Ctrl Pts',(0.140941713289669,-0.0528325230436766,
-0.397568012775598));
#46791=CARTESIAN_POINT('Ctrl Pts',(0.120726385988382,0.0898942810326212,
-0.389620721467646));
#46792=CARTESIAN_POINT('Ctrl Pts',(-0.0102173800744564,0.150171392683833,
-0.381673430159694));
#46793=CARTESIAN_POINT('Ctrl Pts',(-0.131789917680354,0.0727135450517523,
-0.373726138851743));
#46794=CARTESIAN_POINT('Ctrl Pts',(-0.132486710437372,-0.0714360804752875,
-0.365778847543792));
#46795=CARTESIAN_POINT('Ctrl Pts',(-0.0116686704320159,-0.150065599544122,
-0.35783155623584));
#46796=CARTESIAN_POINT('Ctrl Pts',(0.119851699878208,-0.0910571912178954,
-0.349884264927888));
#46797=CARTESIAN_POINT('Ctrl Pts',(0.141445880467903,0.0514675133928953,
-0.341936973619936));
#46798=CARTESIAN_POINT('Ctrl Pts',(0.0333080113052628,0.146786983139092,
-0.333989682311985));
#46799=CARTESIAN_POINT('Ctrl Pts',(-0.105379468531873,0.107475623506582,
-0.326042391004033));
#46800=CARTESIAN_POINT('Ctrl Pts',(-0.14741447316628,-0.0304107733754844,
-0.318095099696082));
#46801=CARTESIAN_POINT('Ctrl Pts',(-0.0542431239375945,-0.140404862955942,
-0.31014780838813));
#46802=CARTESIAN_POINT('Ctrl Pts',(0.088679208706928,-0.121621708503485,
-0.302200517080178));
#46803=CARTESIAN_POINT('Ctrl Pts',(0.150266295122196,0.00871106115410149,
-0.294253225772228));
#46804=CARTESIAN_POINT('Ctrl Pts',(0.0740313791546959,0.131054175578779,
-0.286305934464275));
#46805=CARTESIAN_POINT('Ctrl Pts',(-0.0701040124716336,0.133196356825569,
-0.278358643156324));
#46806=CARTESIAN_POINT('Ctrl Pts',(-0.149941050524403,0.0131728282375115,
-0.270411351848372));
#46807=CARTESIAN_POINT('Ctrl Pts',(-0.092254395683996,-0.11893262173657,
-0.26246406054042));
#46808=CARTESIAN_POINT('Ctrl Pts',(0.0500466135038247,-0.141954846740938,
-0.254516769232468));
#46809=CARTESIAN_POINT('Ctrl Pts',(0.146445615989062,-0.0347782057238245,
-0.246569477924518));
#46810=CARTESIAN_POINT('Ctrl Pts',(0.108526885952636,0.104296486333508,
-0.238622186616565));
#46811=CARTESIAN_POINT('Ctrl Pts',(-0.0289310835603638,0.147711998300275,
-0.230674895308614));
#46812=CARTESIAN_POINT('Ctrl Pts',(-0.139853895164789,0.0556482707761755,
-0.222727604000662));
#46813=CARTESIAN_POINT('Ctrl Pts',(-0.122504802193644,-0.0874552198327828,
-0.214780312692711));
#46814=CARTESIAN_POINT('Ctrl Pts',(0.00720386637860762,-0.150346088594642,
-0.206833021384759));
#46815=CARTESIAN_POINT('Ctrl Pts',(0.13030525617202,-0.075341769476037,
-0.198885730076808));
#46816=CARTESIAN_POINT('Ctrl Pts',(0.133892610659253,0.0687648955194049,
-0.190938438768856));
#46817=CARTESIAN_POINT('Ctrl Pts',(0.014675661361578,0.149801425434866,
-0.182991147460905));
#46818=CARTESIAN_POINT('Ctrl Pts',(-0.11800158480147,0.0934423237107693,
-0.175043856152952));
#46819=CARTESIAN_POINT('Ctrl Pts',(-0.142449540356412,-0.0486206807040808,
-0.167096564845001));
#46820=CARTESIAN_POINT('Ctrl Pts',(-0.0362449020418857,-0.146089525550903,
-0.159149273537049));
#46821=CARTESIAN_POINT('Ctrl Pts',(0.103203015007595,-0.109567233280859,
-0.151201982229098));
#46822=CARTESIAN_POINT('Ctrl Pts',(0.147994675645917,0.027448479198832,
-0.143254690921146));
#46823=CARTESIAN_POINT('Ctrl Pts',(0.0570478139685668,0.139288875912043,
-0.135307399613195));
#46824=CARTESIAN_POINT('Ctrl Pts',(-0.0862224217148439,0.123375558151578,
-0.127360108305243));
#46825=CARTESIAN_POINT('Ctrl Pts',(-0.150410795001361,-0.00569590911631693,
-0.119412816997291));
#46826=CARTESIAN_POINT('Ctrl Pts',(-0.0766445274621928,-0.12954330722548,
-0.11146552568934));
#46827=CARTESIAN_POINT('Ctrl Pts',(0.0674187564615154,-0.134575264392198,
-0.103518234381388));
#46828=CARTESIAN_POINT('Ctrl Pts',(0.149646942931058,-0.0161772797550832,
-0.0955709430734365));
#46829=CARTESIAN_POINT('Ctrl Pts',(0.0946204674793121,0.117059178191346,
-0.0876236517654852));
#46830=CARTESIAN_POINT('Ctrl Pts',(-0.0471891212084412,0.142928971075017,
-0.0796763604575334));
#46831=CARTESIAN_POINT('Ctrl Pts',(-0.145720146807228,0.0377097379155704,
-0.0717290691495822));
#46832=CARTESIAN_POINT('Ctrl Pts',(-0.110593905137976,-0.10210255282505,
-0.0637817778416302));
#46833=CARTESIAN_POINT('Ctrl Pts',(0.0259580684157336,-0.148256045218673,
-0.0558344865336788));
#46834=CARTESIAN_POINT('Ctrl Pts',(0.138719431502144,-0.0584538229284914,
-0.047887195225727));
#46835=CARTESIAN_POINT('Ctrl Pts',(0.124215712985446,0.0850041361652265,
-0.0399399039177754));
#46836=CARTESIAN_POINT('Ctrl Pts',(-0.004152737614071,0.150416188445784,
-0.0319926126098237));
#46837=CARTESIAN_POINT('Ctrl Pts',(-0.128834969429613,0.0780250473313025,
-0.0240453213018721));
#46838=CARTESIAN_POINT('Ctrl Pts',(-0.135110406641513,-0.0662414518576971,
-0.0160980299939207));
#46839=CARTESIAN_POINT('Ctrl Pts',(-0.0570343146549906,-0.121442316265599,
-0.0107998357886196));
#46840=CARTESIAN_POINT('Ctrl Pts',(-0.0149499840092685,-0.126419096572166,
-0.00815073868596909));
#46841=CARTESIAN_POINT('Ctrl Pts',(0.120439183586217,-0.0649267562880324,
-2.94314926131403));
#46842=CARTESIAN_POINT('Ctrl Pts',(0.14205299948483,-0.024833110927659,
-2.94050016421138));
#46843=CARTESIAN_POINT('Ctrl Pts',(0.141715520135631,0.0779399629980596,
-2.93520197000608));
#46844=CARTESIAN_POINT('Ctrl Pts',(0.0109341606128859,0.161520108869991,
-2.92725467869813));
#46845=CARTESIAN_POINT('Ctrl Pts',(-0.129750457406967,0.0965515110554682,
-2.91930738739018));
#46846=CARTESIAN_POINT('Ctrl Pts',(-0.151491649088109,-0.0567683102589726,
-2.91136009608222));
#46847=CARTESIAN_POINT('Ctrl Pts',(-0.0342549406055127,-0.158127703177675,
-2.90341280477428));
#46848=CARTESIAN_POINT('Ctrl Pts',(0.114383078266682,-0.114398680790832,
-2.89546551346632));
#46849=CARTESIAN_POINT('Ctrl Pts',(0.15811949456322,0.0342255899845588,
-2.88751822215837));
#46850=CARTESIAN_POINT('Ctrl Pts',(0.0568264098997039,0.151474208223123,
-2.87957093085042));
#46851=CARTESIAN_POINT('Ctrl Pts',(-0.0965845537755583,0.129784753121562,
-2.87162363954247));
#46852=CARTESIAN_POINT('Ctrl Pts',(-0.161410900544422,-0.0109370243537351,
-2.86367634823452));
#46853=CARTESIAN_POINT('Ctrl Pts',(-0.0781928975915483,-0.141629800004137,
-2.85572905692656));
#46854=CARTESIAN_POINT('Ctrl Pts',(0.0767421044758823,-0.14242063978591,
-2.84778176561862));
#46855=CARTESIAN_POINT('Ctrl Pts',(0.161290583296262,-0.0125860262202751,
-2.83983447431066));
#46856=CARTESIAN_POINT('Ctrl Pts',(0.0979056475321585,0.128792635178867,
-2.83188718300271));
#46857=CARTESIAN_POINT('Ctrl Pts',(-0.0552768338809414,0.152044439313014,
-2.82393989169476));
#46858=CARTESIAN_POINT('Ctrl Pts',(-0.157760256221094,0.0358434460527866,
-2.81599260038681));
#46859=CARTESIAN_POINT('Ctrl Pts',(-0.115548312366974,-0.113232669402329,
-2.80804530907885));
#46860=CARTESIAN_POINT('Ctrl Pts',(0.0326428107524121,-0.158453445448113,
-2.80009801777091));
#46861=CARTESIAN_POINT('Ctrl Pts',(0.15089443925921,-0.05834310056466,-2.79215072646295));
#46862=CARTESIAN_POINT('Ctrl Pts',(0.130747938827138,0.095278672194432,
-2.784203435155));
#46863=CARTESIAN_POINT('Ctrl Pts',(-0.00931861788340384,0.161512265598379,
-2.77625614384705));
#46864=CARTESIAN_POINT('Ctrl Pts',(-0.140838277991704,0.0796092223769108,
-2.7683088525391));
#46865=CARTESIAN_POINT('Ctrl Pts',(-0.14318317195546,-0.0753102120683318,
-2.76036156123115));
#46866=CARTESIAN_POINT('Ctrl Pts',(-0.0142025985168282,-0.161156243851845,
-2.75241426992319));
#46867=CARTESIAN_POINT('Ctrl Pts',(0.127804386320586,-0.0991921751552476,
-2.74446697861524));
#46868=CARTESIAN_POINT('Ctrl Pts',(0.152591096121994,0.0537494757885291,
-2.73651968730729));
#46869=CARTESIAN_POINT('Ctrl Pts',(0.0374235307972619,0.157392909948435,
-2.72857239599934));
#46870=CARTESIAN_POINT('Ctrl Pts',(-0.112068338247225,0.116677917050738,
-2.72062510469139));
#46871=CARTESIAN_POINT('Ctrl Pts',(-0.158772800645446,-0.0310523193655248,
-2.71267781338343));
#46872=CARTESIAN_POINT('Ctrl Pts',(-0.0598532208020871,-0.150301832064811,
-2.70473052207548));
#46873=CARTESIAN_POINT('Ctrl Pts',(0.0939628395432803,-0.131696748434227,
-2.69678323076753));
#46874=CARTESIAN_POINT('Ctrl Pts',(0.16159758634093,0.00769862660697697,
-2.68883593945958));
#46875=CARTESIAN_POINT('Ctrl Pts',(0.0810174396286684,0.140032936264449,
-2.68088864815163));
#46876=CARTESIAN_POINT('Ctrl Pts',(-0.0738706931061093,0.143931127498383,
-2.67294135684368));
#46877=CARTESIAN_POINT('Ctrl Pts',(-0.161005729026759,0.0158178375083437,
-2.66499406553573));
#46878=CARTESIAN_POINT('Ctrl Pts',(-0.10046871412908,-0.126803336880895,
-2.65704677422778));
#46879=CARTESIAN_POINT('Ctrl Pts',(0.0522167053515813,-0.153122383880087,
-2.64909948291982));
#46880=CARTESIAN_POINT('Ctrl Pts',(0.157009742288698,-0.0389998665295485,
-2.64115219161187));
#46881=CARTESIAN_POINT('Ctrl Pts',(0.117795787782758,0.110892746126725,
-2.63320490030392));
#46882=CARTESIAN_POINT('Ctrl Pts',(-0.0294587045649093,0.159076187684537,
-2.62525760899597));
#46883=CARTESIAN_POINT('Ctrl Pts',(-0.149694112909478,0.061357324934615,
-2.61731031768802));
#46884=CARTESIAN_POINT('Ctrl Pts',(-0.132632315853919,-0.0926375601692635,
-2.60936302638006));
#46885=CARTESIAN_POINT('Ctrl Pts',(0.00607786107815708,-0.161666658181589,
-2.60141573507212));
#46886=CARTESIAN_POINT('Ctrl Pts',(0.139213514572923,-0.0824175110224898,
-2.59346844376416));
#46887=CARTESIAN_POINT('Ctrl Pts',(0.144664610984601,0.0724237467379446,
-2.58552115245621));
#46888=CARTESIAN_POINT('Ctrl Pts',(0.0174314860702634,0.160839025290102,
-2.57757386114826));
#46889=CARTESIAN_POINT('Ctrl Pts',(-0.125789537612448,0.101735151202198,
-2.56962656984031));
#46890=CARTESIAN_POINT('Ctrl Pts',(-0.153638275457792,-0.0506786846439741,
-2.56167927853235));
#46891=CARTESIAN_POINT('Ctrl Pts',(-0.0405722809007601,-0.156610787576711,
-2.5537319872244));
#46892=CARTESIAN_POINT('Ctrl Pts',(0.109706003946886,-0.118901814371748,
-2.54578469591645));
#46893=CARTESIAN_POINT('Ctrl Pts',(0.159363579905122,0.0278621277491786,
-2.5378374046085));
#46894=CARTESIAN_POINT('Ctrl Pts',(0.0628552597017324,0.149071342285214,
-2.52989011330055));
#46895=CARTESIAN_POINT('Ctrl Pts',(-0.09130296625958,0.133554547339616,
-2.5219428219926));
#46896=CARTESIAN_POINT('Ctrl Pts',(-0.161719474737566,-0.0044564844320954,
-2.51399553068464));
#46897=CARTESIAN_POINT('Ctrl Pts',(-0.0838092954875492,-0.138380095218816,
-2.5060482393767));
#46898=CARTESIAN_POINT('Ctrl Pts',(0.0709695182955605,-0.145383548710932,
-2.49810094806874));
#46899=CARTESIAN_POINT('Ctrl Pts',(0.160656149485851,-0.0190433819283141,
-2.49015365676079));
#46900=CARTESIAN_POINT('Ctrl Pts',(0.102991358993371,0.124763090437783,
-2.48220636545284));
#46901=CARTESIAN_POINT('Ctrl Pts',(-0.0491355682880311,0.154138718990071,
-2.47425907414489));
#46902=CARTESIAN_POINT('Ctrl Pts',(-0.156196085938658,0.0421406158038896,
-2.46631178283693));
#46903=CARTESIAN_POINT('Ctrl Pts',(-0.119995885602437,-0.108508231030529,
-2.45836449152899));
#46904=CARTESIAN_POINT('Ctrl Pts',(0.0262627494478528,-0.159634948411453,
-2.45041720022103));
#46905=CARTESIAN_POINT('Ctrl Pts',(0.148433582812218,-0.0643468744883253,
-2.44246990891309));
#46906=CARTESIAN_POINT('Ctrl Pts',(0.134463350161716,0.0899591920049057,
-2.43452261760513));
#46907=CARTESIAN_POINT('Ctrl Pts',(-0.00283465969473679,0.161756030698404,
-2.42657532629718));
#46908=CARTESIAN_POINT('Ctrl Pts',(-0.137532762001164,0.0851926530824045,
-2.41862803498923));
#46909=CARTESIAN_POINT('Ctrl Pts',(-0.146087868389377,-0.069508153998907,
-2.41068074368127));
#46910=CARTESIAN_POINT('Ctrl Pts',(-0.020653363009408,-0.160457120001854,
-2.40273345237332));
#46911=CARTESIAN_POINT('Ctrl Pts',(0.123724098564309,-0.104237211193206,
-2.39478616106537));
#46912=CARTESIAN_POINT('Ctrl Pts',(0.154623664158228,0.0475875114412515,
-2.38683886975742));
#46913=CARTESIAN_POINT('Ctrl Pts',(0.0437047135457649,0.155765679072029,
-2.37889157844947));
#46914=CARTESIAN_POINT('Ctrl Pts',(-0.107299547811519,0.121077891467977,
-2.37094428714151));
#46915=CARTESIAN_POINT('Ctrl Pts',(-0.159890265917922,-0.0246607304754712,
-2.36299699583357));
#46916=CARTESIAN_POINT('Ctrl Pts',(-0.0658320193152775,-0.147780898616028,
-2.35504970452561));
#46917=CARTESIAN_POINT('Ctrl Pts',(0.0886063725192689,-0.135358632941768,
-2.34710241321766));
#46918=CARTESIAN_POINT('Ctrl Pts',(0.161776322388465,0.00121254993757108,
-2.33915512190971));
#46919=CARTESIAN_POINT('Ctrl Pts',(0.0865674447129999,0.136671600117762,
-2.33120783060176));
#46920=CARTESIAN_POINT('Ctrl Pts',(-0.0680398007854702,0.146777499201892,
-2.32326053929381));
#46921=CARTESIAN_POINT('Ctrl Pts',(-0.160241956850158,0.0222612674329143,
-2.31531324798586));
#46922=CARTESIAN_POINT('Ctrl Pts',(-0.105472582533561,-0.122672666460744,
-2.30736595667791));
#46923=CARTESIAN_POINT('Ctrl Pts',(0.0460346697578994,-0.155093062201921,
-2.29941866536995));
#46924=CARTESIAN_POINT('Ctrl Pts',(0.155319610253441,-0.0452644168592387,
-2.291471374062));
#46925=CARTESIAN_POINT('Ctrl Pts',(0.122147723174673,0.106080075820726,
-2.28352408275405));
#46926=CARTESIAN_POINT('Ctrl Pts',(-0.0230562319120901,0.160129506752827,
-2.2755767914461));
#46927=CARTESIAN_POINT('Ctrl Pts',(-0.147113355322838,0.0673105448540142,
-2.26762950013814));
#46928=CARTESIAN_POINT('Ctrl Pts',(-0.13624030566074,-0.0872446438261734,
-2.2596822088302));
#46929=CARTESIAN_POINT('Ctrl Pts',(-0.000409681739256192,-0.16178034776746,
-2.25173491752224));
#46930=CARTESIAN_POINT('Ctrl Pts',(0.135796696156851,-0.0879335321465694,
-2.2437876262143));
#46931=CARTESIAN_POINT('Ctrl Pts',(0.147452371807367,0.0665646062954607,
-2.23584033490634));
#46932=CARTESIAN_POINT('Ctrl Pts',(0.0238669335270067,0.160010681665022,
-2.22789304359839));
#46933=CARTESIAN_POINT('Ctrl Pts',(-0.121608899846648,0.106697348800126,
-2.21994575229043));
#46934=CARTESIAN_POINT('Ctrl Pts',(-0.155546865924041,-0.0444771993733432,
-2.21199846098249));
#46935=CARTESIAN_POINT('Ctrl Pts',(-0.0468195689190186,-0.154857924334291,
-2.20405116967453));
#46936=CARTESIAN_POINT('Ctrl Pts',(0.104849937673813,-0.123205273152918,
-2.19610387836658));
#46937=CARTESIAN_POINT('Ctrl Pts',(0.160352646860941,0.0214494150870821,
-2.18815658705863));
#46938=CARTESIAN_POINT('Ctrl Pts',(0.068782302441517,0.146431020052896,
-2.18020929575068));
#46939=CARTESIAN_POINT('Ctrl Pts',(-0.0858741428449303,0.137108279668065,
-2.17226200444273));
#46940=CARTESIAN_POINT('Ctrl Pts',(-0.161768106430643,0.00203187222333996,
-2.16431471313477));
#46941=CARTESIAN_POINT('Ctrl Pts',(-0.0892907780255418,-0.134908138088409,
-2.15636742182682));
#46942=CARTESIAN_POINT('Ctrl Pts',(0.065082718856964,-0.148112418348608,
-2.14842013051887));
#46943=CARTESIAN_POINT('Ctrl Pts',(0.15976331770074,-0.0254701998449192,
-2.14047283921092));
#46944=CARTESIAN_POINT('Ctrl Pts',(0.107911386844908,0.120532905681794,
-2.13252554790297));
#46945=CARTESIAN_POINT('Ctrl Pts',(-0.0429152568883603,0.155985029695461,
-2.12457825659502));
#46946=CARTESIAN_POINT('Ctrl Pts',(-0.154380667736248,0.048370013357431,
-2.11663096528707));
#46947=CARTESIAN_POINT('Ctrl Pts',(-0.124250435068012,-0.103609257058902,
-2.10868367397912));
#46948=CARTESIAN_POINT('Ctrl Pts',(0.0198404415629177,-0.160559663805939,
-2.10073638267116));
#46949=CARTESIAN_POINT('Ctrl Pts',(0.145733961413755,-0.0702471440952718,
-2.09278909136321));
#46950=CARTESIAN_POINT('Ctrl Pts',(0.137962467690555,0.0844950073768885,
-2.08484180005526));
#46951=CARTESIAN_POINT('Ctrl Pts',(0.00365385840641593,0.161739599608858,
-2.07689450874731));
#46952=CARTESIAN_POINT('Ctrl Pts',(-0.134006015255314,0.0906390458813432,
-2.06894721743935));
#46953=CARTESIAN_POINT('Ctrl Pts',(-0.148757572459151,-0.0635942874710312,
-2.0609999261314));
#46954=CARTESIAN_POINT('Ctrl Pts',(-0.0270709051811781,-0.159499889829302,
-2.05305263482345));
#46955=CARTESIAN_POINT('Ctrl Pts',(0.119444792155413,-0.109114574598621,
-2.0451053435155));
#46956=CARTESIAN_POINT('Ctrl Pts',(0.15640750945962,0.04134899935339,-2.03715805220755));
#46957=CARTESIAN_POINT('Ctrl Pts',(0.0499155942801435,0.153887888446583,
-2.0292107608996));
#46958=CARTESIAN_POINT('Ctrl Pts',(-0.102358158724142,0.125283103830848,
-2.02126346959164));
#46959=CARTESIAN_POINT('Ctrl Pts',(-0.160750536772648,-0.0182294731189203,
-2.0133161782837));
#46960=CARTESIAN_POINT('Ctrl Pts',(-0.0717049225281518,-0.145022249493378,
-2.00536888697574));
#46961=CARTESIAN_POINT('Ctrl Pts',(0.0831073760915768,-0.138802783841179,
-1.99742159566779));
#46962=CARTESIAN_POINT('Ctrl Pts',(0.161694830168414,-0.00527547720076154,
-1.98947430435984));
#46963=CARTESIAN_POINT('Ctrl Pts',(0.0919782001481242,0.133090418364356,
-1.98152701305189));
#46964=CARTESIAN_POINT('Ctrl Pts',(-0.0620994617966974,0.149387769269938,
-1.97357972174394));
#46965=CARTESIAN_POINT('Ctrl Pts',(-0.159220424537894,0.0286688885878118,
-1.96563243043599));
#46966=CARTESIAN_POINT('Ctrl Pts',(-0.110306791082952,-0.118344668675314,
-1.95768513912803));
#46967=CARTESIAN_POINT('Ctrl Pts',(0.03977858425274,-0.156814262736958,
-1.94973784782008));
#46968=CARTESIAN_POINT('Ctrl Pts',(0.153379636013345,-0.0514561562818434,
-1.94179055651213));
#46969=CARTESIAN_POINT('Ctrl Pts',(0.126303175608487,0.101096768465166,
-1.93384326520418));
#46970=CARTESIAN_POINT('Ctrl Pts',(-0.0166166717349957,0.160925246569142,
-1.92589597389623));
#46971=CARTESIAN_POINT('Ctrl Pts',(-0.144295955853084,0.0731554911632232,
-1.91794868258828));
#46972=CARTESIAN_POINT('Ctrl Pts',(-0.139629143627699,-0.0817113885127615,
-1.91000139128032));
#46973=CARTESIAN_POINT('Ctrl Pts',(-0.00689656555560029,-0.161633802610794,
-1.90205409997237));
#46974=CARTESIAN_POINT('Ctrl Pts',(0.132161439477111,-0.0933081061763968,
-1.89410680866442));
#46975=CARTESIAN_POINT('Ctrl Pts',(0.150002945415843,0.0605983921359247,
-1.88615951735647));
#46976=CARTESIAN_POINT('Ctrl Pts',(0.0302639893905353,0.158924949926238,
-1.87821222604852));
#46977=CARTESIAN_POINT('Ctrl Pts',(-0.117232645856884,0.111487916422733,
-1.87026493474057));
#46978=CARTESIAN_POINT('Ctrl Pts',(-0.157205248629181,-0.0382041694887514,
-1.86231764343261));
#46979=CARTESIAN_POINT('Ctrl Pts',(-0.0529915444618639,-0.152855961540379,
-1.85437035212466));
#46980=CARTESIAN_POINT('Ctrl Pts',(0.0998252131124366,-0.127310547834593,
-1.84642306081671));
#46981=CARTESIAN_POINT('Ctrl Pts',(0.161083775628675,0.0150021995753526,
-1.83847576950876));
#46982=CARTESIAN_POINT('Ctrl Pts',(0.0745987041484787,0.143555153520365,
-1.83052847820081));
#46983=CARTESIAN_POINT('Ctrl Pts',(-0.0803071850044249,0.140441463961156,
-1.82258118689286));
#46984=CARTESIAN_POINT('Ctrl Pts',(-0.161556523072208,0.0085169604734811,
-1.81463389558491));
#46985=CARTESIAN_POINT('Ctrl Pts',(-0.0946286302465571,-0.131219172000695,
-1.80668660427695));
#46986=CARTESIAN_POINT('Ctrl Pts',(0.0590912294185051,-0.150603039042038,
-1.798739312969));
#46987=CARTESIAN_POINT('Ctrl Pts',(0.158613495703762,-0.0318560472048982,
-1.79079202166105));
#46988=CARTESIAN_POINT('Ctrl Pts',(0.112657831857984,0.116108835511971,
-1.7828447303531));
#46989=CARTESIAN_POINT('Ctrl Pts',(-0.036625913365931,0.157580427823379,
-1.77489743904515));
#46990=CARTESIAN_POINT('Ctrl Pts',(-0.15231691768219,0.0545216044397509,
-1.76695014773719));
#46991=CARTESIAN_POINT('Ctrl Pts',(-0.128305119219744,-0.0985436205185058,
-1.75900285642925));
#46992=CARTESIAN_POINT('Ctrl Pts',(0.0133862189721914,-0.16122610801144,
-1.75105556512129));
#46993=CARTESIAN_POINT('Ctrl Pts',(0.142799916981525,-0.0760344163715165,
-1.74310827381334));
#46994=CARTESIAN_POINT('Ctrl Pts',(0.141239663164244,0.0788949067566377,
-1.73516098250539));
#46995=CARTESIAN_POINT('Ctrl Pts',(0.0101364990266846,0.161462999322971,
-1.72721369119744));
#46996=CARTESIAN_POINT('Ctrl Pts',(-0.13026371067837,0.0959396395823433,
-1.71926639988948));
#46997=CARTESIAN_POINT('Ctrl Pts',(-0.151187989810213,-0.0575781251868712,
-1.71131910858153));
#46998=CARTESIAN_POINT('Ctrl Pts',(-0.0334449019524261,-0.15828609318661,
-1.70337181727358));
#46999=CARTESIAN_POINT('Ctrl Pts',(0.11497335063763,-0.11381641975587,-1.69542452596563));
#47000=CARTESIAN_POINT('Ctrl Pts',(0.157939762595976,0.0350439745750224,
-1.68747723465768));
#47001=CARTESIAN_POINT('Ctrl Pts',(0.0560461823707901,0.151762558638644,
-1.67952994334973));
#47002=CARTESIAN_POINT('Ctrl Pts',(-0.097252119545145,0.129286789761617,
-1.67158265204178));
#47003=CARTESIAN_POINT('Ctrl Pts',(-0.161352229406179,-0.0117688924093824,
-1.66363536073382));
#47004=CARTESIAN_POINT('Ctrl Pts',(-0.0774624834741187,-0.142030322174209,
-1.65568806942587));
#47005=CARTESIAN_POINT('Ctrl Pts',(0.0774746957713786,-0.142023660979501,
-1.64774077811792));
#47006=CARTESIAN_POINT('Ctrl Pts',(0.161353240766724,-0.0117550183735887,
-1.63979348680997));
#47007=CARTESIAN_POINT('Ctrl Pts',(0.0972410023641809,0.129295151580007,
-1.63184619550202));
#47008=CARTESIAN_POINT('Ctrl Pts',(-0.0560592315808636,0.151757738904646,
-1.62389890419407));
#47009=CARTESIAN_POINT('Ctrl Pts',(-0.157942775294506,0.0350303938767022,
-1.61595161288612));
#47010=CARTESIAN_POINT('Ctrl Pts',(-0.114963563622508,-0.113826305404776,
-1.60800432157816));
#47011=CARTESIAN_POINT('Ctrl Pts',(0.0334585121770555,-0.158283216816521,
-1.60005703027021));
#47012=CARTESIAN_POINT('Ctrl Pts',(0.15119294014952,-0.0575651249614849,
-1.59210973896226));
#47013=CARTESIAN_POINT('Ctrl Pts',(0.130255460755053,0.0959508400503948,
-1.58416244765431));
#47014=CARTESIAN_POINT('Ctrl Pts',(-0.0101503825061297,0.161462127131619,
-1.57621515634636));
#47015=CARTESIAN_POINT('Ctrl Pts',(-0.141246446479757,0.0788827618667677,
-1.5682678650384));
#47016=CARTESIAN_POINT('Ctrl Pts',(-0.142793378577391,-0.0760466948482432,
-1.56032057373045));
#47017=CARTESIAN_POINT('Ctrl Pts',(-0.0133723557750614,-0.161227258439486,
-1.5523732824225));
#47018=CARTESIAN_POINT('Ctrl Pts',(0.128313592092439,-0.0985325877424461,
-1.54442599111455));
#47019=CARTESIAN_POINT('Ctrl Pts',(0.152312229038119,0.0545347013224366,
-1.5364786998066));
#47020=CARTESIAN_POINT('Ctrl Pts',(0.0366123635594306,0.157583576547431,
-1.52853140849865));
#47021=CARTESIAN_POINT('Ctrl Pts',(-0.112667815146693,0.116099148114697,
-1.5205841171907));
#47022=CARTESIAN_POINT('Ctrl Pts',(-0.158610755951326,-0.0318696855873517,
-1.51263682588274));
#47023=CARTESIAN_POINT('Ctrl Pts',(-0.059078279484957,-0.150608119488907,
-1.50468953457479));
#47024=CARTESIAN_POINT('Ctrl Pts',(0.0946399128755136,-0.131211034801968,
-1.49674224326684));
#47025=CARTESIAN_POINT('Ctrl Pts',(0.161555790137746,0.00853085200062658,
-1.48879495195889));
#47026=CARTESIAN_POINT('Ctrl Pts',(0.0802951087430872,0.140448368715423,
-1.48084766065094));
#47027=CARTESIAN_POINT('Ctrl Pts',(-0.0746110475700918,0.143548738564228,
-1.47290036934299));
#47028=CARTESIAN_POINT('Ctrl Pts',(-0.161085065008549,0.0149883486108072,
-1.46495307803503));
#47029=CARTESIAN_POINT('Ctrl Pts',(-0.0998142658506054,-0.127319130909666,
-1.45700578672708));
#47030=CARTESIAN_POINT('Ctrl Pts',(0.0530046877002974,-0.152851404457669,
-1.44905849541913));
#47031=CARTESIAN_POINT('Ctrl Pts',(0.157208533062154,-0.0381906519364803,
-1.44111120411118));
#47032=CARTESIAN_POINT('Ctrl Pts',(0.117223059051512,0.111497996347438,
-1.43316391280323));
#47033=CARTESIAN_POINT('Ctrl Pts',(-0.0302776545594956,0.158922347066935,
-1.42521662149528));
#47034=CARTESIAN_POINT('Ctrl Pts',(-0.150008155459448,0.0605854937963053,
-1.41726933018732));
#47035=CARTESIAN_POINT('Ctrl Pts',(-0.13215341582115,-0.0933194698318111,
-1.40932203887937));
#47036=CARTESIAN_POINT('Ctrl Pts',(0.00691046373367479,-0.161633209006915,
-1.40137474757142));
#47037=CARTESIAN_POINT('Ctrl Pts',(0.139636169126457,-0.0816993820942073,
-1.39342745626347));
#47038=CARTESIAN_POINT('Ctrl Pts',(0.14428966498996,0.0731678982886138,
-1.38548016495552));
#47039=CARTESIAN_POINT('Ctrl Pts',(0.01660283439572,0.160926674771202,-1.37753287364757));
#47040=CARTESIAN_POINT('Ctrl Pts',(-0.126311868022924,0.101085907818286,
-1.36958558233961));
#47041=CARTESIAN_POINT('Ctrl Pts',(-0.1533752109502,-0.0514693445544957,
-1.36163829103166));
#47042=CARTESIAN_POINT('Ctrl Pts',(-0.0397651003138635,-0.156817682548608,
-1.35369099972371));
#47043=CARTESIAN_POINT('Ctrl Pts',(0.11031696663014,-0.118335183425778,
-1.34574370841576));
#47044=CARTESIAN_POINT('Ctrl Pts',(0.159217958833437,0.028682579169278,
-1.33779641710781));
#47045=CARTESIAN_POINT('Ctrl Pts',(0.0620866163479071,0.149393108386416,
-1.32984912579986));
#47046=CARTESIAN_POINT('Ctrl Pts',(-0.0919896436874009,0.133082509057925,
-1.3219018344919));
#47047=CARTESIAN_POINT('Ctrl Pts',(-0.161694375954805,-0.00528938063232889,
-1.31395454318395));
#47048=CARTESIAN_POINT('Ctrl Pts',(-0.0830954407230262,-0.138809929378031,
-1.306007251876));
#47049=CARTESIAN_POINT('Ctrl Pts',(0.0717173921098091,-0.145016083355798,
-1.29805996056805));
#47050=CARTESIAN_POINT('Ctrl Pts',(0.160752103653288,-0.0182156507962345,
-1.2901126692601));
#47051=CARTESIAN_POINT('Ctrl Pts',(0.102347385784237,0.125291904710641,
-1.28216537795215));
#47052=CARTESIAN_POINT('Ctrl Pts',(-0.0499288262609556,0.153883595847937,
-1.2742180866442));
#47053=CARTESIAN_POINT('Ctrl Pts',(-0.156411064306094,0.0413355503836927,
-1.26627079533624));
#47054=CARTESIAN_POINT('Ctrl Pts',(-0.119435409415436,-0.109124844745158,
-1.25832350402829));
#47055=CARTESIAN_POINT('Ctrl Pts',(0.0270846197985837,-0.15949756152761,
-1.25037621272034));
#47056=CARTESIAN_POINT('Ctrl Pts',(0.148763040111663,-0.0635814962046623,
-1.24242892141239));
#47057=CARTESIAN_POINT('Ctrl Pts',(0.133998221093683,0.0906505681538529,
-1.23448163010444));
#47058=CARTESIAN_POINT('Ctrl Pts',(-0.00366776569351205,0.161739284831192,
-1.22653433879648));
#47059=CARTESIAN_POINT('Ctrl Pts',(-0.137969732547029,0.0844831442584205,
-1.21858704748853));
#47060=CARTESIAN_POINT('Ctrl Pts',(-0.145727920621714,-0.0702596748793999,
-1.21063975618058));
#47061=CARTESIAN_POINT('Ctrl Pts',(-0.019826635646634,-0.160561369207613,
-1.20269246487263));
#47062=CARTESIAN_POINT('Ctrl Pts',(0.124259343528249,-0.103598572909169,
-1.19474517356468));
#47063=CARTESIAN_POINT('Ctrl Pts',(0.154376508033714,0.0483832877159527,
-1.18679788225673));
#47064=CARTESIAN_POINT('Ctrl Pts',(0.0429018442401126,0.155988719219323,
-1.17885059094878));
#47065=CARTESIAN_POINT('Ctrl Pts',(-0.107921750558149,0.120523626394796,
-1.17090329964082));
#47066=CARTESIAN_POINT('Ctrl Pts',(-0.159761127035922,-0.0254839371192833,
-1.16295600833287));
#47067=CARTESIAN_POINT('Ctrl Pts',(-0.0650699830591519,-0.148118013987393,
-1.15500871702492));
#47068=CARTESIAN_POINT('Ctrl Pts',(0.0893023778727434,-0.134900459855264,
-1.14706142571697));
#47069=CARTESIAN_POINT('Ctrl Pts',(0.161767931120567,0.00204578196761214,
-1.13911413440902));
#47070=CARTESIAN_POINT('Ctrl Pts',(0.0858623531693627,0.137115663113691,
-1.13116684310107));
#47071=CARTESIAN_POINT('Ctrl Pts',(-0.0687948931681688,0.146425105213786,
-1.12321955179312));
#47072=CARTESIAN_POINT('Ctrl Pts',(-0.160354490612175,0.0214356269653556,
-1.11527226048516));
#47073=CARTESIAN_POINT('Ctrl Pts',(-0.104839343388522,-0.123214288297872,
-1.10732496917721));
#47074=CARTESIAN_POINT('Ctrl Pts',(0.0468328843205382,-0.154853897946118,
-1.09937767786926));
#47075=CARTESIAN_POINT('Ctrl Pts',(0.155550689754317,-0.0444638243951627,
-1.09143038656131));
#47076=CARTESIAN_POINT('Ctrl Pts',(0.121599724945644,0.106707805038019,
-1.08348309525336));
#47077=CARTESIAN_POINT('Ctrl Pts',(-0.0238806920770757,0.160008628857346,
-1.0755358039454));
#47078=CARTESIAN_POINT('Ctrl Pts',(-0.147458094869793,0.0665519272467647,
-1.06758851263745));
#47079=CARTESIAN_POINT('Ctrl Pts',(-0.135789134624223,-0.0879452084021196,
-1.0596412213295));
#47080=CARTESIAN_POINT('Ctrl Pts',(0.000423592542104506,-0.161780311942603,
-1.05169393002155));
#47081=CARTESIAN_POINT('Ctrl Pts',(0.136247806953129,-0.0872329287789347,
-1.0437466387136));
#47082=CARTESIAN_POINT('Ctrl Pts',(0.147107567031384,0.0673231942572166,
-1.03579934740565));
#47083=CARTESIAN_POINT('Ctrl Pts',(0.023042462971293,0.160131488668233,
-1.0278520560977));
#47084=CARTESIAN_POINT('Ctrl Pts',(-0.122156844097886,0.106069572465116,
-1.01990476478974));
#47085=CARTESIAN_POINT('Ctrl Pts',(-0.155315717584476,-0.0452777719649154,
-1.01195747348179));
#47086=CARTESIAN_POINT('Ctrl Pts',(-0.0460213337946129,-0.155097019954134,
-1.00401018217384));
#47087=CARTESIAN_POINT('Ctrl Pts',(0.105483130244754,-0.122663596868249,
-0.996062890865889));
#47088=CARTESIAN_POINT('Ctrl Pts',(0.160240042106027,0.022275045875293,
-0.988115599557937));
#47089=CARTESIAN_POINT('Ctrl Pts',(0.0680271797607449,0.146783349112517,
-0.980168308249986));
#47090=CARTESIAN_POINT('Ctrl Pts',(-0.0865791962028742,0.13666415604595,
-0.972221016942034));
#47091=CARTESIAN_POINT('Ctrl Pts',(-0.161776426052429,0.00119863947484806,
-0.964273725634083));
#47092=CARTESIAN_POINT('Ctrl Pts',(-0.0885947332782831,-0.135366251326679,
-0.956326434326131));
#47093=CARTESIAN_POINT('Ctrl Pts',(0.0658447261231557,-0.147775237454231,
-0.948379143018179));
#47094=CARTESIAN_POINT('Ctrl Pts',(0.159892385798223,-0.0246469821000468,
-0.940431851710227));
#47095=CARTESIAN_POINT('Ctrl Pts',(0.107289136441681,0.121087117252359,
-0.932484560402278));
#47096=CARTESIAN_POINT('Ctrl Pts',(-0.0437181070127741,0.155761920513673,
-0.924537269094323));
#47097=CARTESIAN_POINT('Ctrl Pts',(-0.154627755434431,0.0475742158337616,
-0.916589977786374));
#47098=CARTESIAN_POINT('Ctrl Pts',(-0.123715135192255,-0.104247849317143,
-0.908642686478421));
#47099=CARTESIAN_POINT('Ctrl Pts',(0.020667159958694,-0.160455343513793,
-0.90069539517047));
#47100=CARTESIAN_POINT('Ctrl Pts',(0.146093844560002,-0.0694955922671763,
-0.892748103862517));
#47101=CARTESIAN_POINT('Ctrl Pts',(0.137525436138657,0.0852044786250095,
-0.884800812554568));
#47102=CARTESIAN_POINT('Ctrl Pts',(0.00282075097081221,0.161756273840766,
-0.876853521246614));
#47103=CARTESIAN_POINT('Ctrl Pts',(-0.134471084873137,0.0899476297404762,
-0.868906229938664));
#47104=CARTESIAN_POINT('Ctrl Pts',(-0.148428049349295,-0.0643596374232403,
-0.86095893863071));
#47105=CARTESIAN_POINT('Ctrl Pts',(-0.0262490230201646,-0.159637206043499,
-0.85301164732276));
#47106=CARTESIAN_POINT('Ctrl Pts',(0.120005215320353,-0.108497912693302,
-0.845064356014807));
#47107=CARTESIAN_POINT('Ctrl Pts',(0.156192461868825,0.0421540462855391,
-0.837117064706857));
#47108=CARTESIAN_POINT('Ctrl Pts',(0.0491223143731926,0.154142943378894,
-0.829169773398904));
#47109=CARTESIAN_POINT('Ctrl Pts',(-0.103002086460407,0.124754234187424,
-0.821222482090954));
#47110=CARTESIAN_POINT('Ctrl Pts',(-0.160654511432484,-0.0190571959972504,
-0.813275190783002));
#47111=CARTESIAN_POINT('Ctrl Pts',(-0.0709570171198838,-0.145389650540663,
-0.805327899475051));
#47112=CARTESIAN_POINT('Ctrl Pts',(0.0838211938938518,-0.138372888302216,
-0.797380608167099));
#47113=CARTESIAN_POINT('Ctrl Pts',(0.161719857333879,-0.0044425788454637,
-0.789433316859147));
#47114=CARTESIAN_POINT('Ctrl Pts',(0.0912914821342712,0.133562397599832,
-0.781486025551195));
#47115=CARTESIAN_POINT('Ctrl Pts',(-0.0628680774803865,0.149065937077549,
-0.773538734243243));
#47116=CARTESIAN_POINT('Ctrl Pts',(-0.159365975061913,0.027848424649403,
-0.765591442935292));
#47117=CARTESIAN_POINT('Ctrl Pts',(-0.109695779679766,-0.118911247085109,
-0.757644151627341));
#47118=CARTESIAN_POINT('Ctrl Pts',(0.0405857470466367,-0.156607298359796,
-0.74969686031939));
#47119=CARTESIAN_POINT('Ctrl Pts',(0.15364263253448,-0.0506654737544443,
-0.741749569011437));
#47120=CARTESIAN_POINT('Ctrl Pts',(0.125780789374263,0.101745966933707,
-0.733802277703486));
#47121=CARTESIAN_POINT('Ctrl Pts',(-0.0174453158698736,0.160837525836132,
-0.725854986395534));
#47122=CARTESIAN_POINT('Ctrl Pts',(-0.144670837859916,0.0724113073752861,
-0.717907695087582));
#47123=CARTESIAN_POINT('Ctrl Pts',(-0.139206427326868,-0.0824294810961295,
-0.709960403779631));
#47124=CARTESIAN_POINT('Ctrl Pts',(-0.00606396002700117,-0.161667180193379,
-0.702013112471679));
#47125=CARTESIAN_POINT('Ctrl Pts',(0.1326402808736,-0.0926261553377884,
-0.694065821163729));
#47126=CARTESIAN_POINT('Ctrl Pts',(0.149688836500554,0.0613701962682061,
-0.686118529855775));
#47127=CARTESIAN_POINT('Ctrl Pts',(0.0294450261708669,0.159078720125241,
-0.678171238547825));
#47128=CARTESIAN_POINT('Ctrl Pts',(-0.117805322543121,0.110882616957749,
-0.670223947239873));
#47129=CARTESIAN_POINT('Ctrl Pts',(-0.157006388275539,-0.0390133669856671,
-0.662276655931922));
#47130=CARTESIAN_POINT('Ctrl Pts',(-0.0522035388156852,-0.153126873206524,
-0.65432936462397));
#47131=CARTESIAN_POINT('Ctrl Pts',(0.10047961703755,-0.12679469753454,-0.646382073316018));
#47132=CARTESIAN_POINT('Ctrl Pts',(0.161004368322975,0.0158316816481386,
-0.638434782008066));
#47133=CARTESIAN_POINT('Ctrl Pts',(0.0738583168071857,0.143937478793041,
-0.630487490700115));
#47134=CARTESIAN_POINT('Ctrl Pts',(-0.081029480165993,0.14002596940181,
-0.622540199392163));
#47135=CARTESIAN_POINT('Ctrl Pts',(-0.161598247715861,0.00768473148853606,
-0.614592908084211));
#47136=CARTESIAN_POINT('Ctrl Pts',(-0.0939515151520932,-0.131704827411578,
-0.60664561677626));
#47137=CARTESIAN_POINT('Ctrl Pts',(0.0598661443958943,-0.15029668498692,
-0.598698325468309));
#47138=CARTESIAN_POINT('Ctrl Pts',(0.158775470116437,-0.0310386670492156,
-0.590751034160357));
#47139=CARTESIAN_POINT('Ctrl Pts',(0.112058305192951,0.116687552893062,
-0.582803742852405));
#47140=CARTESIAN_POINT('Ctrl Pts',(-0.0374370642025506,0.1573896914883,
-0.574856451544454));
#47141=CARTESIAN_POINT('Ctrl Pts',(-0.152595717253679,0.0537363549073017,
-0.566909160236501));
#47142=CARTESIAN_POINT('Ctrl Pts',(-0.127795856721654,-0.0992031641010812,
-0.558961868928551));
#47143=CARTESIAN_POINT('Ctrl Pts',(0.0142164555799897,-0.161155022117307,
-0.551014577620598));
#47144=CARTESIAN_POINT('Ctrl Pts',(0.143189647077946,-0.0752978999214523,
-0.543067286312648));
#47145=CARTESIAN_POINT('Ctrl Pts',(0.140831432123592,0.0796213318709609,
-0.535119995004695));
#47146=CARTESIAN_POINT('Ctrl Pts',(0.00930473026448263,0.161513066832355,
-0.527172703696745));
#47147=CARTESIAN_POINT('Ctrl Pts',(-0.130756131271888,0.0952674283146994,
-0.519225412388792));
#47148=CARTESIAN_POINT('Ctrl Pts',(-0.150889421418604,-0.0583560730930949,
-0.51127812108084));
#47149=CARTESIAN_POINT('Ctrl Pts',(-0.0326291870467958,-0.158456255526732,
-0.50333082977289));
#47150=CARTESIAN_POINT('Ctrl Pts',(0.115558050524615,-0.113222726172084,
-0.495383538464937));
#47151=CARTESIAN_POINT('Ctrl Pts',(0.157757169457645,0.0358569971916244,
-0.487436247156986));
#47152=CARTESIAN_POINT('Ctrl Pts',(0.0552637679074694,0.152049218082689,
-0.479488955849034));
#47153=CARTESIAN_POINT('Ctrl Pts',(-0.0979167364692866,0.128784166270905,
-0.471541664541083));
#47154=CARTESIAN_POINT('Ctrl Pts',(-0.161289472071172,-0.0125998000734305,
-0.463594373233132));
#47155=CARTESIAN_POINT('Ctrl Pts',(-0.0767299119706533,-0.142427417907731,
-0.455647081925179));
#47156=CARTESIAN_POINT('Ctrl Pts',(0.0782051777977488,-0.141622734504423,
-0.447699790617228));
#47157=CARTESIAN_POINT('Ctrl Pts',(0.161411646107643,-0.0109237934669493,
-0.439752499309276));
#47158=CARTESIAN_POINT('Ctrl Pts',(0.0965737625129634,0.129794287844178,
-0.431805208001325));
#47159=CARTESIAN_POINT('Ctrl Pts',(-0.0568401341946973,0.151466986197049,
-0.423857916693373));
#47160=CARTESIAN_POINT('Ctrl Pts',(-0.158121108452566,0.0342164262397469,
-0.415910625385421));
#47161=CARTESIAN_POINT('Ctrl Pts',(-0.114375762814762,-0.114416929007158,
-0.40796333407747));
#47162=CARTESIAN_POINT('Ctrl Pts',(0.0342733248257124,-0.158108785234341,
-0.400016042769518));
#47163=CARTESIAN_POINT('Ctrl Pts',(0.151487430643043,-0.0567856242376266,
-0.392068751461566));
#47164=CARTESIAN_POINT('Ctrl Pts',(0.129759526809581,0.0966204634900976,
-0.384121460153615));
#47165=CARTESIAN_POINT('Ctrl Pts',(-0.0109818776801944,0.161407704665871,
-0.376174168845663));
#47166=CARTESIAN_POINT('Ctrl Pts',(-0.141650867923135,0.0781542089686166,
-0.368226877537712));
#47167=CARTESIAN_POINT('Ctrl Pts',(-0.142399796980305,-0.0767811603380389,
-0.36027958622976));
#47168=CARTESIAN_POINT('Ctrl Pts',(-0.0125417583021156,-0.161293995739392,
-0.352332294921809));
#47169=CARTESIAN_POINT('Ctrl Pts',(0.128819393840036,-0.0978703863973884,
-0.344385003613857));
#47170=CARTESIAN_POINT('Ctrl Pts',(0.152029321249178,0.0553184801255625,
-0.336437712305906));
#47171=CARTESIAN_POINT('Ctrl Pts',(0.0358002250341034,0.157770062592353,
-0.328490420997953));
#47172=CARTESIAN_POINT('Ctrl Pts',(-0.113264303078354,0.115517299185288,
-0.320543129690002));
#47173=CARTESIAN_POINT('Ctrl Pts',(-0.15844450346407,-0.0326862063401563,
-0.312595838382051));
#47174=CARTESIAN_POINT('Ctrl Pts',(-0.0583017708779276,-0.150910411421424,
-0.304648547074099));
#47175=CARTESIAN_POINT('Ctrl Pts',(0.0953144755013862,-0.130721840266996,
-0.296701255766148));
#47176=CARTESIAN_POINT('Ctrl Pts',(0.161509708013311,0.00936285107942815,
-0.288753964458196));
#47177=CARTESIAN_POINT('Ctrl Pts',(0.0795706477049501,0.140860075204769,
-0.280806673150245));
#47178=CARTESIAN_POINT('Ctrl Pts',(-0.0753494226742529,0.143162541419151,
-0.272859381842292));
#47179=CARTESIAN_POINT('Ctrl Pts',(-0.161160127556965,0.0141584620863805,
-0.264912090534341));
#47180=CARTESIAN_POINT('Ctrl Pts',(-0.0991571695951433,-0.127831547282851,
-0.256964799226389));
#47181=CARTESIAN_POINT('Ctrl Pts',(0.0537912638857975,-0.152576370034002,
-0.249017507918438));
#47182=CARTESIAN_POINT('Ctrl Pts',(0.157403153241977,-0.0373804241803696,
-0.241070216610486));
#47183=CARTESIAN_POINT('Ctrl Pts',(0.11664722050643,0.112100288629876,-0.233122925302535));
#47184=CARTESIAN_POINT('Ctrl Pts',(-0.03109580132088,0.15876429039619,-0.225175633994583));
#47185=CARTESIAN_POINT('Ctrl Pts',(-0.150318218428302,0.059812055372734,
-0.217228342686632));
#47186=CARTESIAN_POINT('Ctrl Pts',(-0.131671009899015,-0.0939989037990694,
-0.20928105137868));
#47187=CARTESIAN_POINT('Ctrl Pts',(0.00774288308919283,-0.161595471892866,
-0.201333760070728));
#47188=CARTESIAN_POINT('Ctrl Pts',(0.140055119212391,-0.0809790856917334,
-0.193386468762777));
#47189=CARTESIAN_POINT('Ctrl Pts',(0.143910891228999,0.0739101086366355,
-0.185439177454825));
#47190=CARTESIAN_POINT('Ctrl Pts',(0.0157737420722441,0.161010055264145,
-0.177491886146873));
#47191=CARTESIAN_POINT('Ctrl Pts',(-0.126830847136387,0.100433982260212,
-0.169544594838921));
#47192=CARTESIAN_POINT('Ctrl Pts',(-0.153108078234609,-0.0522586381566147,
-0.16159730353097));
#47193=CARTESIAN_POINT('Ctrl Pts',(-0.0389568634868797,-0.157020418959173,
-0.153650012223018));
#47194=CARTESIAN_POINT('Ctrl Pts',(0.110925000223214,-0.117765410005127,
-0.145702720915067));
#47195=CARTESIAN_POINT('Ctrl Pts',(0.159068118580144,0.0295022636793513,
-0.137755429607115));
#47196=CARTESIAN_POINT('Ctrl Pts',(0.0613163169383187,0.149710922597531,
-0.129808138299164));
#47197=CARTESIAN_POINT('Ctrl Pts',(-0.0926738637166896,0.132606918649559,
-0.121860846991212));
#47198=CARTESIAN_POINT('Ctrl Pts',(-0.161665019843371,-0.00612209556041882,
-0.11391355568326));
#47199=CARTESIAN_POINT('Ctrl Pts',(-0.0823793202671913,-0.13923615876769,
-0.105966264375309));
#47200=CARTESIAN_POINT('Ctrl Pts',(0.072463247076575,-0.144644623334344,
-0.098018973067357));
#47201=CARTESIAN_POINT('Ctrl Pts',(0.160844013877,-0.0173877164374548,-0.0900716817594055));
#47202=CARTESIAN_POINT('Ctrl Pts',(0.10170027857703,0.125817926598835,-0.0821243904514541));
#47203=CARTESIAN_POINT('Ctrl Pts',(-0.0507199647238506,0.153623381518765,
-0.0741770991435023));
#47204=CARTESIAN_POINT('Ctrl Pts',(-0.156623402096616,0.0405313031445145,
-0.0662298078355511));
#47205=CARTESIAN_POINT('Ctrl Pts',(-0.118868900789494,-0.109742197881292,
-0.0582825165275991));
#47206=CARTESIAN_POINT('Ctrl Pts',(0.027900335514407,-0.15934904467435,
-0.0503352252196477));
#47207=CARTESIAN_POINT('Ctrl Pts',(0.14909887050496,-0.0628275280611914,
-0.042387933911696));
#47208=CARTESIAN_POINT('Ctrl Pts',(0.133509936600416,0.0913644220801899,
-0.0344406426037444));
#47209=CARTESIAN_POINT('Ctrl Pts',(-0.0044634589477341,0.161670816842846,
-0.0264933512957926));
#47210=CARTESIAN_POINT('Ctrl Pts',(-0.138474820834309,0.0838631351225796,
-0.0185460599878411));
#47211=CARTESIAN_POINT('Ctrl Pts',(-0.145219806667121,-0.0711978527135158,
-0.0105987686798896));
#47212=CARTESIAN_POINT('Ctrl Pts',(-0.0613018075622001,-0.130529025318469,
-0.00530057447458853));
#47213=CARTESIAN_POINT('Ctrl Pts',(-0.0160685904325773,-0.135878184512857,
-0.00265147737193801));
#47214=CARTESIAN_POINT('Ctrl Pts',(0.128823493644022,-0.069446598083337,
-2.93765));
#47215=CARTESIAN_POINT('Ctrl Pts',(0.151941943903563,-0.0265618548091487,
-2.93500090289735));
#47216=CARTESIAN_POINT('Ctrl Pts',(0.151580971107978,0.0833657122950276,
-2.92970270869205));
#47217=CARTESIAN_POINT('Ctrl Pts',(0.0116953364202053,0.172764245811242,
-2.9217554173841));
#47218=CARTESIAN_POINT('Ctrl Pts',(-0.138782966866511,0.103272893425666,
-2.91380812607614));
#47219=CARTESIAN_POINT('Ctrl Pts',(-0.162037660106299,-0.0607202061494744,
-2.9058608347682));
#47220=CARTESIAN_POINT('Ctrl Pts',(-0.0366395801762509,-0.169135679591106,
-2.89791354346024));
#47221=CARTESIAN_POINT('Ctrl Pts',(0.12234579575611,-0.122362484441713,
-2.88996625215229));
#47222=CARTESIAN_POINT('Ctrl Pts',(0.169126899538293,0.0366081863273628,
-2.88201896084434));
#47223=CARTESIAN_POINT('Ctrl Pts',(0.0607823503659455,0.162019005104728,
-2.87407166953639));
#47224=CARTESIAN_POINT('Ctrl Pts',(-0.103308236397252,0.138819650059126,
-2.86612437822844));
#47225=CARTESIAN_POINT('Ctrl Pts',(-0.172647435005854,-0.0116983995188776,
-2.85817708692048));
#47226=CARTESIAN_POINT('Ctrl Pts',(-0.0836362547964333,-0.151489283614881,
-2.85022979561253));
#47227=CARTESIAN_POINT('Ctrl Pts',(0.0820844654854486,-0.15233517728973,
-2.84228250430458));
#47228=CARTESIAN_POINT('Ctrl Pts',(0.172518741936108,-0.0134621957780814,
-2.83433521299663));
#47229=CARTESIAN_POINT('Ctrl Pts',(0.104721297396897,0.137758466350652,
-2.82638792168868));
#47230=CARTESIAN_POINT('Ctrl Pts',(-0.0591249014323184,0.162628932530307,
-2.81844063038073));
#47231=CARTESIAN_POINT('Ctrl Pts',(-0.168742653009007,0.0383386685899805,
-2.81049333907278));
#47232=CARTESIAN_POINT('Ctrl Pts',(-0.123592147011918,-0.121115301787186,
-2.80254604776482));
#47233=CARTESIAN_POINT('Ctrl Pts',(0.0349152227561978,-0.169484098237391,
-2.79459875645688));
#47234=CARTESIAN_POINT('Ctrl Pts',(0.161398875831068,-0.0624046246492733,
-2.78665146514892));
#47235=CARTESIAN_POINT('Ctrl Pts',(0.139849887428109,0.101911446560615,
-2.77870417384097));
#47236=CARTESIAN_POINT('Ctrl Pts',(-0.00996732853818697,0.172755856534424,
-2.77075688253302));
#47237=CARTESIAN_POINT('Ctrl Pts',(-0.150642660216236,0.0851511762825492,
-2.76280959122507));
#47238=CARTESIAN_POINT('Ctrl Pts',(-0.153150792732914,-0.0805528926453607,
-2.75486229991711));
#47239=CARTESIAN_POINT('Ctrl Pts',(-0.0151913048999562,-0.172375050522329,
-2.74691500860916));
#47240=CARTESIAN_POINT('Ctrl Pts',(0.136701421070846,-0.106097385959945,
-2.73896771730121));
#47241=CARTESIAN_POINT('Ctrl Pts',(0.163213644563884,0.0574912171142146,
-2.73102042599326));
#47242=CARTESIAN_POINT('Ctrl Pts',(0.0400287500981403,0.168349734119888,
-2.72307313468531));
#47243=CARTESIAN_POINT('Ctrl Pts',(-0.119869916334605,0.124800388528227,
-2.71512584337735));
#47244=CARTESIAN_POINT('Ctrl Pts',(-0.169825685177861,-0.0332140101527191,
-2.70717855206941));
#47245=CARTESIAN_POINT('Ctrl Pts',(-0.064019871108235,-0.160765014600296,
-2.69923126076145));
#47246=CARTESIAN_POINT('Ctrl Pts',(0.100504012915477,-0.140864747914112,
-2.6912839694535));
#47247=CARTESIAN_POINT('Ctrl Pts',(0.172847116835337,0.00823456242596275,
-2.68333667814555));
#47248=CARTESIAN_POINT('Ctrl Pts',(0.0866574258333968,0.149781255050633,
-2.6753893868376));
#47249=CARTESIAN_POINT('Ctrl Pts',(-0.0790131623320317,0.153950816805319,
-2.66744209552965));
#47250=CARTESIAN_POINT('Ctrl Pts',(-0.172214057687311,0.0169189878994688,
-2.6594948042217));
#47251=CARTESIAN_POINT('Ctrl Pts',(-0.107462790519202,-0.135630684103927,
-2.65154751291375));
#47252=CARTESIAN_POINT('Ctrl Pts',(0.0558517436740735,-0.163781917638226,
-2.64360022160579));
#47253=CARTESIAN_POINT('Ctrl Pts',(0.1679398924462,-0.0417148216086108,
-2.63565293029784));
#47254=CARTESIAN_POINT('Ctrl Pts',(0.125996079239947,0.118612485990478,
-2.62770563898989));
#47255=CARTESIAN_POINT('Ctrl Pts',(-0.0315094567007179,0.170150192345199,
-2.61975834768194));
#47256=CARTESIAN_POINT('Ctrl Pts',(-0.160114989397424,0.0656286826543376,
-2.61181105637399));
#47257=CARTESIAN_POINT('Ctrl Pts',(-0.141865444364848,-0.0990864749188582,
-2.60386376506603));
#47258=CARTESIAN_POINT('Ctrl Pts',(0.00650096816217477,-0.172920997075647,
-2.59591647375808));
#47259=CARTESIAN_POINT('Ctrl Pts',(0.148904789751492,-0.088154962456717,
-2.58796918245013));
#47260=CARTESIAN_POINT('Ctrl Pts',(0.154735361356446,0.0774654875578245,
-2.58002189114218));
#47261=CARTESIAN_POINT('Ctrl Pts',(0.0186449697524707,0.172035748958206,
-2.57207459983422));
#47262=CARTESIAN_POINT('Ctrl Pts',(-0.134546309735667,0.108817389939271,
-2.56412730852628));
#47263=CARTESIAN_POINT('Ctrl Pts',(-0.164333722735227,-0.0542066544684583,
-2.55618001721832));
#47264=CARTESIAN_POINT('Ctrl Pts',(-0.0433966987745295,-0.167513164712969,
-2.54823272591038));
#47265=CARTESIAN_POINT('Ctrl Pts',(0.117343129381529,-0.127179101284886,
-2.54028543460242));
#47266=CARTESIAN_POINT('Ctrl Pts',(0.1704575912232,0.0298017350344859,-2.53233814329447));
#47267=CARTESIAN_POINT('Ctrl Pts',(0.0672308953579195,0.159448864925574,
-2.52439085198652));
#47268=CARTESIAN_POINT('Ctrl Pts',(-0.0976589739600992,0.142851876507598,
-2.51644356067857));
#47269=CARTESIAN_POINT('Ctrl Pts',(-0.172977490428231,-0.00476672023854133,
-2.50849626937062));
#47270=CARTESIAN_POINT('Ctrl Pts',(-0.0896436352611125,-0.148013352349895,
-2.50054897806266));
#47271=CARTESIAN_POINT('Ctrl Pts',(0.075910023771653,-0.155504347552306,
-2.49260168675471));
#47272=CARTESIAN_POINT('Ctrl Pts',(0.171840142351577,-0.0203690768880506,
-2.48465439544676));
#47273=CARTESIAN_POINT('Ctrl Pts',(0.110161047971342,0.133448406983887,
-2.47670710413881));
#47274=CARTESIAN_POINT('Ctrl Pts',(-0.0525561148836437,0.164869004379291,
-2.46875981283085));
#47275=CARTESIAN_POINT('Ctrl Pts',(-0.167069593839744,0.0450742124823536,
-2.46081252152291));
#47276=CARTESIAN_POINT('Ctrl Pts',(-0.128349335705578,-0.116061974137174,
-2.45286523021495));
#47277=CARTESIAN_POINT('Ctrl Pts',(0.028091016858721,-0.170747850904556,
-2.444917938907));
#47278=CARTESIAN_POINT('Ctrl Pts',(0.158766708164214,-0.0688263481188763,
-2.43697064759905));
#47279=CARTESIAN_POINT('Ctrl Pts',(0.143823945157437,0.0962216535714894,
-2.4290233562911));
#47280=CARTESIAN_POINT('Ctrl Pts',(-0.00303199302997265,0.173016591212946,
-2.42107606498315));
#47281=CARTESIAN_POINT('Ctrl Pts',(-0.147107032478502,0.0911232945631927,
-2.4131287736752));
#47282=CARTESIAN_POINT('Ctrl Pts',(-0.15625769807261,-0.0743469273724919,
-2.40518148236724));
#47283=CARTESIAN_POINT('Ctrl Pts',(-0.0220911359504884,-0.17162725753533,
-2.39723419105929));
#47284=CARTESIAN_POINT('Ctrl Pts',(0.132337086240727,-0.111493629513062,
-2.38928689975134));
#47285=CARTESIAN_POINT('Ctrl Pts',(0.165387708748813,0.0509002908783366,
-2.38133960844339));
#47286=CARTESIAN_POINT('Ctrl Pts',(0.0467471940611836,0.166609224426762,
-2.37339231713544));
#47287=CARTESIAN_POINT('Ctrl Pts',(-0.114769149075218,0.129506664837111,
-2.36544502582749));
#47288=CARTESIAN_POINT('Ctrl Pts',(-0.171020942204186,-0.0263774741829819,
-2.35749773451953));
#47289=CARTESIAN_POINT('Ctrl Pts',(-0.0704148805173739,-0.158068587702951,
-2.34955044321158));
#47290=CARTESIAN_POINT('Ctrl Pts',(0.0947746582729476,-0.144781552574654,
-2.34160315190363));
#47291=CARTESIAN_POINT('Ctrl Pts',(0.173038295498278,0.00129696096009361,
-2.33365586059568));
#47292=CARTESIAN_POINT('Ctrl Pts',(0.0925937915859414,0.146185921266108,
-2.32570856928773));
#47293=CARTESIAN_POINT('Ctrl Pts',(-0.0727763555268022,0.15699533716935,
-2.31776127797977));
#47294=CARTESIAN_POINT('Ctrl Pts',(-0.171397115914642,0.0238109737899195,
-2.30981398667183));
#47295=CARTESIAN_POINT('Ctrl Pts',(-0.112815000575814,-0.131212459247438,
-2.30186669536387));
#47296=CARTESIAN_POINT('Ctrl Pts',(0.0492393489425894,-0.165889783689024,
-2.29391940405592));
#47297=CARTESIAN_POINT('Ctrl Pts',(0.166132102763322,-0.048415475295804,
-2.28597211274797));
#47298=CARTESIAN_POINT('Ctrl Pts',(0.130650972312169,0.113464784186839,
-2.27802482144002));
#47299=CARTESIAN_POINT('Ctrl Pts',(-0.0246612793008269,0.171276837663264,
-2.27007753013207));
#47300=CARTESIAN_POINT('Ctrl Pts',(-0.157354573736509,0.0719963328294086,
-2.26213023882412));
#47301=CARTESIAN_POINT('Ctrl Pts',(-0.145724602473588,-0.0933181335571831,
-2.25418294751616));
#47302=CARTESIAN_POINT('Ctrl Pts',(-0.000438201516819747,-0.173042601101902,
-2.24623565620821));
#47303=CARTESIAN_POINT('Ctrl Pts',(0.145250111328747,-0.0940549784735931,
-2.23828836490026));
#47304=CARTESIAN_POINT('Ctrl Pts',(0.157717190674275,0.0711984661526903,
-2.23034107359231));
#47305=CARTESIAN_POINT('Ctrl Pts',(0.0255284174798185,0.171149740629828,
-2.22239378228436));
#47306=CARTESIAN_POINT('Ctrl Pts',(-0.130074639083192,0.114125028298172,
-2.2144464909764));
#47307=CARTESIAN_POINT('Ctrl Pts',(-0.166375178717216,-0.0475734560810524,
-2.20649919966846));
#47308=CARTESIAN_POINT('Ctrl Pts',(-0.0500788884436116,-0.165638276823124,
-2.1985519083605));
#47309=CARTESIAN_POINT('Ctrl Pts',(0.112149010623523,-0.131782143072748,
-2.19060461705255));
#47310=CARTESIAN_POINT('Ctrl Pts',(0.171515511551972,0.0229426047724884,
-2.1826573257446));
#47311=CARTESIAN_POINT('Ctrl Pts',(0.0735705460428639,0.156624738057678,
-2.17471003443665));
#47312=CARTESIAN_POINT('Ctrl Pts',(-0.0918522258750713,0.146653000032309,
-2.1667627431287));
#47313=CARTESIAN_POINT('Ctrl Pts',(-0.173029507590898,0.00217331993337852,
-2.15881545182074));
#47314=CARTESIAN_POINT('Ctrl Pts',(-0.0955067083065008,-0.144299696760383,
-2.15086816051279));
#47315=CARTESIAN_POINT('Ctrl Pts',(0.0696134179040222,-0.158423186006346,
-2.14292086920484));
#47316=CARTESIAN_POINT('Ctrl Pts',(0.170885156554018,-0.0272432943343881,
-2.13497357789689));
#47317=CARTESIAN_POINT('Ctrl Pts',(0.115423580959264,0.12892374015371,-2.12702628658893));
#47318=CARTESIAN_POINT('Ctrl Pts',(-0.0459027797961832,0.166843845027812,
-2.11907899528099));
#47319=CARTESIAN_POINT('Ctrl Pts',(-0.165127796259457,0.0517372662514804,
-2.11113170397303));
#47320=CARTESIAN_POINT('Ctrl Pts',(-0.132900063381712,-0.110821960683875,
-2.10318441266508));
#47321=CARTESIAN_POINT('Ctrl Pts',(0.0212216234075226,-0.171736939872093,
-2.09523712135713));
#47322=CARTESIAN_POINT('Ctrl Pts',(0.155879154050091,-0.0751373618735018,
-2.08728983004918));
#47323=CARTESIAN_POINT('Ctrl Pts',(0.147566651902153,0.0903770826209298,
-2.07934253874123));
#47324=CARTESIAN_POINT('Ctrl Pts',(0.00390821982662287,0.172999016281793,
-2.07139524743328));
#47325=CARTESIAN_POINT('Ctrl Pts',(-0.143334773123449,0.0969488351159036,
-2.06344795612533));
#47326=CARTESIAN_POINT('Ctrl Pts',(-0.159113252179034,-0.0680213701544789,
-2.05550066481737));
#47327=CARTESIAN_POINT('Ctrl Pts',(-0.0289554319259212,-0.170603390290653,
-2.04755337350942));
#47328=CARTESIAN_POINT('Ctrl Pts',(0.127759878179759,-0.116710527992013,
-2.03960608220147));
#47329=CARTESIAN_POINT('Ctrl Pts',(0.167295735497278,0.044227488071404,
-2.03165879089352));
#47330=CARTESIAN_POINT('Ctrl Pts',(0.0533904419725765,0.164600712400203,
-2.02371149958557));
#47331=CARTESIAN_POINT('Ctrl Pts',(-0.109483767800323,0.134004620834232,
-2.01576420827762));
#47332=CARTESIAN_POINT('Ctrl Pts',(-0.171941100359414,-0.0194985082474348,
-2.00781691696966));
#47333=CARTESIAN_POINT('Ctrl Pts',(-0.0766966227808798,-0.155117896680843,
-1.99986962566171));
#47334=CARTESIAN_POINT('Ctrl Pts',(0.0888928521176931,-0.148465466217109,
-1.99192233435376));
#47335=CARTESIAN_POINT('Ctrl Pts',(0.172951130240434,-0.00564272675556493,
-1.98397504304581));
#47336=CARTESIAN_POINT('Ctrl Pts',(0.0983812138986072,0.142355437439242,
-1.97602775173786));
#47337=CARTESIAN_POINT('Ctrl Pts',(-0.06642248298153,0.159787319807454,
-1.96808046042991));
#47338=CARTESIAN_POINT('Ctrl Pts',(-0.17030447017081,0.0306646581021379,
-1.96013316912195));
#47339=CARTESIAN_POINT('Ctrl Pts',(-0.117985739996266,-0.126583170185515,
-1.952185877814));
#47340=CARTESIAN_POINT('Ctrl Pts',(0.0425477493542096,-0.167730804688861,
-1.94423858650605));
#47341=CARTESIAN_POINT('Ctrl Pts',(0.164057078242671,-0.0550382493831285,
-1.9362912951981));
#47342=CARTESIAN_POINT('Ctrl Pts',(0.135095704369094,0.108134566525693,
-1.92834400389014));
#47343=CARTESIAN_POINT('Ctrl Pts',(-0.0177734325482762,0.172127972485977,
-1.9203967125822));
#47344=CARTESIAN_POINT('Ctrl Pts',(-0.154341042492961,0.0782481719841884,
-1.91244942127424));
#47345=CARTESIAN_POINT('Ctrl Pts',(-0.149349352603055,-0.0873996836020006,
-1.90450212996629));
#47346=CARTESIAN_POINT('Ctrl Pts',(-0.00737666631873438,-0.172885854281672,
-1.89655483865834));
#47347=CARTESIAN_POINT('Ctrl Pts',(0.141361788178154,-0.0998037006315704,
-1.88860754735039));
#47348=CARTESIAN_POINT('Ctrl Pts',(0.160445321115353,0.0648169171503288,
-1.88066025604244));
#47349=CARTESIAN_POINT('Ctrl Pts',(0.032370801003498,0.169988426250357,
-1.87271296473448));
#47350=CARTESIAN_POINT('Ctrl Pts',(-0.125393734486796,0.119249088751808,
-1.86476567342654));
#47351=CARTESIAN_POINT('Ctrl Pts',(-0.168149008857156,-0.0408637325392291,
-1.85681838211858));
#47352=CARTESIAN_POINT('Ctrl Pts',(-0.0566805227991419,-0.163496948448273,
-1.84887109081063));
#47353=CARTESIAN_POINT('Ctrl Pts',(0.106774492519686,-0.136173204279861,
-1.84092379950268));
#47354=CARTESIAN_POINT('Ctrl Pts',(0.172297537462134,0.0160465697632314,
-1.83297650819473));
#47355=CARTESIAN_POINT('Ctrl Pts',(0.0797918534780101,0.153548669597705,
-1.82502921688678));
#47356=CARTESIAN_POINT('Ctrl Pts',(-0.0858977272091994,0.150218222186841,
-1.81708192557883));
#47357=CARTESIAN_POINT('Ctrl Pts',(-0.172803194968885,0.0091098641716988,
-1.80913463427087));
#47358=CARTESIAN_POINT('Ctrl Pts',(-0.10121615228637,-0.14035392524979,
-1.80118734296292));
#47359=CARTESIAN_POINT('Ctrl Pts',(0.0632048340975654,-0.16108718994191,
-1.79324005165497));
#47360=CARTESIAN_POINT('Ctrl Pts',(0.169655290306931,-0.0340736890804721,
-1.78529276034702));
#47361=CARTESIAN_POINT('Ctrl Pts',(0.120500447231245,0.124191690679173,
-1.77734546903907));
#47362=CARTESIAN_POINT('Ctrl Pts',(-0.0391756069512533,0.168550305952503,
-1.76939817773112));
#47363=CARTESIAN_POINT('Ctrl Pts',(-0.162920379337028,0.0583170970930484,
-1.76145088642316));
#47364=CARTESIAN_POINT('Ctrl Pts',(-0.1372370122259,-0.105403682535241,
-1.75350359511521));
#47365=CARTESIAN_POINT('Ctrl Pts',(0.0143180935251707,-0.172449778238437,
-1.74555630380726));
#47366=CARTESIAN_POINT('Ctrl Pts',(0.152740857666704,-0.0813275120480199,
-1.73760901249931));
#47367=CARTESIAN_POINT('Ctrl Pts',(0.151071987605236,0.0843871339582318,
-1.72966172119136));
#47368=CARTESIAN_POINT('Ctrl Pts',(0.0108421460446119,0.172703160613315,
-1.72171442988341));
#47369=CARTESIAN_POINT('Ctrl Pts',(-0.139331949992912,0.102618426843595,
-1.71376713857545));
#47370=CARTESIAN_POINT('Ctrl Pts',(-0.161712861748395,-0.0615863959152187,
-1.7058198472675));
#47371=CARTESIAN_POINT('Ctrl Pts',(-0.035773151110808,-0.169305095836731,
-1.69787255595955));
#47372=CARTESIAN_POINT('Ctrl Pts',(0.122977159625931,-0.121739689612795,
-1.6899252646516));
#47373=CARTESIAN_POINT('Ctrl Pts',(0.16893465562522,0.0374835423281985,
-1.68197797334365));
#47374=CARTESIAN_POINT('Ctrl Pts',(0.0599478077103157,0.162327428881901,
-1.67403068203569));
#47375=CARTESIAN_POINT('Ctrl Pts',(-0.104022274404773,0.13828702124328,
-1.66608339072775));
#47376=CARTESIAN_POINT('Ctrl Pts',(-0.172584679507357,-0.0125881776291934,
-1.65813609941979));
#47377=CARTESIAN_POINT('Ctrl Pts',(-0.0828549932865788,-0.151917687923962,
-1.65018880811184));
#47378=CARTESIAN_POINT('Ctrl Pts',(0.082868055736469,-0.151910563013699,
-1.64224151680389));
#47379=CARTESIAN_POINT('Ctrl Pts',(0.172585761273234,-0.0125733377597181,
-1.63429422549594));
#47380=CARTESIAN_POINT('Ctrl Pts',(0.104010383307121,0.138295965165246,
-1.62634693418799));
#47381=CARTESIAN_POINT('Ctrl Pts',(-0.0599617653342634,0.162322273624663,
-1.61839964288004));
#47382=CARTESIAN_POINT('Ctrl Pts',(-0.168937878051169,0.0374690162167301,
-1.61045235157208));
#47383=CARTESIAN_POINT('Ctrl Pts',(-0.122966691292916,-0.121750263445934,
-1.60250506026413));
#47384=CARTESIAN_POINT('Ctrl Pts',(0.035787708804044,-0.169302019229655,
-1.59455776895618));
#47385=CARTESIAN_POINT('Ctrl Pts',(0.161718156702961,-0.0615724906860013,
-1.58661047764823));
#47386=CARTESIAN_POINT('Ctrl Pts',(0.139323125755536,0.102630407026321,
-1.57866318634028));
#47387=CARTESIAN_POINT('Ctrl Pts',(-0.0108569960151533,0.172702227704822,
-1.57071589503232));
#47388=CARTESIAN_POINT('Ctrl Pts',(-0.15107924313768,0.0843741436082613,
-1.56276860372438));
#47389=CARTESIAN_POINT('Ctrl Pts',(-0.152733864095016,-0.0813406452844256,
-1.55482131241642));
#47390=CARTESIAN_POINT('Ctrl Pts',(-0.0143032652488869,-0.172451008752924,
-1.54687402110847));
#47391=CARTESIAN_POINT('Ctrl Pts',(0.137246074933157,-0.105391881718297,
-1.53892672980052));
#47392=CARTESIAN_POINT('Ctrl Pts',(0.162915364295475,0.0583311057083122,
-1.53097943849257));
#47393=CARTESIAN_POINT('Ctrl Pts',(0.0391611138821227,0.168553673873318,
-1.52303214718461));
#47394=CARTESIAN_POINT('Ctrl Pts',(-0.12051112550133,0.124181328898849,
-1.51508485587667));
#47395=CARTESIAN_POINT('Ctrl Pts',(-0.169652359828074,-0.0340882768917243,
-1.50713756456871));
#47396=CARTESIAN_POINT('Ctrl Pts',(-0.0631909826612261,-0.161092624061407,
-1.49919027326076));
#47397=CARTESIAN_POINT('Ctrl Pts',(0.101228220349588,-0.140345221584266,
-1.49124298195281));
#47398=CARTESIAN_POINT('Ctrl Pts',(0.172802411011577,0.00912472275017703,
-1.48329569064486));
#47399=CARTESIAN_POINT('Ctrl Pts',(0.0858848102653002,0.150225607611934,
-1.4753483993369));
#47400=CARTESIAN_POINT('Ctrl Pts',(-0.0798050561804062,0.153541808067782,
-1.46740110802895));
#47401=CARTESIAN_POINT('Ctrl Pts',(-0.172298916601508,0.0160317545710972,
-1.459453816721));
#47402=CARTESIAN_POINT('Ctrl Pts',(-0.106762783169999,-0.136182384861176,
-1.45150652541305));
#47403=CARTESIAN_POINT('Ctrl Pts',(0.0566945809971845,-0.163492074126654,
-1.4435592341051));
#47404=CARTESIAN_POINT('Ctrl Pts',(0.168152521934197,-0.0408492739696887,
-1.43561194279715));
#47405=CARTESIAN_POINT('Ctrl Pts',(0.125383480301026,0.119259870385153,
-1.42766465148919));
#47406=CARTESIAN_POINT('Ctrl Pts',(-0.0323854174659853,0.169985642194378,
-1.41971736018125));
#47407=CARTESIAN_POINT('Ctrl Pts',(-0.160450893853394,0.0648031208996024,
-1.41177006887329));
#47408=CARTESIAN_POINT('Ctrl Pts',(-0.141353205959616,-0.0998158553618607,
-1.40382277756534));
#47409=CARTESIAN_POINT('Ctrl Pts',(0.00739153201114258,-0.172885219354373,
-1.39587548625739));
#47410=CARTESIAN_POINT('Ctrl Pts',(0.149356867178203,-0.0873868413629536,
-1.38792819494944));
#47411=CARTESIAN_POINT('Ctrl Pts',(0.154334313694721,0.0782614428250668,
-1.37998090364149));
#47412=CARTESIAN_POINT('Ctrl Pts',(0.0177586319299275,0.17212950011157,
-1.37203361233353));
#47413=CARTESIAN_POINT('Ctrl Pts',(-0.135105001901376,0.108122949820611,
-1.36408632102558));
#47414=CARTESIAN_POINT('Ctrl Pts',(-0.164052345131089,-0.0550523557504232,
-1.35613902971763));
#47415=CARTESIAN_POINT('Ctrl Pts',(-0.0425333267380425,-0.167734462568895,
-1.34819173840968));
#47416=CARTESIAN_POINT('Ctrl Pts',(0.117996623908803,-0.126573024625337,
-1.34024444710173));
#47417=CARTESIAN_POINT('Ctrl Pts',(0.170301832817638,0.0306793017462093,
-1.33229715579378));
#47418=CARTESIAN_POINT('Ctrl Pts',(0.0664087433035997,0.159793030603709,
-1.32434986448582));
#47419=CARTESIAN_POINT('Ctrl Pts',(-0.0983934540738328,0.142346977530617,
-1.31640257317788));
#47420=CARTESIAN_POINT('Ctrl Pts',(-0.172950644406985,-0.00565759806718521,
-1.30845528186992));
#47421=CARTESIAN_POINT('Ctrl Pts',(-0.0888800858747583,-0.148473109186738,
-1.30050799056197));
#47422=CARTESIAN_POINT('Ctrl Pts',(0.076709960425885,-0.15511130129085,
-1.29256069925402));
#47423=CARTESIAN_POINT('Ctrl Pts',(0.171942776317623,-0.019483723691048,
-1.28461340794607));
#47424=CARTESIAN_POINT('Ctrl Pts',(0.10947224490789,0.134014034382628,-1.27666611663812));
#47425=CARTESIAN_POINT('Ctrl Pts',(-0.0534045950907516,0.164596120974568,
-1.26871882533016));
#47426=CARTESIAN_POINT('Ctrl Pts',(-0.167299537812514,0.0442131028587772,
-1.26077153402221));
#47427=CARTESIAN_POINT('Ctrl Pts',(-0.12774984226529,-0.116721513089383,
-1.25282424271426));
#47428=CARTESIAN_POINT('Ctrl Pts',(0.0289701012791813,-0.170600899905467,
-1.24487695140631));
#47429=CARTESIAN_POINT('Ctrl Pts',(0.15911910045929,-0.0680076884308508,
-1.23692966009836));
#47430=CARTESIAN_POINT('Ctrl Pts',(0.143326436375369,0.0969611595053348,
-1.22898236879041));
#47431=CARTESIAN_POINT('Ctrl Pts',(-0.00392309526217261,0.172998679591046,
-1.22103507748245));
#47432=CARTESIAN_POINT('Ctrl Pts',(-0.147574422497777,0.0903643936577289,
-1.2130877861745));
#47433=CARTESIAN_POINT('Ctrl Pts',(-0.155872692731499,-0.0751507649815555,
-1.20514049486655));
#47434=CARTESIAN_POINT('Ctrl Pts',(-0.021206856399661,-0.171738763994403,
-1.1971932035586));
#47435=CARTESIAN_POINT('Ctrl Pts',(0.132909591999709,-0.110810532762696,
-1.18924591225065));
#47436=CARTESIAN_POINT('Ctrl Pts',(0.165123346981426,0.0517514646974669,
-1.1812986209427));
#47437=CARTESIAN_POINT('Ctrl Pts',(0.0458884334335047,0.166847791395931,
-1.17335132963475));
#47438=CARTESIAN_POINT('Ctrl Pts',(-0.115434666136934,0.128913814894044,
-1.16540403832679));
#47439=CARTESIAN_POINT('Ctrl Pts',(-0.170882813387225,-0.0272579879218593,
-1.15745674701884));
#47440=CARTESIAN_POINT('Ctrl Pts',(-0.0695997955103653,-0.158429171182573,
-1.14950945571089));
#47441=CARTESIAN_POINT('Ctrl Pts',(0.0955191156709451,-0.144291484011088,
-1.14156216440294));
#47442=CARTESIAN_POINT('Ctrl Pts',(0.173029320076704,0.00218819799715939,
-1.13361487309499));
#47443=CARTESIAN_POINT('Ctrl Pts',(0.0918396154674594,0.146660897472607,
-1.12566758178703));
#47444=CARTESIAN_POINT('Ctrl Pts',(-0.0735840132663084,0.156618411460164,
-1.11772029047909));
#47445=CARTESIAN_POINT('Ctrl Pts',(-0.171517483654975,0.0229278567979429,
-1.10977299917113));
#47446=CARTESIAN_POINT('Ctrl Pts',(-0.112137678822651,-0.131791785802262,
-1.10182570786318));
#47447=CARTESIAN_POINT('Ctrl Pts',(0.0500931307897824,-0.165633970140062,
-1.09387841655523));
#47448=CARTESIAN_POINT('Ctrl Pts',(0.166379268741419,-0.0475591500108228,
-1.08593112524728));
#47449=CARTESIAN_POINT('Ctrl Pts',(0.130064825476295,0.114136212441549,
-1.07798383393933));
#47450=CARTESIAN_POINT('Ctrl Pts',(-0.0255431338240911,0.171147544917028,
-1.07003654263137));
#47451=CARTESIAN_POINT('Ctrl Pts',(-0.157723312144672,0.0711849044587089,
-1.06208925132342));
#47452=CARTESIAN_POINT('Ctrl Pts',(-0.145242023404015,-0.0940674675655127,
-1.05414196001547));
#47453=CARTESIAN_POINT('Ctrl Pts',(0.000453080712868733,-0.173042562783117,
-1.04619466870752));
#47454=CARTESIAN_POINT('Ctrl Pts',(0.145732625964489,-0.0933056029731116,
-1.03824737739957));
#47455=CARTESIAN_POINT('Ctrl Pts',(0.157348382496199,0.0720098628141407,
-1.03030008609162));
#47456=CARTESIAN_POINT('Ctrl Pts',(0.024646551842481,0.171278957548664,
-1.02235279478366));
#47457=CARTESIAN_POINT('Ctrl Pts',(-0.130660728183639,0.11345354964567,
-1.01440550347571));
#47458=CARTESIAN_POINT('Ctrl Pts',(-0.166127939108261,-0.0484297601101159,
-1.00645821216776));
#47459=CARTESIAN_POINT('Ctrl Pts',(-0.0492250846032552,-0.165894016958069,
-0.998510920859811));
#47460=CARTESIAN_POINT('Ctrl Pts',(0.112826282560356,-0.131202758280047,
-0.990563629551857));
#47461=CARTESIAN_POINT('Ctrl Pts',(0.171395067876608,0.0238257114112947,
-0.982616338243905));
#47462=CARTESIAN_POINT('Ctrl Pts',(0.0727628558960999,0.157001594318417,
-0.974669046935956));
#47463=CARTESIAN_POINT('Ctrl Pts',(-0.0926063611495833,0.146177958979164,
-0.966721755628002));
#47464=CARTESIAN_POINT('Ctrl Pts',(-0.173038406378754,0.00128208212784741,
-0.958774464320052));
#47465=CARTESIAN_POINT('Ctrl Pts',(-0.0947622087723417,-0.144789701309411,
-0.9508271730121));
#47466=CARTESIAN_POINT('Ctrl Pts',(0.0704284719029783,-0.158062532442362,
-0.942879881704148));
#47467=CARTESIAN_POINT('Ctrl Pts',(0.171023209658835,-0.0263627687216561,
-0.934932590396196));
#47468=CARTESIAN_POINT('Ctrl Pts',(0.114758012923362,0.129516532869604,
-0.926985299088245));
#47469=CARTESIAN_POINT('Ctrl Pts',(-0.0467615199073322,0.16660520421835,
-0.919038007780294));
#47470=CARTESIAN_POINT('Ctrl Pts',(-0.16539208483705,0.050886069704146,
-0.911090716472341));
#47471=CARTESIAN_POINT('Ctrl Pts',(-0.132327498888257,-0.111505008204384,
-0.90314342516439));
#47472=CARTESIAN_POINT('Ctrl Pts',(0.0221058933671197,-0.17162535737799,
-0.895196133856439));
#47473=CARTESIAN_POINT('Ctrl Pts',(0.156264090271199,-0.0743334911624345,
-0.887248842548486));
#47474=CARTESIAN_POINT('Ctrl Pts',(0.147099196629942,0.0911359433347066,
-0.879301551240536));
#47475=CARTESIAN_POINT('Ctrl Pts',(0.00301711605757047,0.173016851281536,
-0.871354259932582));
#47476=CARTESIAN_POINT('Ctrl Pts',(-0.143832218316713,0.096209286406122,
-0.863406968624633));
#47477=CARTESIAN_POINT('Ctrl Pts',(-0.158760789492189,-0.0688399995387715,
-0.85545967731668));
#47478=CARTESIAN_POINT('Ctrl Pts',(-0.0280763348730118,-0.170750265700466,
-0.84751238600873));
#47479=CARTESIAN_POINT('Ctrl Pts',(0.128359314906885,-0.116050937494345,
-0.839565094700776));
#47480=CARTESIAN_POINT('Ctrl Pts',(0.167065717482201,0.0450885779198969,
-0.831617803392827));
#47481=CARTESIAN_POINT('Ctrl Pts',(0.0525419383045171,0.164873522846713,
-0.823670512084872));
#47482=CARTESIAN_POINT('Ctrl Pts',(-0.110172522225335,0.133438934210332,
-0.815723220776924));
#47483=CARTESIAN_POINT('Ctrl Pts',(-0.171838390265988,-0.0203838526161073,
-0.80777592946897));
#47484=CARTESIAN_POINT('Ctrl Pts',(-0.0758966523332277,-0.155510874157695,
-0.79982863816102));
#47485=CARTESIAN_POINT('Ctrl Pts',(0.0896563619686924,-0.148005643727598,
-0.791881346853067));
#47486=CARTESIAN_POINT('Ctrl Pts',(0.172977899658784,-0.00475184662183322,
-0.783934055545116));
#47487=CARTESIAN_POINT('Ctrl Pts',(0.0976466903734667,0.142860273259537,
-0.775986764237163));
#47488=CARTESIAN_POINT('Ctrl Pts',(-0.0672446054394721,0.159443083437229,
-0.768039472929214));
#47489=CARTESIAN_POINT('Ctrl Pts',(-0.170460153117567,0.0297870780006496,
-0.76009218162126));
#47490=CARTESIAN_POINT('Ctrl Pts',(-0.117332193357448,-0.12718919065161,
-0.75214489031331));
#47491=CARTESIAN_POINT('Ctrl Pts',(0.0434111023590466,-0.167509432596059,
-0.744197599005357));
#47492=CARTESIAN_POINT('Ctrl Pts',(0.16433838312751,-0.0541925239098243,
-0.736250307697407));
#47493=CARTESIAN_POINT('Ctrl Pts',(0.134536952493496,0.108828958602222,
-0.728303016389454));
#47494=CARTESIAN_POINT('Ctrl Pts',(-0.0186597623062839,0.172034145120539,
-0.720355725081503));
#47495=CARTESIAN_POINT('Ctrl Pts',(-0.154742021712401,0.0774521822354978,
-0.712408433773552));
#47496=CARTESIAN_POINT('Ctrl Pts',(-0.148897209130542,-0.0881677658207174,
-0.704461142465599));
#47497=CARTESIAN_POINT('Ctrl Pts',(-0.00648609939667713,-0.172921555427013,
-0.696513851157649));
#47498=CARTESIAN_POINT('Ctrl Pts',(0.141873963865172,-0.0990742761460573,
-0.688566559849696));
#47499=CARTESIAN_POINT('Ctrl Pts',(0.160109345674077,0.0656424500190254,
-0.680619268541746));
#47500=CARTESIAN_POINT('Ctrl Pts',(0.0314948260924915,0.170152901080425,
-0.672671977233793));
#47501=CARTESIAN_POINT('Ctrl Pts',(-0.126006277757622,0.118601651684748,
-0.664724685925842));
#47502=CARTESIAN_POINT('Ctrl Pts',(-0.167936304945184,-0.0417292618918592,
-0.65677739461789));
#47503=CARTESIAN_POINT('Ctrl Pts',(-0.0558376605567283,-0.163786719486755,
-0.648830103309939));
#47504=CARTESIAN_POINT('Ctrl Pts',(0.107474452427893,-0.135621443334034,
-0.640882812001987));
#47505=CARTESIAN_POINT('Ctrl Pts',(0.172212602258851,0.0169337957917512,
-0.632935520694036));
#47506=CARTESIAN_POINT('Ctrl Pts',(0.0789999244635886,0.153957610242003,
-0.624988229386083));
#47507=CARTESIAN_POINT('Ctrl Pts',(-0.0866703045663745,0.149773803193526,
-0.617040938078132));
#47508=CARTESIAN_POINT('Ctrl Pts',(-0.172847824251535,0.00821970000618283,
-0.609093646770181));
#47509=CARTESIAN_POINT('Ctrl Pts',(-0.100491900182772,-0.140873389305209,
-0.601146355462228));
#47510=CARTESIAN_POINT('Ctrl Pts',(0.0640336943712063,-0.160759509211294,
-0.593199064154279));
#47511=CARTESIAN_POINT('Ctrl Pts',(0.169828540482666,-0.0331994074376132,
-0.585251772846325));
#47512=CARTESIAN_POINT('Ctrl Pts',(0.119859184834551,0.12481069516463,-0.577304481538374));
#47513=CARTESIAN_POINT('Ctrl Pts',(-0.0400432256242976,0.16834629160835,
-0.569357190230424));
#47514=CARTESIAN_POINT('Ctrl Pts',(-0.163218587393212,0.0574771828297637,
-0.56140989892247));
#47515=CARTESIAN_POINT('Ctrl Pts',(-0.136692297688386,-0.106109139895445,
-0.55346260761452));
#47516=CARTESIAN_POINT('Ctrl Pts',(0.0152061266152587,-0.172373743737386,
-0.545515316306566));
#47517=CARTESIAN_POINT('Ctrl Pts',(0.153157718617635,-0.0805397233948725,
-0.537568024998617));
#47518=CARTESIAN_POINT('Ctrl Pts',(0.150635337776628,0.0851641287726385,
-0.529620733690664));
#47519=CARTESIAN_POINT('Ctrl Pts',(0.00995247414000182,0.172756713545882,
-0.521673442382713));
#47520=CARTESIAN_POINT('Ctrl Pts',(-0.139858650185577,0.101899419944128,
-0.513726151074762));
#47521=CARTESIAN_POINT('Ctrl Pts',(-0.161393508676135,-0.0624185002534306,
-0.505778859766809));
#47522=CARTESIAN_POINT('Ctrl Pts',(-0.034900650643503,-0.16948710393815,
-0.497831568458858));
#47523=CARTESIAN_POINT('Ctrl Pts',(0.123602563086265,-0.121104666364214,
-0.489884277150907));
#47524=CARTESIAN_POINT('Ctrl Pts',(0.168739351362149,0.0383531630841987,
-0.481936985842954));
#47525=CARTESIAN_POINT('Ctrl Pts',(0.0591109258779971,0.16263404397151,
-0.473989694535003));
#47526=CARTESIAN_POINT('Ctrl Pts',(-0.104733158284532,0.13774940788413,
-0.466042403227052));
#47527=CARTESIAN_POINT('Ctrl Pts',(-0.17251755335367,-0.0134769284907569,
-0.4580951119191));
#47528=CARTESIAN_POINT('Ctrl Pts',(-0.0820714242054011,-0.152342427266925,
-0.450147820611148));
#47529=CARTESIAN_POINT('Ctrl Pts',(0.083649389882709,-0.151481726254132,
-0.442200529303197));
#47530=CARTESIAN_POINT('Ctrl Pts',(0.172648232471067,-0.0116842475708879,
-0.434253237995245));
#47531=CARTESIAN_POINT('Ctrl Pts',(0.103296693906605,0.138829848536424,
-0.426305946687294));
#47532=CARTESIAN_POINT('Ctrl Pts',(-0.0607970300704926,0.162011280321123,
-0.418358655379342));
#47533=CARTESIAN_POINT('Ctrl Pts',(-0.169128625777697,0.0365983846532847,
-0.410411364071391));
#47534=CARTESIAN_POINT('Ctrl Pts',(-0.122337971042862,-0.122382002997978,
-0.402464072763438));
#47535=CARTESIAN_POINT('Ctrl Pts',(0.0366592442042335,-0.169115444685149,
-0.394516781455488));
#47536=CARTESIAN_POINT('Ctrl Pts',(0.162033147996417,-0.0607387254315766,
-0.386569490147535));
#47537=CARTESIAN_POINT('Ctrl Pts',(0.138792667630779,0.103346645947574,
-0.378622198839585));
#47538=CARTESIAN_POINT('Ctrl Pts',(-0.0117463752859325,0.172644016647908,
-0.370674907531632));
#47539=CARTESIAN_POINT('Ctrl Pts',(-0.151511818165916,0.0835948728854811,
-0.362727616223682));
#47540=CARTESIAN_POINT('Ctrl Pts',(-0.152312883523237,-0.0821262402007903,
-0.354780324915729));
#47541=CARTESIAN_POINT('Ctrl Pts',(-0.0134148461722152,-0.172522391934662,
-0.346833033607778));
#47542=CARTESIAN_POINT('Ctrl Pts',(0.137787087801864,-0.104683581576881,
-0.338885742299826));
#47543=CARTESIAN_POINT('Ctrl Pts',(0.162612762030453,0.0591694468582298,
-0.330938450991874));
#47544=CARTESIAN_POINT('Ctrl Pts',(0.0382924387629439,0.168753142045614,
-0.322991159683923));
#47545=CARTESIAN_POINT('Ctrl Pts',(-0.121149137624835,0.123558974863995,
-0.315043868375971));
#47546=CARTESIAN_POINT('Ctrl Pts',(-0.169474533761859,-0.0349616393048283,
-0.30709657706802));
#47547=CARTESIAN_POINT('Ctrl Pts',(-0.0623604178182606,-0.161415959886906,
-0.299149285760068));
#47548=CARTESIAN_POINT('Ctrl Pts',(0.101949742295844,-0.139821972030507,
-0.291201994452117));
#47549=CARTESIAN_POINT('Ctrl Pts',(0.172753120904425,0.0100146410047549,
-0.283254703144165));
#47550=CARTESIAN_POINT('Ctrl Pts',(0.0851099162552044,0.150665974830759,
-0.275307411836213));
#47551=CARTESIAN_POINT('Ctrl Pts',(-0.0805948328768723,0.153128726012732,
-0.267360120528262));
#47552=CARTESIAN_POINT('Ctrl Pts',(-0.172379204589526,0.0151440959352495,
-0.25941282922031));
#47553=CARTESIAN_POINT('Ctrl Pts',(-0.106059943506291,-0.136730472829133,
-0.251465537912358));
#47554=CARTESIAN_POINT('Ctrl Pts',(0.0575359142677703,-0.163197893327065,
-0.243518246604407));
#47555=CARTESIAN_POINT('Ctrl Pts',(0.168360690494893,-0.0399826426369145,
-0.235570955296455));
#47556=CARTESIAN_POINT('Ctrl Pts',(0.124767555060224,0.119904090926243,
-0.227623663988504));
#47557=CARTESIAN_POINT('Ctrl Pts',(-0.0332605190813962,0.169816582492104,
-0.219676372680552));
#47558=CARTESIAN_POINT('Ctrl Pts',(-0.160782541691814,0.0639758399692923,
-0.2117290813726));
#47559=CARTESIAN_POINT('Ctrl Pts',(-0.140837217604386,-0.100542587765356,
-0.203781790064649));
#47560=CARTESIAN_POINT('Ctrl Pts',(0.00828189979977818,-0.172844855191089,
-0.195834498756697));
#47561=CARTESIAN_POINT('Ctrl Pts',(0.149804982252761,-0.0866164019074298,
-0.187887207448745));
#47562=CARTESIAN_POINT('Ctrl Pts',(0.153929171798746,0.0790553217538663,
-0.179939916140794));
#47563=CARTESIAN_POINT('Ctrl Pts',(0.0168718227829098,0.172218685093424,
-0.171992624832842));
#47564=CARTESIAN_POINT('Ctrl Pts',(-0.135660109471302,0.107425640809655,
-0.164045333524891));
#47565=CARTESIAN_POINT('Ctrl Pts',(-0.163766616112805,-0.0558965956091489,
-0.156098042216939));
#47566=CARTESIAN_POINT('Ctrl Pts',(-0.0416688249318735,-0.167951312367441,
-0.148150750908988));
#47567=CARTESIAN_POINT('Ctrl Pts',(0.118646985438833,-0.125963586729395,
-0.140203459601036));
#47568=CARTESIAN_POINT('Ctrl Pts',(0.170141561514371,0.031556048159871,
-0.132256168293084));
#47569=CARTESIAN_POINT('Ctrl Pts',(0.0655848199080706,0.160132969283019,
-0.124308876985133));
#47570=CARTESIAN_POINT('Ctrl Pts',(-0.099125305718535,0.141838279147541,
-0.116361585677181));
#47571=CARTESIAN_POINT('Ctrl Pts',(-0.172919244685382,-0.0065482820045211,
-0.108414294369229));
#47572=CARTESIAN_POINT('Ctrl Pts',(-0.0881141130721895,-0.1489290103099,
-0.100467003061277));
#47573=CARTESIAN_POINT('Ctrl Pts',(0.0775077376916343,-0.15471398227649,
-0.0925197117533261));
#47574=CARTESIAN_POINT('Ctrl Pts',(0.172041084822943,-0.0185981531198262,
-0.0845724204453744));
#47575=CARTESIAN_POINT('Ctrl Pts',(0.108780089674747,0.134576675006324,
-0.076625129137423));
#47576=CARTESIAN_POINT('Ctrl Pts',(-0.0542508082392599,0.164317791962513,
-0.0686778378294712));
#47577=CARTESIAN_POINT('Ctrl Pts',(-0.167526657386005,0.0433528683734585,
-0.06073054652152));
#47578=CARTESIAN_POINT('Ctrl Pts',(-0.127143896441013,-0.117381842937533,
-0.0527832552135681));
#47579=CARTESIAN_POINT('Ctrl Pts',(0.0298426026130803,-0.170442044130026,
-0.0448359639056166));
#47580=CARTESIAN_POINT('Ctrl Pts',(0.159478309507775,-0.0672012331938912,
-0.0368886725976649));
#47581=CARTESIAN_POINT('Ctrl Pts',(0.142804160215386,0.0977247079951531,
-0.0289413812897132));
#47582=CARTESIAN_POINT('Ctrl Pts',(-0.00477418028139723,0.172925445239909,
-0.0209940899817616));
#47583=CARTESIAN_POINT('Ctrl Pts',(-0.148114672239004,0.0897012229138564,
-0.01304679867381));
#47584=CARTESIAN_POINT('Ctrl Pts',(-0.155329206692728,-0.0761542535693343,
-0.00509950736585855));
#47585=CARTESIAN_POINT('Ctrl Pts',(-0.0655693004694094,-0.139615734371339,
0.000198686839442543));
#47586=CARTESIAN_POINT('Ctrl Pts',(-0.0171871968558861,-0.145337272453549,
0.00284778394209306));
#47587=CARTESIAN_POINT('Ctrl Pts',(-0.146319403921505,0.000134192518820611,
-0.0587155045842896));
#47588=CARTESIAN_POINT('Ctrl Pts',(-0.145990313106502,-0.0362412802340569,
-0.0567380881273823));
#47589=CARTESIAN_POINT('Ctrl Pts',(-0.132264295006575,-0.0728382504267649,
-0.0547606716704749));
#47590=CARTESIAN_POINT('Ctrl Pts',(-0.107709940089491,-0.0994360912511227,
-0.0527832552135677));
#47591=CARTESIAN_POINT('Ctrl Pts',(-0.0748150634229754,-0.135068576668367,
-0.0501341581109172));
#47592=CARTESIAN_POINT('Ctrl Pts',(-0.0224862304049495,-0.152755310399195,
-0.047485061008267));
#47593=CARTESIAN_POINT('Ctrl Pts',(0.0252841372531801,-0.144391875441922,
-0.0448359639056166));
#47594=CARTESIAN_POINT('Ctrl Pts',(0.0730545049113125,-0.136028440484648,
-0.042186866802966));
#47595=CARTESIAN_POINT('Ctrl Pts',(0.116266407209548,-0.101614836839265,
-0.0395377697003152));
#47596=CARTESIAN_POINT('Ctrl Pts',(0.135093333476596,-0.0569203781517345,
-0.0368886725976646));
#47597=CARTESIAN_POINT('Ctrl Pts',(0.153920259743645,-0.0122259194642038,
-0.0342395754950141));
#47598=CARTESIAN_POINT('Ctrl Pts',(0.148362209979515,0.0427493942654739,
-0.0315904783923637));
#47599=CARTESIAN_POINT('Ctrl Pts',(0.120986795014652,0.0827705073377738,
-0.0289413812897131));
#47600=CARTESIAN_POINT('Ctrl Pts',(0.093611380049789,0.122791620410074,
-0.0262922841870625));
#47601=CARTESIAN_POINT('Ctrl Pts',(0.0444185998841973,0.147858532824991,
-0.0236431870844121));
#47602=CARTESIAN_POINT('Ctrl Pts',(-0.00406787219153488,0.146521285311441,
-0.0209940899817616));
#47603=CARTESIAN_POINT('Ctrl Pts',(-0.0488742093476865,0.145285535206551,
-0.0185460599878418));
#47604=CARTESIAN_POINT('Ctrl Pts',(-0.0930773873900169,0.12150167906643,
-0.0160980299939217));
#47605=CARTESIAN_POINT('Ctrl Pts',(-0.119330942213657,0.085138415363241,
-0.013650000000002));
#47606=CARTESIAN_POINT('',(-0.000893209148009567,0.117964196654764,-2.93765));
#47607=CARTESIAN_POINT('Ctrl Pts',(-0.0008932091480129,0.117964196654764,
-2.93765));
#47608=CARTESIAN_POINT('Ctrl Pts',(0.00208421411728759,0.118354195981894,
-2.93765));
#47609=CARTESIAN_POINT('Ctrl Pts',(0.00507143193442542,0.118622138849448,
-2.93765));
#47610=CARTESIAN_POINT('Ctrl Pts',(0.00806195760498323,0.118765052615256,
-2.93765));
#47611=CARTESIAN_POINT('Ctrl Pts',(0.0152384124430961,0.119108007098531,
-2.93765));
#47612=CARTESIAN_POINT('Ctrl Pts',(0.0224335537438771,0.118732751163502,
-2.93765));
#47613=CARTESIAN_POINT('Ctrl Pts',(0.0295711880776548,0.117700942165764,
-2.93765));
#47614=CARTESIAN_POINT('Ctrl Pts',(0.0334765121796589,0.117136392574247,
-2.93765));
#47615=CARTESIAN_POINT('Ctrl Pts',(0.0373569563325073,0.116375728419311,
-2.93765));
#47616=CARTESIAN_POINT('Ctrl Pts',(0.0411928145026145,0.115431075471498,
-2.93765));
#47617=CARTESIAN_POINT('Ctrl Pts',(0.0481018456958536,0.113729595282767,
-2.93765));
#47618=CARTESIAN_POINT('Ctrl Pts',(0.0548737925559738,0.111431279199373,
-2.93765));
#47619=CARTESIAN_POINT('Ctrl Pts',(0.0614384215502389,0.10858518186639,
-2.93765));
#47620=CARTESIAN_POINT('Ctrl Pts',(0.0646734046575246,0.107182653741505,
-2.93765));
#47621=CARTESIAN_POINT('Ctrl Pts',(0.0678508377690415,0.105649735926586,
-2.93765));
#47622=CARTESIAN_POINT('Ctrl Pts',(0.0709571867534955,0.103995938706946,
-2.93765));
#47623=CARTESIAN_POINT('Ctrl Pts',(0.0793412397536873,0.099532330911938,
-2.93765));
#47624=CARTESIAN_POINT('Ctrl Pts',(0.0872211356366982,0.0941863465303336,
-2.93765));
#47625=CARTESIAN_POINT('Ctrl Pts',(0.0944378463806949,0.0880609267163502,
-2.93765));
#47626=CARTESIAN_POINT('Ctrl Pts',(0.0970752818418381,0.0858223169112907,
-2.93765));
#47627=CARTESIAN_POINT('Ctrl Pts',(0.0996240141760927,0.0834791156530963,
-2.93765));
#47628=CARTESIAN_POINT('Ctrl Pts',(0.102075530811344,0.0810347775427261,
-2.93765));
#47629=CARTESIAN_POINT('Ctrl Pts',(0.104250398830597,0.0788662779665695,
-2.93765));
#47630=CARTESIAN_POINT('Ctrl Pts',(0.106344685942108,0.0766219445137936,
-2.93765));
#47631=CARTESIAN_POINT('Ctrl Pts',(0.108348175066807,0.0743108418799378,
-2.93765));
#47632=CARTESIAN_POINT('Ctrl Pts',(0.111175899843332,0.0710489513618998,
-2.93765));
#47633=CARTESIAN_POINT('Ctrl Pts',(0.113826045040914,0.0676509280277566,
-2.93765));
#47634=CARTESIAN_POINT('Ctrl Pts',(0.116284186664136,0.0641259479802579,
-2.93765));
#47635=CARTESIAN_POINT('Ctrl Pts',(0.120002164263989,0.0587943606002954,
-2.93765));
#47636=CARTESIAN_POINT('Ctrl Pts',(0.123281449454453,0.0531727090630523,
-2.93765));
#47637=CARTESIAN_POINT('Ctrl Pts',(0.126128015808201,0.047316382515659,
-2.93765));
#47638=CARTESIAN_POINT('Ctrl Pts',(0.127562547730943,0.0443650768588713,
-2.93765));
#47639=CARTESIAN_POINT('Ctrl Pts',(0.128887043644863,0.0413540347815275,
-2.93765));
#47640=CARTESIAN_POINT('Ctrl Pts',(0.130101371942864,0.0382896759029232,
-2.93765));
#47641=CARTESIAN_POINT('Ctrl Pts',(0.131334954033748,0.0351767300554848,
-2.93765));
#47642=CARTESIAN_POINT('Ctrl Pts',(0.132451910687336,0.0320157007800445,
-2.93765));
#47643=CARTESIAN_POINT('Ctrl Pts',(0.133451273547085,0.0288208664690228,
-2.93765));
#47644=CARTESIAN_POINT('Ctrl Pts',(0.13594044569831,0.0208633037907661,
-2.93765));
#47645=CARTESIAN_POINT('Ctrl Pts',(0.137706627804123,0.0126846288520797,
-2.93765));
#47646=CARTESIAN_POINT('Ctrl Pts',(0.138759382734113,0.00439393427432196,
-2.93765));
#47647=CARTESIAN_POINT('Ctrl Pts',(0.139457649115666,-0.00110507897032189,
-2.93765));
#47648=CARTESIAN_POINT('Ctrl Pts',(0.139841620680567,-0.00665378048569686,
-2.93765));
#47649=CARTESIAN_POINT('Ctrl Pts',(0.13990842161102,-0.0122228021535617,
-2.93765));
#47650=CARTESIAN_POINT('Ctrl Pts',(0.139946458473856,-0.0153938375250784,
-2.93765));
#47651=CARTESIAN_POINT('Ctrl Pts',(0.139881269861857,-0.0185709804508514,
-2.93765));
#47652=CARTESIAN_POINT('Ctrl Pts',(0.139713346423489,-0.0217351033015259,
-2.93765));
#47653=CARTESIAN_POINT('Ctrl Pts',(0.139165794893991,-0.0320524260245424,
-2.93765));
#47654=CARTESIAN_POINT('Ctrl Pts',(0.137530845631308,-0.0422672851557336,
-2.93765));
#47655=CARTESIAN_POINT('Ctrl Pts',(0.134806053950555,-0.0521934162937557,
-2.93765));
#47656=CARTESIAN_POINT('Ctrl Pts',(0.133196241206826,-0.0580577957671597,
-2.93765));
#47657=CARTESIAN_POINT('Ctrl Pts',(0.131205098375125,-0.0638217359559869,
-2.93765));
#47658=CARTESIAN_POINT('Ctrl Pts',(0.128823493644037,-0.0694465980833095,
-2.93765));
#47659=CARTESIAN_POINT('Ctrl Pts',(-0.000893209148009566,0.117964196654764,
-2.93765));
#47660=CARTESIAN_POINT('Ctrl Pts',(-0.0369831781664475,0.117488069255602,
-2.93520197000608));
#47661=CARTESIAN_POINT('Ctrl Pts',(-0.0981247360162019,0.0868112407524339,
-2.93105639951488));
#47662=CARTESIAN_POINT('Ctrl Pts',(-0.117478474975439,0.0250944040704393,
-2.92691082902367));
#47663=CARTESIAN_POINT('Ctrl Pts',(-0.117640397146581,-8.56657636452585E-5,
-2.92521328852638));
#47664=CARTESIAN_POINT('Origin',(-3.28582941601228E-18,0.,-2.93765));
#47665=CARTESIAN_POINT('',(-0.111717694016329,0.0372841450039274,-2.93765));
#47666=CARTESIAN_POINT('Ctrl Pts',(0.0262268935511073,-0.144224038131951,
-2.93765));
#47667=CARTESIAN_POINT('Ctrl Pts',(0.0225529367225777,-0.144559449307367,
-2.93765));
#47668=CARTESIAN_POINT('Ctrl Pts',(0.018871621332308,-0.144745852633568,
-2.93765));
#47669=CARTESIAN_POINT('Ctrl Pts',(0.0151894836933861,-0.144777913300572,
-2.93765));
#47670=CARTESIAN_POINT('Ctrl Pts',(0.00801195125766715,-0.144840408649714,
-2.93765));
#47671=CARTESIAN_POINT('Ctrl Pts',(0.000830984588550291,-0.144317119643943,
-2.93765));
#47672=CARTESIAN_POINT('Ctrl Pts',(-0.0062939751165674,-0.143238551230609,
-2.93765));
#47673=CARTESIAN_POINT('Ctrl Pts',(-0.0109733672327204,-0.142530190097499,
-2.93765));
#47674=CARTESIAN_POINT('Ctrl Pts',(-0.0156307259998283,-0.141580965612318,
-2.93765));
#47675=CARTESIAN_POINT('Ctrl Pts',(-0.0202259413021322,-0.140404321648008,
-2.93765));
#47676=CARTESIAN_POINT('Ctrl Pts',(-0.0264890284927663,-0.138800604900045,
-2.93765));
#47677=CARTESIAN_POINT('Ctrl Pts',(-0.0326462411610736,-0.136773775845124,
-2.93765));
#47678=CARTESIAN_POINT('Ctrl Pts',(-0.0386527104818304,-0.13434452281258,
-2.93765));
#47679=CARTESIAN_POINT('Ctrl Pts',(-0.0417103306569216,-0.1331079006497,
-2.93765));
#47680=CARTESIAN_POINT('Ctrl Pts',(-0.0447288163869714,-0.131766884032008,
-2.93765));
#47681=CARTESIAN_POINT('Ctrl Pts',(-0.0477016792219733,-0.130323591521167,
-2.93765));
#47682=CARTESIAN_POINT('Ctrl Pts',(-0.0508144489056172,-0.128812375759888,
-2.93765));
#47683=CARTESIAN_POINT('Ctrl Pts',(-0.0538686917803179,-0.127193116028306,
-2.93765));
#47684=CARTESIAN_POINT('Ctrl Pts',(-0.0568558823257219,-0.125470616735044,
-2.93765));
#47685=CARTESIAN_POINT('Ctrl Pts',(-0.0653824269832697,-0.120553967822511,
-2.93765));
#47686=CARTESIAN_POINT('Ctrl Pts',(-0.0733713052120728,-0.114795730576438,
-2.93765));
#47687=CARTESIAN_POINT('Ctrl Pts',(-0.080650133064915,-0.108259608267344,
-2.93765));
#47688=CARTESIAN_POINT('Ctrl Pts',(-0.0835973555190745,-0.105613109844528,
-2.93765));
#47689=CARTESIAN_POINT('Ctrl Pts',(-0.0864276939354442,-0.102838727361706,
-2.93765));
#47690=CARTESIAN_POINT('Ctrl Pts',(-0.0891274150692409,-0.0999395069146105,
-2.93765));
#47691=CARTESIAN_POINT('Ctrl Pts',(-0.0911100509910371,-0.097810361599689,
-2.93765));
#47692=CARTESIAN_POINT('Ctrl Pts',(-0.0930196844243488,-0.0956163133794605,
-2.93765));
#47693=CARTESIAN_POINT('Ctrl Pts',(-0.0948462221025146,-0.0933654881788209,
-2.93765));
#47694=CARTESIAN_POINT('Ctrl Pts',(-0.0976832640047863,-0.0898694281274804,
-2.93765));
#47695=CARTESIAN_POINT('Ctrl Pts',(-0.100324145957716,-0.086232035159791,
-2.93765));
#47696=CARTESIAN_POINT('Ctrl Pts',(-0.102751026356172,-0.0824594073302338,
-2.93765));
#47697=CARTESIAN_POINT('Ctrl Pts',(-0.106748435662813,-0.0762453649711815,
-2.93765));
#47698=CARTESIAN_POINT('Ctrl Pts',(-0.110166211331277,-0.0696643617856752,
-2.93765));
#47699=CARTESIAN_POINT('Ctrl Pts',(-0.112992526824757,-0.0628009944060238,
-2.93765));
#47700=CARTESIAN_POINT('Ctrl Pts',(-0.114133115052098,-0.0600312130241466,
-2.93765));
#47701=CARTESIAN_POINT('Ctrl Pts',(-0.115177892243825,-0.0572131827636228,
-2.93765));
#47702=CARTESIAN_POINT('Ctrl Pts',(-0.116122837122688,-0.0543598758198917,
-2.93765));
#47703=CARTESIAN_POINT('Ctrl Pts',(-0.119054866830036,-0.0455064697532169,
-2.93765));
#47704=CARTESIAN_POINT('Ctrl Pts',(-0.121016207235663,-0.0363600245602272,
-2.93765));
#47705=CARTESIAN_POINT('Ctrl Pts',(-0.121991070818189,-0.027094190560155,
-2.93765));
#47706=CARTESIAN_POINT('Ctrl Pts',(-0.122559674353073,-0.0216897564828892,
-2.93765));
#47707=CARTESIAN_POINT('Ctrl Pts',(-0.122791706067432,-0.0162445702826281,
-2.93765));
#47708=CARTESIAN_POINT('Ctrl Pts',(-0.122676027364733,-0.0107949329128276,
-2.93765));
#47709=CARTESIAN_POINT('Ctrl Pts',(-0.122612206719513,-0.00778833476608035,
-2.93765));
#47710=CARTESIAN_POINT('Ctrl Pts',(-0.122442102964897,-0.00478029932637062,
-2.93765));
#47711=CARTESIAN_POINT('Ctrl Pts',(-0.12216540228983,-0.00179153671437861,
-2.93765));
#47712=CARTESIAN_POINT('Ctrl Pts',(-0.121359044251975,0.00691828213531097,
-2.93765));
#47713=CARTESIAN_POINT('Ctrl Pts',(-0.119650749016099,0.0154971799534183,
-2.93765));
#47714=CARTESIAN_POINT('Ctrl Pts',(-0.117001838809494,0.0237911387571977,
-2.93765));
#47715=CARTESIAN_POINT('Ctrl Pts',(-0.115534100011671,0.0283867513579932,
-2.93765));
#47716=CARTESIAN_POINT('Ctrl Pts',(-0.113776792745658,0.0328945535045048,
-2.93765));
#47717=CARTESIAN_POINT('Ctrl Pts',(-0.111717694016322,0.037284145003949,
-2.93765));
#47718=CARTESIAN_POINT('Origin',(0.,0.,-2.93765));
#47719=CARTESIAN_POINT('Origin',(0.,0.,-3.06008671147362));
#47720=CARTESIAN_POINT('Ctrl Pts',(-0.111717694016322,0.037284145003949,
-2.93765));
#47721=CARTESIAN_POINT('Ctrl Pts',(-0.115720921699064,0.0252889292013365,
-2.93679557049121));
#47722=CARTESIAN_POINT('Ctrl Pts',(-0.11762911624172,0.0126318964897331,
-2.93594114098241));
#47723=CARTESIAN_POINT('Ctrl Pts',(-0.117558445841294,-3.12605290917947E-5,
-2.93508671147362));
#47724=CARTESIAN_POINT('Ctrl Pts',(-0.138823048348883,0.046330160232009,
-2.95414778394209));
#47725=CARTESIAN_POINT('Ctrl Pts',(-0.15424614371138,0.000116611595973093,
-2.95149868683944));
#47726=CARTESIAN_POINT('Ctrl Pts',(-0.13504236871914,-0.108121172854393,
-2.94620049263414));
#47727=CARTESIAN_POINT('Ctrl Pts',(0.0180999205918092,-0.172211081102293,
-2.93825320132619));
#47728=CARTESIAN_POINT('Ctrl Pts',(0.15443488214358,-0.0779478857227474,
-2.93030591001824));
#47729=CARTESIAN_POINT('Ctrl Pts',(0.149227010588132,0.0876039139611851,
-2.92235861871029));
#47730=CARTESIAN_POINT('Ctrl Pts',(0.00709707033375117,0.17291318152139,
-2.91441132740233));
#47731=CARTESIAN_POINT('Ctrl Pts',(-0.141514212609231,0.0995730889212593,
-2.90646403609439));
#47732=CARTESIAN_POINT('Ctrl Pts',(-0.160345505504641,-0.0650644803652693,
-2.89851674478643));
#47733=CARTESIAN_POINT('Ctrl Pts',(-0.0321025340682361,-0.170041405975025,
-2.89056945347848));
#47734=CARTESIAN_POINT('Ctrl Pts',(0.125580313835011,-0.119050713111042,
-2.88262216217053));
#47735=CARTESIAN_POINT('Ctrl Pts',(0.168084926783387,0.0411272070241147,
-2.87467487086258));
#47736=CARTESIAN_POINT('Ctrl Pts',(0.0564234196368953,0.163586137243789,
-2.86672757955463));
#47737=CARTESIAN_POINT('Ctrl Pts',(-0.106988207737868,0.13600510865514,
-2.85878028824668));
#47738=CARTESIAN_POINT('Ctrl Pts',(-0.172272163300253,-0.0163171448586885,
-2.85083299693872));
#47739=CARTESIAN_POINT('Ctrl Pts',(-0.0795504967991995,-0.153673888715109,
-2.84288570563077));
#47740=CARTESIAN_POINT('Ctrl Pts',(0.0861336102392644,-0.150083061316343,
-2.83493841432282));
#47741=CARTESIAN_POINT('Ctrl Pts',(0.172817302014886,-0.00883838299254691,
-2.82699112301487));
#47742=CARTESIAN_POINT('Ctrl Pts',(0.100995520311121,0.140512776799912,
-2.81904383170691));
#47743=CARTESIAN_POINT('Ctrl Pts',(-0.0634578319565696,0.160987690016662,
-2.81109654039897));
#47744=CARTESIAN_POINT('Ctrl Pts',(-0.169708614925762,0.0338071110003193,
-2.80314924909101));
#47745=CARTESIAN_POINT('Ctrl Pts',(-0.120305186517372,-0.124380852578114,
-2.79520195778306));
#47746=CARTESIAN_POINT('Ctrl Pts',(0.0394403609169686,-0.168488551460744,
-2.78725466647511));
#47747=CARTESIAN_POINT('Ctrl Pts',(0.163011799154919,-0.0580610684788042,
-2.77930737516716));
#47748=CARTESIAN_POINT('Ctrl Pts',(0.137071248485045,0.105619160687613,
-2.77136008385921));
#47749=CARTESIAN_POINT('Ctrl Pts',(-0.0145890045231812,0.172427072037811,
-2.76341279255126));
#47750=CARTESIAN_POINT('Ctrl Pts',(-0.152868440543263,0.0810874475707317,
-2.7554655012433));
#47751=CARTESIAN_POINT('Ctrl Pts',(-0.150939225174926,-0.084624373309619,
-2.74751820993535));
#47752=CARTESIAN_POINT('Ctrl Pts',(-0.0105708060663173,-0.172719982367763,
-2.7395709186274));
#47753=CARTESIAN_POINT('Ctrl Pts',(0.139492998563312,-0.102399402381208,
-2.73162362731945));
#47754=CARTESIAN_POINT('Ctrl Pts',(0.16161590755552,0.0618403806498103,
-2.7236763360115));
#47755=CARTESIAN_POINT('Ctrl Pts',(0.0355071190986658,0.169361089825304,
-2.71572904470354));
#47756=CARTESIAN_POINT('Ctrl Pts',(-0.123168268870792,0.121546336011192,
-2.7077817533956));
#47757=CARTESIAN_POINT('Ctrl Pts',(-0.168875559555085,-0.0377489024866377,
-2.69983446208764));
#47758=CARTESIAN_POINT('Ctrl Pts',(-0.0596927083592543,-0.162421411220021,
-2.69188717077969));
#47759=CARTESIAN_POINT('Ctrl Pts',(0.104239403721097,-0.138123426564634,
-2.68393987947174));
#47760=CARTESIAN_POINT('Ctrl Pts',(0.172564691021556,0.0128593027283262,
-2.67599258816379));
#47761=CARTESIAN_POINT('Ctrl Pts',(0.0826162201395204,0.152047671550354,
-2.66804529685583));
#47762=CARTESIAN_POINT('Ctrl Pts',(-0.0831066143792944,0.151780186126033,
-2.66009800554788));
#47763=CARTESIAN_POINT('Ctrl Pts',(-0.172605302986316,0.0123021800927432,
-2.65215071423994));
#47764=CARTESIAN_POINT('Ctrl Pts',(-0.103792984723003,-0.138459201847778,
-2.64420342293198));
#47765=CARTESIAN_POINT('Ctrl Pts',(0.0602167094800405,-0.162227871074707,
-2.63625613162403));
#47766=CARTESIAN_POINT('Ctrl Pts',(0.168996536794456,-0.0372035590436465,
-2.62830884031608));
#47767=CARTESIAN_POINT('Ctrl Pts',(0.122775263710156,0.12194330188631,-2.62036154900813));
#47768=CARTESIAN_POINT('Ctrl Pts',(-0.0360536481919909,0.169245586961913,
-2.61241425770017));
#47769=CARTESIAN_POINT('Ctrl Pts',(-0.161814692259995,0.0613183465435701,
-2.60446696639222));
#47770=CARTESIAN_POINT('Ctrl Pts',(-0.139161716510039,-0.102849165830422,
-2.59651967508427));
#47771=CARTESIAN_POINT('Ctrl Pts',(0.0111283079130825,-0.172684958861581,
-2.58857238377632));
#47772=CARTESIAN_POINT('Ctrl Pts',(0.151211614465995,-0.0841366858428694,
-2.58062509246837));
#47773=CARTESIAN_POINT('Ctrl Pts',(0.152605885847715,0.0815804992548367,
-2.57267780116042));
#47774=CARTESIAN_POINT('Ctrl Pts',(0.014032317163657,0.172473268447759,
-2.56473050985246));
#47775=CARTESIAN_POINT('Ctrl Pts',(-0.137411483317849,0.105176130877793,
-2.55678321854451));
#47776=CARTESIAN_POINT('Ctrl Pts',(-0.162823522878765,-0.058586983634443,
-2.54883592723656));
#47777=CARTESIAN_POINT('Ctrl Pts',(-0.0388962582402102,-0.168614991471532,
-2.54088863592861));
#47778=CARTESIAN_POINT('Ctrl Pts',(0.120706073728026,-0.12399184658355,
-2.53294134462066));
#47779=CARTESIAN_POINT('Ctrl Pts',(0.169598597036642,0.0343547687699517,
-2.52499405331271));
#47780=CARTESIAN_POINT('Ctrl Pts',(0.0629378192812766,0.161191703130625,
-2.51704676200475));
#47781=CARTESIAN_POINT('Ctrl Pts',(-0.10144858664574,0.140186014001455,
-2.5090994706968));
#47782=CARTESIAN_POINT('Ctrl Pts',(-0.172787863547209,-0.0093961941670593,
-2.50115217938885));
#47783=CARTESIAN_POINT('Ctrl Pts',(-0.0856486917575374,-0.150360353332441,
-2.4932048880809));
#47784=CARTESIAN_POINT('Ctrl Pts',(0.0800461813615386,-0.153416241328843,
-2.48525759677295));
#47785=CARTESIAN_POINT('Ctrl Pts',(0.172323892039918,-0.0157610433109308,
-2.477310305465));
#47786=CARTESIAN_POINT('Ctrl Pts',(0.106548701766463,0.136349948316512,
-2.46936301415705));
#47787=CARTESIAN_POINT('Ctrl Pts',(-0.0569513669756151,0.163402803077679,
-2.46141572284909));
#47788=CARTESIAN_POINT('Ctrl Pts',(-0.168216492221969,0.0405850464896916,
-2.45346843154115));
#47789=CARTESIAN_POINT('Ctrl Pts',(-0.125195962305283,-0.119456708796486,
-2.44552114023319));
#47790=CARTESIAN_POINT('Ctrl Pts',(0.0326524350392282,-0.169934554285005,
-2.43757384892524));
#47791=CARTESIAN_POINT('Ctrl Pts',(0.160552506472577,-0.064550963737247,
-2.42962655761728));
#47792=CARTESIAN_POINT('Ctrl Pts',(0.141196216047521,0.100037806992637,
-2.42167926630934));
#47793=CARTESIAN_POINT('Ctrl Pts',(-0.00766313565102988,0.172873394731602,
-2.41373197500138));
#47794=CARTESIAN_POINT('Ctrl Pts',(-0.14949397374247,0.0871520858540961,
-2.40578468369343));
#47795=CARTESIAN_POINT('Ctrl Pts',(-0.154211171089647,-0.078503814972228,
-2.39783739238548));
#47796=CARTESIAN_POINT('Ctrl Pts',(-0.017488184714347,-0.172157188782319,
-2.38989010107753));
#47797=CARTESIAN_POINT('Ctrl Pts',(0.135274703579161,-0.107910559379536,
-2.38194280976958));
#47798=CARTESIAN_POINT('Ctrl Pts',(0.163965653425891,0.0553100239617989,
-2.37399551846162));
#47799=CARTESIAN_POINT('Ctrl Pts',(0.0422697539875444,0.16780107911413,
-2.36604822715368));
#47800=CARTESIAN_POINT('Ctrl Pts',(-0.118195332713031,0.126387489803738,
-2.35810093584572));
#47801=CARTESIAN_POINT('Ctrl Pts',(-0.170253424927118,-0.0309468181663384,
-2.35015364453777));
#47802=CARTESIAN_POINT('Ctrl Pts',(-0.0661576177127792,-0.159897166555896,
-2.34220635322982));
#47803=CARTESIAN_POINT('Ctrl Pts',(0.0986169687224061,-0.142192221074285,
-2.33425906192187));
#47804=CARTESIAN_POINT('Ctrl Pts',(0.172941543814754,0.0059293066208318,
-2.32631177061392));
#47805=CARTESIAN_POINT('Ctrl Pts',(0.088646716969042,0.148612562808953,
-2.31836447930597));
#47806=CARTESIAN_POINT('Ctrl Pts',(-0.0769535551690017,0.154990595201404,
-2.31041718799801));
#47807=CARTESIAN_POINT('Ctrl Pts',(-0.171973175436669,0.0192135677130206,
-2.30246989669006));
#47808=CARTESIAN_POINT('Ctrl Pts',(-0.10926156678474,-0.134185857219671,
-2.29452260538211));
#47809=CARTESIAN_POINT('Ctrl Pts',(0.0536631196270061,-0.164512017329835,
-2.28657531407415));
#47810=CARTESIAN_POINT('Ctrl Pts',(0.167368793917039,-0.0439502113395367,
-2.27862802276621));
#47811=CARTESIAN_POINT('Ctrl Pts',(0.127566309273023,0.116922072306703,
-2.27068073145825));
#47812=CARTESIAN_POINT('Ctrl Pts',(-0.0292380896479154,0.170555176901126,
-2.26273344015031));
#47813=CARTESIAN_POINT('Ctrl Pts',(-0.159225749273804,0.0677576196617771,
-2.25478614884235));
#47814=CARTESIAN_POINT('Ctrl Pts',(-0.143173928935275,-0.0971862146977188,
-2.2468388575344));
#47815=CARTESIAN_POINT('Ctrl Pts',(0.00419488140978216,-0.172992303944401,
-2.23889156622645));
#47816=CARTESIAN_POINT('Ctrl Pts',(0.147716209156132,-0.0901324348199692,
-2.2309442749185));
#47817=CARTESIAN_POINT('Ctrl Pts',(0.155754435294457,0.0753955578276256,
-2.22299698361055));
#47818=CARTESIAN_POINT('Ctrl Pts',(0.0209370188228705,0.17177187050517,
-2.2150496923026));
#47819=CARTESIAN_POINT('Ctrl Pts',(-0.133083518719539,0.11060158814077,
-2.20710240099464));
#47820=CARTESIAN_POINT('Ctrl Pts',(-0.165041839853626,-0.0520108195644357,
-2.19915510968669));
#47821=CARTESIAN_POINT('Ctrl Pts',(-0.0456262495787772,-0.166919680096175,
-2.19120781837874));
#47822=CARTESIAN_POINT('Ctrl Pts',(0.115637055601487,-0.12873230218501,
-2.18326052707079));
#47823=CARTESIAN_POINT('Ctrl Pts',(0.170839779866426,0.0275264212934636,
-2.17531323576284));
#47824=CARTESIAN_POINT('Ctrl Pts',(0.0693508087069927,0.15853832213607,
-2.16736594445488));
#47825=CARTESIAN_POINT('Ctrl Pts',(-0.0957456887782547,0.144141240921575,
-2.15941865314693));
#47826=CARTESIAN_POINT('Ctrl Pts',(-0.173025670016707,-0.00246003441113623,
-2.15147136183898));
#47827=CARTESIAN_POINT('Ctrl Pts',(-0.0916090900206878,-0.146805002910718,
-2.14352407053103));
#47828=CARTESIAN_POINT('Ctrl Pts',(0.0738299796018623,-0.156502614566092,
-2.13557677922308));
#47829=CARTESIAN_POINT('Ctrl Pts',(0.171553294228662,-0.022658364754064,
-2.12762948791513));
#47830=CARTESIAN_POINT('Ctrl Pts',(0.111930488710947,0.131967798916868,
-2.11968219660717));
#47831=CARTESIAN_POINT('Ctrl Pts',(-0.0503532899098111,0.165555067724588,
-2.11173490529923));
#47832=CARTESIAN_POINT('Ctrl Pts',(-0.166453782809105,0.0472977001827116,
-2.10378761399127));
#47833=CARTESIAN_POINT('Ctrl Pts',(-0.129885351301263,-0.114340411803446,
-2.09584032268332));
#47834=CARTESIAN_POINT('Ctrl Pts',(0.0258119852080813,-0.171107205206712,
-2.08789303137537));
#47835=CARTESIAN_POINT('Ctrl Pts',(0.157834954262227,-0.0709370246562046,
-2.07994574006742));
#47836=CARTESIAN_POINT('Ctrl Pts',(0.14509405977175,0.0942955358062407,
-2.07199844875947));
#47837=CARTESIAN_POINT('Ctrl Pts',(-0.000724940060565141,0.173041638676773,
-2.06405115745151));
#47838=CARTESIAN_POINT('Ctrl Pts',(-0.145879035692817,0.0930765340962364,
-2.05610386614356));
#47839=CARTESIAN_POINT('Ctrl Pts',(-0.157235057788262,-0.0722569779077145,
-2.04815657483561));
#47840=CARTESIAN_POINT('Ctrl Pts',(-0.0243774324284428,-0.171317468584586,
-2.04020928352766));
#47841=CARTESIAN_POINT('Ctrl Pts',(0.130838809995228,-0.11324813487677,
-2.03226199221971));
#47842=CARTESIAN_POINT('Ctrl Pts',(0.166051649338603,0.0486906973246862,
-2.02431470091175));
#47843=CARTESIAN_POINT('Ctrl Pts',(0.0489643950900598,0.165971148900942,
-2.01636740960381));
#47844=CARTESIAN_POINT('Ctrl Pts',(-0.113032271287723,0.131025340684818,
-2.00842011829585));
#47845=CARTESIAN_POINT('Ctrl Pts',(-0.17135742603286,-0.0240949537751543,
-2.0004728269879));
#47846=CARTESIAN_POINT('Ctrl Pts',(-0.0725161080183242,-0.157115716374617,
-1.99252553567995));
#47847=CARTESIAN_POINT('Ctrl Pts',(0.0928359015918849,-0.146032289681619,
-1.984578244372));
#47848=CARTESIAN_POINT('Ctrl Pts',(0.17304020831898,-0.00101022718139327,
-1.97663095306405));
#47849=CARTESIAN_POINT('Ctrl Pts',(0.0945346194978198,0.144938400606728,
-1.96868366175609));
#47850=CARTESIAN_POINT('Ctrl Pts',(-0.0706767109076062,0.157951691315151,
-1.96073637044814));
#47851=CARTESIAN_POINT('Ctrl Pts',(-0.171064417284779,0.0260940489969148,
-1.95278907914019));
#47852=CARTESIAN_POINT('Ctrl Pts',(-0.114554394151342,-0.129696665472376,
-1.94484178783224));
#47853=CARTESIAN_POINT('Ctrl Pts',(0.0470232089796812,-0.166531534765303,
-1.93689449652429));
#47854=CARTESIAN_POINT('Ctrl Pts',(0.165471826899637,-0.0506261667177226,
-1.92894720521634));
#47855=CARTESIAN_POINT('Ctrl Pts',(0.132152155711843,0.111712765585439,
-1.92099991390838));
#47856=CARTESIAN_POINT('Ctrl Pts',(-0.0223754996390369,0.171590417185628,
-1.91305262260043));
#47857=CARTESIAN_POINT('Ctrl Pts',(-0.156380680791286,0.0740879000194224,
-1.90510533129248));
#47858=CARTESIAN_POINT('Ctrl Pts',(-0.146955836313892,-0.0913669328987178,
-1.89715803998453));
#47859=CARTESIAN_POINT('Ctrl Pts',(-0.00274529284687124,-0.173021379087149,
-1.88921074867658));
#47860=CARTESIAN_POINT('Ctrl Pts',(0.143983192231577,-0.0959831996176365,
-1.88126345736863));
#47861=CARTESIAN_POINT('Ctrl Pts',(0.158652443090577,0.0690893374944751,
-1.87331616606068));
#47862=CARTESIAN_POINT('Ctrl Pts',(0.0278080418568483,0.170794165773079,
-1.86536887475272));
#47863=CARTESIAN_POINT('Ctrl Pts',(-0.128541480188837,0.115849135192702,
-1.85742158344477));
#47864=CARTESIAN_POINT('Ctrl Pts',(-0.166994675753097,-0.0453509925376745,
-1.84947429213682));
#47865=CARTESIAN_POINT('Ctrl Pts',(-0.0522828479776232,-0.164955867011098,
-1.84152700082887));
#47866=CARTESIAN_POINT('Ctrl Pts',(0.110382027370459,-0.133265683083161,
-1.83357970952092));
#47867=CARTESIAN_POINT('Ctrl Pts',(0.171806155238182,0.0206537956876658,
-1.82563241821296));
#47868=CARTESIAN_POINT('Ctrl Pts',(0.0756522426187192,0.155629921418706,
-1.81768512690501));
#47869=CARTESIAN_POINT('Ctrl Pts',(-0.0898887774288336,0.147864606807659,
-1.80973783559706));
#47870=CARTESIAN_POINT('Ctrl Pts',(-0.172985152874525,0.00448008247821151,
-1.80179054428911));
#47871=CARTESIAN_POINT('Ctrl Pts',(-0.0974221288036245,-0.143013506611804,
-1.79384325298116));
#47872=CARTESIAN_POINT('Ctrl Pts',(0.0674950172757856,-0.159337242655242,
-1.7858959616732));
#47873=CARTESIAN_POINT('Ctrl Pts',(0.170506741222779,-0.0295192386694261,
-1.77794867036526));
#47874=CARTESIAN_POINT('Ctrl Pts',(0.117132227817026,0.127373370296363,
-1.7700013790573));
#47875=CARTESIAN_POINT('Ctrl Pts',(-0.0436742161369485,0.167441025734009,
-1.76205408774936));
#47876=CARTESIAN_POINT('Ctrl Pts',(-0.164423321114139,0.0539342722935164,
-1.7541067964414));
#47877=CARTESIAN_POINT('Ctrl Pts',(-0.134365810835652,-0.109040190446056,
-1.74615950513345));
#47878=CARTESIAN_POINT('Ctrl Pts',(0.0189300150352012,-0.172004618498461,
-1.7382122138255));
#47879=CARTESIAN_POINT('Ctrl Pts',(0.154863513744348,-0.0772089785244452,
-1.73026492251755));
#47880=CARTESIAN_POINT('Ctrl Pts',(0.148758509787723,0.088401583808041,
-1.72231763120959));
#47881=CARTESIAN_POINT('Ctrl Pts',(0.00621442164551661,0.172931533323585,
-1.71437033990164));
#47882=CARTESIAN_POINT('Ctrl Pts',(-0.142029441247508,0.0988512623741091,
-1.70642304859369));
#47883=CARTESIAN_POINT('Ctrl Pts',(-0.160006021153813,-0.0658939105574994,
-1.69847575728574));
#47884=CARTESIAN_POINT('Ctrl Pts',(-0.0312274673769587,-0.170202172533887,
-1.69052846597779));
#47885=CARTESIAN_POINT('Ctrl Pts',(0.126192453246251,-0.118403543011715,
-1.68258117466984));
#47886=CARTESIAN_POINT('Ctrl Pts',(0.167870539828374,0.0419930483742822,
-1.67463388336188));
#47887=CARTESIAN_POINT('Ctrl Pts',(0.0555802736177277,0.163874242755269,
-1.66668659205393));
#47888=CARTESIAN_POINT('Ctrl Pts',(-0.107687389731462,0.135452428353494,
-1.65873930074598));
#47889=CARTESIAN_POINT('Ctrl Pts',(-0.172185787011349,-0.0172043310046124,
-1.65079200943803));
#47890=CARTESIAN_POINT('Ctrl Pts',(-0.0787579512096747,-0.154081534829091,
-1.64284471813008));
#47891=CARTESIAN_POINT('Ctrl Pts',(0.0869055015709199,-0.149637455373784,
-1.63489742682213));
#47892=CARTESIAN_POINT('Ctrl Pts',(0.172860525825677,-0.00794813596417602,
-1.62695013551418));
#47893=CARTESIAN_POINT('Ctrl Pts',(0.10027045663234,0.141031095084652,-1.61900284420622));
#47894=CARTESIAN_POINT('Ctrl Pts',(-0.064286178327947,0.160658711341843,
-1.61105555289827));
#47895=CARTESIAN_POINT('Ctrl Pts',(-0.169880490330225,0.0329325562201978,
-1.60310826159032));
#47896=CARTESIAN_POINT('Ctrl Pts',(-0.119662952948367,-0.124998847777535,
-1.59516097028237));
#47897=CARTESIAN_POINT('Ctrl Pts',(0.0403076582879941,-0.168283174849338,
-1.58721367897441));
#47898=CARTESIAN_POINT('Ctrl Pts',(0.163308687143305,-0.0572206864478598,
-1.57926638766647));
#47899=CARTESIAN_POINT('Ctrl Pts',(0.1365254263793,0.106323761248294,-1.57131909635851));
#47900=CARTESIAN_POINT('Ctrl Pts',(-0.015476917110248,0.172349642560687,
-1.56337180505056));
#47901=CARTESIAN_POINT('Ctrl Pts',(-0.153284063299477,0.0802990049280576,
-1.55542451374261));
#47902=CARTESIAN_POINT('Ctrl Pts',(-0.150501355189484,-0.0854006811457802,
-1.54747722243466));
#47903=CARTESIAN_POINT('Ctrl Pts',(-0.00968105111241323,-0.172772137520472,
-1.53952993112671));
#47904=CARTESIAN_POINT('Ctrl Pts',(0.1400185685051,-0.101679568880954,-1.53158263981875));
#47905=CARTESIAN_POINT('Ctrl Pts',(0.161295247592536,0.0626719822416413,
-1.52363534851081));
#47906=CARTESIAN_POINT('Ctrl Pts',(0.0346343337556016,0.169541726956345,
-1.51568805720285));
#47907=CARTESIAN_POINT('Ctrl Pts',(-0.123792673905044,0.120910330995634,
-1.5077407658949));
#47908=CARTESIAN_POINT('Ctrl Pts',(-0.16867888930721,-0.0386182153409498,
-1.49979347458695));
#47909=CARTESIAN_POINT('Ctrl Pts',(-0.0588553458434272,-0.162726711143821,
-1.491846183279));
#47910=CARTESIAN_POINT('Ctrl Pts',(0.104949442106884,-0.137584697025097,
-1.48389889197105));
#47911=CARTESIAN_POINT('Ctrl Pts',(0.172496168671101,0.0137479470403931,
-1.47595160066309));
#47912=CARTESIAN_POINT('Ctrl Pts',(0.0818319847294822,0.152471179339796,
-1.46800430935515));
#47913=CARTESIAN_POINT('Ctrl Pts',(-0.0838872738395407,0.151350122371288,
-1.46005701804719));
#47914=CARTESIAN_POINT('Ctrl Pts',(-0.172666377295255,0.0114129928488046,
-1.45210972673924));
#47915=CARTESIAN_POINT('Ctrl Pts',(-0.103078457436309,-0.138991963316535,
-1.44416243543129));
#47916=CARTESIAN_POINT('Ctrl Pts',(0.0610514846030254,-0.161915565903346,
-1.43621514412334));
#47917=CARTESIAN_POINT('Ctrl Pts',(0.16918591647428,-0.0363326288725753,
-1.42826785281538));
#47918=CARTESIAN_POINT('Ctrl Pts',(0.122145551731954,0.122574052907337,
-1.42032056150743));
#47919=CARTESIAN_POINT('Ctrl Pts',(-0.0369248894035242,0.169057643413635,
-1.41237327019948));
#47920=CARTESIAN_POINT('Ctrl Pts',(-0.162128373273433,0.0604840874424386,
-1.40442597889153));
#47921=CARTESIAN_POINT('Ctrl Pts',(-0.138630133783172,-0.10356457049249,
-1.39647868758358));
#47922=CARTESIAN_POINT('Ctrl Pts',(0.0120175946397989,-0.17262535060966,
-1.38853139627563));
#47923=CARTESIAN_POINT('Ctrl Pts',(0.15164296468403,-0.0833567364756583,
-1.38058410496768));
#47924=CARTESIAN_POINT('Ctrl Pts',(0.152183671577224,0.0823654318225178,
-1.37263681365972));
#47925=CARTESIAN_POINT('Ctrl Pts',(0.0131437870297985,0.172543255784019,
-1.36468952235177));
#47926=CARTESIAN_POINT('Ctrl Pts',(-0.137951382742217,0.104466981642739,
-1.35674223104382));
#47927=CARTESIAN_POINT('Ctrl Pts',(-0.162519603902411,-0.0594248483501469,
-1.34879493973587));
#47928=CARTESIAN_POINT('Ctrl Pts',(-0.0380272708106778,-0.168813094660117,
-1.34084764842792));
#47929=CARTESIAN_POINT('Ctrl Pts',(0.12134310731451,-0.123368490958159,
-1.33290035711997));
#47930=CARTESIAN_POINT('Ctrl Pts',(0.169419399085581,0.0352278507365205,
-1.32495306581201));
#47931=CARTESIAN_POINT('Ctrl Pts',(0.0621067474779282,0.161513733693909,
-1.31700577450406));
#47932=CARTESIAN_POINT('Ctrl Pts',(-0.1021692856514,0.139661631536786,-1.30905848319611));
#47933=CARTESIAN_POINT('Ctrl Pts',(-0.172737175387357,-0.010286033892214,
-1.30111119188816));
#47934=CARTESIAN_POINT('Ctrl Pts',(-0.0848731068556039,-0.150799502607639,
-1.29316390058021));
#47935=CARTESIAN_POINT('Ctrl Pts',(0.080835308113122,-0.153001918995452,
-1.28521660927226));
#47936=CARTESIAN_POINT('Ctrl Pts',(0.172402785366406,-0.0148732596272302,
-1.2772693179643));
#47937=CARTESIAN_POINT('Ctrl Pts',(0.105845001886694,0.136896931410605,
-1.26932202665635));
#47938=CARTESIAN_POINT('Ctrl Pts',(-0.0577922370382871,0.16310730085482,
-1.2613747353484));
#47939=CARTESIAN_POINT('Ctrl Pts',(-0.168423299000403,0.0397180891767819,
-1.25342744404045));
#47940=CARTESIAN_POINT('Ctrl Pts',(-0.124579025709963,-0.120099960895874,
-1.2454801527325));
#47941=CARTESIAN_POINT('Ctrl Pts',(0.0335272699740489,-0.169764119949185,
-1.23753286142455));
#47942=CARTESIAN_POINT('Ctrl Pts',(0.160882854206129,-0.0637231627944186,
-1.22958557011659));
#47943=CARTESIAN_POINT('Ctrl Pts',(0.140679086570741,0.100763727876932,
-1.22163827880865));
#47944=CARTESIAN_POINT('Ctrl Pts',(-0.00855343890287729,0.172831631760418,
-1.21369098750069));
#47945=CARTESIAN_POINT('Ctrl Pts',(-0.149940877919179,0.0863809434010756,
-1.20574369619274));
#47946=CARTESIAN_POINT('Ctrl Pts',(-0.153804782352703,-0.0792970565624726,
-1.19779640488479));
#47947=CARTESIAN_POINT('Ctrl Pts',(-0.016601236745816,-0.172244980166459,
-1.18984911357684));
#47948=CARTESIAN_POINT('Ctrl Pts',(0.135828715344837,-0.107212379610778,
-1.18190182226888));
#47949=CARTESIAN_POINT('Ctrl Pts',(0.16367859766873,0.0561538148235014,
-1.17395453096093));
#47950=CARTESIAN_POINT('Ctrl Pts',(0.04140491396222,0.168016568688374,-1.16600723965298));
#47951=CARTESIAN_POINT('Ctrl Pts',(-0.11884473864751,0.125777034270327,
-1.15805994834503));
#47952=CARTESIAN_POINT('Ctrl Pts',(-0.170091771343399,-0.0318233181063728,
-1.15011265703708));
#47953=CARTESIAN_POINT('Ctrl Pts',(-0.0653331708643289,-0.160235798243859,
-1.14216536572913));
#47954=CARTESIAN_POINT('Ctrl Pts',(0.0993480384953303,-0.141682396581807,
-1.13421807442118));
#47955=CARTESIAN_POINT('Ctrl Pts',(0.17290871023143,0.00681998388102105,
-1.12627078311322));
#47956=CARTESIAN_POINT('Ctrl Pts',(0.0878800945018856,0.149067176951782,
-1.11832349180527));
#47957=CARTESIAN_POINT('Ctrl Pts',(-0.0777508318389294,0.154592180922545,
-1.11037620049732));
#47958=CARTESIAN_POINT('Ctrl Pts',(-0.172069856051197,0.018327544640642,
-1.10242890918937));
#47959=CARTESIAN_POINT('Ctrl Pts',(-0.10856897732768,-0.134746841952068,
-1.09448161788142));
#47960=CARTESIAN_POINT('Ctrl Pts',(0.0545097464461239,-0.1642334369013,
-1.08653432657347));
#47961=CARTESIAN_POINT('Ctrl Pts',(0.167592944620013,-0.0430875755598672,
-1.07858703526552));
#47962=CARTESIAN_POINT('Ctrl Pts',(0.126962396181698,0.117577566779703,
-1.07063974395756));
#47963=CARTESIAN_POINT('Ctrl Pts',(-0.0301161664627092,0.170402320323477,
-1.06269245264961));
#47964=CARTESIAN_POINT('Ctrl Pts',(-0.159572630867386,0.0669366098043176,
-1.05474516134166));
#47965=CARTESIAN_POINT('Ctrl Pts',(-0.142671460689015,-0.0979223598515507,
-1.04679787003371));
#47966=CARTESIAN_POINT('Ctrl Pts',(0.0050858431223512,-0.172968403050293,
-1.03885057872576));
#47967=CARTESIAN_POINT('Ctrl Pts',(0.148178487554465,-0.0893704094211579,
-1.03090328741781));
#47968=CARTESIAN_POINT('Ctrl Pts',(0.155364035533507,0.0761967894125327,
-1.02295599610985));
#47969=CARTESIAN_POINT('Ctrl Pts',(0.0200520097346351,0.171877430629029,
-1.0150087048019));
#47970=CARTESIAN_POINT('Ctrl Pts',(-0.133651420012675,0.109914658634004,
-1.00706141349395));
#47971=CARTESIAN_POINT('Ctrl Pts',(-0.164771762764467,-0.0528601972142011,
-0.999114122185998));
#47972=CARTESIAN_POINT('Ctrl Pts',(-0.0447659047812013,-0.167152469389939,
-0.991166830878048));
#47973=CARTESIAN_POINT('Ctrl Pts',(0.116298572704249,-0.128134992258121,
-0.983219539570095));
#47974=CARTESIAN_POINT('Ctrl Pts',(0.170695735664292,0.028405986694009,
-0.975272248262145));
#47975=CARTESIAN_POINT('Ctrl Pts',(0.0685333183915558,0.158893418756964,
-0.967324956954192));
#47976=CARTESIAN_POINT('Ctrl Pts',(-0.0964868352949552,0.143646179443793,
-0.959377665646241));
#47977=CARTESIAN_POINT('Ctrl Pts',(-0.173010704215006,-0.00335119099153059,
-0.95143037433829));
#47978=CARTESIAN_POINT('Ctrl Pts',(-0.0908517383104639,-0.147274899083318,
-0.943483083030339));
#47979=CARTESIAN_POINT('Ctrl Pts',(0.0746350855393954,-0.156120268577023,
-0.935535791722385));
#47980=CARTESIAN_POINT('Ctrl Pts',(0.171667723247975,-0.0217744586359998,
-0.927588500414436));
#47981=CARTESIAN_POINT('Ctrl Pts',(0.111249288223971,0.132542559669315,
-0.919641209106481));
#47982=CARTESIAN_POINT('Ctrl Pts',(-0.0512053329868681,0.165293521130557,
-0.911693917798533));
#47983=CARTESIAN_POINT('Ctrl Pts',(-0.166695187287125,0.0464397328733114,
-0.903746626490578));
#47984=CARTESIAN_POINT('Ctrl Pts',(-0.129294704597221,-0.115007885021643,
-0.89579933518263));
#47985=CARTESIAN_POINT('Ctrl Pts',(0.0266929507556997,-0.170971987863474,
-0.887852043874675));
#47986=CARTESIAN_POINT('Ctrl Pts',(0.158198230206126,-0.0701231360799296,
-0.879904752566726));
#47987=CARTESIAN_POINT('Ctrl Pts',(0.144606454839957,0.0950416091649022,
-0.871957461258772));
#47988=CARTESIAN_POINT('Ctrl Pts',(-0.00161620190464337,0.173035609472263,
-0.864010169950822));
#47989=CARTESIAN_POINT('Ctrl Pts',(-0.146356502392492,0.0923239322249147,
-0.85606287864287));
#47990=CARTESIAN_POINT('Ctrl Pts',(-0.156860804015258,-0.0730658772459555,
-0.848115587334918));
#47991=CARTESIAN_POINT('Ctrl Pts',(-0.0234947181556815,-0.171440754993727,
-0.840168296026968));
#47992=CARTESIAN_POINT('Ctrl Pts',(0.131420372415852,-0.112572731903036,
-0.832221004719014));
#47993=CARTESIAN_POINT('Ctrl Pts',(0.165798659537729,0.0495453201576731,
-0.824273713411065));
#47994=CARTESIAN_POINT('Ctrl Pts',(0.048108891535868,0.166221144290443,
-0.816326422103112));
#47995=CARTESIAN_POINT('Ctrl Pts',(-0.113705633508154,0.130441416592061,
-0.808379130795161));
#47996=CARTESIAN_POINT('Ctrl Pts',(-0.171231049144374,-0.0249772308903897,
-0.800431839487209));
#47997=CARTESIAN_POINT('Ctrl Pts',(-0.0717059030162035,-0.157487135114794,
-0.792484548179257));
#47998=CARTESIAN_POINT('Ctrl Pts',(0.0935868267762013,-0.145552190323593,
-0.784537256871307));
#47999=CARTESIAN_POINT('Ctrl Pts',(0.173043116317887,-0.000118949688376935,
-0.776589965563353));
#48000=CARTESIAN_POINT('Ctrl Pts',(0.0937868431381373,0.145423389825078,
-0.768642674255404));
#48001=CARTESIAN_POINT('Ctrl Pts',(-0.0714893223132149,0.157585567388741,
-0.76069538294745));
#48002=CARTESIAN_POINT('Ctrl Pts',(-0.171196548687525,0.0252126153247527,
-0.7527480916395));
#48003=CARTESIAN_POINT('Ctrl Pts',(-0.113884856601376,-0.130284971086147,
-0.744800800331547));
#48004=CARTESIAN_POINT('Ctrl Pts',(0.0478803256378469,-0.166287127195246,
-0.736853509023597));
#48005=CARTESIAN_POINT('Ctrl Pts',(0.165730388064043,-0.0497732129380442,
-0.728906217715644));
#48006=CARTESIAN_POINT('Ctrl Pts',(0.13157501294286,0.112391949102775,-0.720958926407693));
#48007=CARTESIAN_POINT('Ctrl Pts',(-0.0232589996105465,0.171472893458854,
-0.713011635099741));
#48008=CARTESIAN_POINT('Ctrl Pts',(-0.156760204982269,0.0732814600560811,
-0.70506434379179));
#48009=CARTESIAN_POINT('Ctrl Pts',(-0.146483290802742,-0.0921226344045439,
-0.697117052483838));
#48010=CARTESIAN_POINT('Ctrl Pts',(-0.0018540893212253,-0.173033223997078,
-0.689169761175886));
#48011=CARTESIAN_POINT('Ctrl Pts',(0.144475655203828,-0.0952403239571285,
-0.681222469867936));
#48012=CARTESIAN_POINT('Ctrl Pts',(0.158294485823848,0.0699055792608682,
-0.673275178559983));
#48013=CARTESIAN_POINT('Ctrl Pts',(0.0269279774118191,0.170935128883862,
-0.665327887252032));
#48014=CARTESIAN_POINT('Ctrl Pts',(-0.12913646984271,0.115185530387271,
-0.65738059594408));
#48015=CARTESIAN_POINT('Ctrl Pts',(-0.166758874988585,-0.0462105168395193,
-0.649433304636128));
#48016=CARTESIAN_POINT('Ctrl Pts',(-0.0514325297353875,-0.165222967952561,
-0.641486013328178));
#48017=CARTESIAN_POINT('Ctrl Pts',(0.111066963894049,-0.132695379668595,
-0.633538722020224));
#48018=CARTESIAN_POINT('Ctrl Pts',(0.171697496489914,0.0215384296811568,
-0.625591430712274));
#48019=CARTESIAN_POINT('Ctrl Pts',(0.0748496487802092,0.156017512900038,
-0.617644139404321));
#48020=CARTESIAN_POINT('Ctrl Pts',(-0.0906491792717766,0.147399662656966,
-0.609696848096371));
#48021=CARTESIAN_POINT('Ctrl Pts',(-0.173005933504491,0.0035890425288093,
-0.601749556788418));
#48022=CARTESIAN_POINT('Ctrl Pts',(-0.096684228537071,-0.143513393821711,
-0.593802265480468));
#48023=CARTESIAN_POINT('Ctrl Pts',(0.0683148073313607,-0.158987488040138,
-0.585854974172515));
#48024=CARTESIAN_POINT('Ctrl Pts',(0.170656521868019,-0.0286406319403842,
-0.577907682864565));
#48025=CARTESIAN_POINT('Ctrl Pts',(0.116474622480369,0.127974984165225,
-0.569960391556612));
#48026=CARTESIAN_POINT('Ctrl Pts',(-0.0445360616588884,0.167213855484376,
-0.562013100248662));
#48027=CARTESIAN_POINT('Ctrl Pts',(-0.164698934976151,0.053086675086657,
-0.554065808940708));
#48028=CARTESIAN_POINT('Ctrl Pts',(-0.133802404118461,-0.109730811106793,
-0.546118517632758));
#48029=CARTESIAN_POINT('Ctrl Pts',(0.0198156941023548,-0.171904835654138,
-0.538171226324805));
#48030=CARTESIAN_POINT('Ctrl Pts',(0.155259133544419,-0.076410311510098,
-0.530223935016855));
#48031=CARTESIAN_POINT('Ctrl Pts',(0.148301213746763,0.0891666095310972,
-0.522276643708902));
#48032=CARTESIAN_POINT('Ctrl Pts',(0.00532363486478151,0.172961247584135,
-0.514329352400952));
#48033=CARTESIAN_POINT('Ctrl Pts',(-0.142536702432337,0.0981184116960201,
-0.506382061093));
#48034=CARTESIAN_POINT('Ctrl Pts',(-0.159664504357515,-0.0667171664738782,
-0.498434769785048));
#48035=CARTESIAN_POINT('Ctrl Pts',(-0.0303504067061914,-0.170360755653416,
-0.490487478477097));
#48036=CARTESIAN_POINT('Ctrl Pts',(0.126800630838936,-0.117752003264836,
-0.482540187169144));
#48037=CARTESIAN_POINT('Ctrl Pts',(0.167652022935169,0.0428571284593396,
-0.474592895861193));
#48038=CARTESIAN_POINT('Ctrl Pts',(0.0547354826705796,0.164158341825365,
-0.466645604553241));
#48039=CARTESIAN_POINT('Ctrl Pts',(-0.108383625088712,0.134895974983183,
-0.45869831324529));
#48040=CARTESIAN_POINT('Ctrl Pts',(-0.172094890103951,-0.0180909660920301,
-0.450751021937338));
#48041=CARTESIAN_POINT('Ctrl Pts',(-0.0779632913239864,-0.154485143169061,
-0.442803730629387));
#48042=CARTESIAN_POINT('Ctrl Pts',(0.0876750742521607,-0.149187853422831,
-0.434856439321435));
#48043=CARTESIAN_POINT('Ctrl Pts',(0.172899170729097,-0.00705769191907936,
-0.426909148013484));
#48044=CARTESIAN_POINT('Ctrl Pts',(0.0995427292295024,0.141545679240223,
-0.418961856705532));
#48045=CARTESIAN_POINT('Ctrl Pts',(-0.0651128173282645,0.160325466703235,
-0.41101456539758));
#48046=CARTESIAN_POINT('Ctrl Pts',(-0.170047859978802,0.0320571297945394,
-0.403067274089629));
#48047=CARTESIAN_POINT('Ctrl Pts',(-0.119017544302387,-0.125613527942909,
-0.395119982781677));
#48048=CARTESIAN_POINT('Ctrl Pts',(0.0411738860545093,-0.168073333284031,
-0.387172691473725));
#48049=CARTESIAN_POINT('Ctrl Pts',(0.163601242855845,-0.0563787867025962,
-0.379225400165774));
#48050=CARTESIAN_POINT('Ctrl Pts',(0.135975982306233,0.107025541296875,
-0.371278108857821));
#48051=CARTESIAN_POINT('Ctrl Pts',(-0.0163644190684062,0.172267640729731,
-0.363330817549871));
#48052=CARTESIAN_POINT('Ctrl Pts',(-0.153695619597269,0.0795084320726162,
-0.355383526241918));
#48053=CARTESIAN_POINT('Ctrl Pts',(-0.150059492535187,-0.0861747234060912,
-0.347436234933969));
#48054=CARTESIAN_POINT('Ctrl Pts',(-0.0087910393354631,-0.172819709181089,
-0.339488943626015));
#48055=CARTESIAN_POINT('Ctrl Pts',(0.140540423890929,-0.100957037925017,
-0.331541652318065));
#48056=CARTESIAN_POINT('Ctrl Pts',(0.160970308618749,0.0635019212088733,
-0.323594361010112));
#48057=CARTESIAN_POINT('Ctrl Pts',(0.0337606295975726,0.169717866305254,
-0.315647069702161));
#48058=CARTESIAN_POINT('Ctrl Pts',(-0.124413794838165,0.120271118345218,
-0.307699778394209));
#48059=CARTESIAN_POINT('Ctrl Pts',(-0.168477744168953,-0.039486503691345,
-0.299752487086258));
#48060=CARTESIAN_POINT('Ctrl Pts',(-0.0580164219515768,-0.163027694082816,
-0.291805195778306));
#48061=CARTESIAN_POINT('Ctrl Pts',(0.105656696284218,-0.137042317494962,
-0.283857904470355));
#48062=CARTESIAN_POINT('Ctrl Pts',(0.172423070161505,0.0146362266327961,
-0.275910613162403));
#48063=CARTESIAN_POINT('Ctrl Pts',(0.0810455783953381,0.152890642213818,
-0.267963321854451));
#48064=CARTESIAN_POINT('Ctrl Pts',(-0.0846657078511696,0.150916043442814,
-0.2600160305465));
#48065=CARTESIAN_POINT('Ctrl Pts',(-0.172722870928364,0.0105235028277298,
-0.252068739238548));
#48066=CARTESIAN_POINT('Ctrl Pts',(-0.102361195579199,-0.139521037458531,
-0.244121447930597));
#48067=CARTESIAN_POINT('Ctrl Pts',(0.0618846400935952,-0.161598965271126,
-0.236174156622645));
#48068=CARTESIAN_POINT('Ctrl Pts',(0.169370807803051,-0.0354607348225401,
-0.228226865314694));
#48069=CARTESIAN_POINT('Ctrl Pts',(0.121512599367703,0.123201552138589,
-0.220279574006742));
#48070=CARTESIAN_POINT('Ctrl Pts',(-0.0377951510689661,0.168865214959562,
-0.21233228269879));
#48071=CARTESIAN_POINT('Ctrl Pts',(-0.162437753107342,0.0596482236948258,
-0.204384991390838));
#48072=CARTESIAN_POINT('Ctrl Pts',(-0.138094873460796,-0.104277227568877,
-0.196437700082887));
#48073=CARTESIAN_POINT('Ctrl Pts',(0.0129065627974987,-0.172561162992656,
-0.188490408774936));
#48074=CARTESIAN_POINT('Ctrl Pts',(0.152070291491269,-0.0825745753144448,
-0.180543117466984));
#48075=CARTESIAN_POINT('Ctrl Pts',(0.151757420906439,0.0831481785180167,
-0.172595826159032));
#48076=CARTESIAN_POINT('Ctrl Pts',(0.012254906519396,0.172608667222736,
-0.164648534851081));
#48077=CARTESIAN_POINT('Ctrl Pts',(-0.138487619250733,0.103755058131125,
-0.156701243543129));
#48078=CARTESIAN_POINT('Ctrl Pts',(-0.162211379504551,-0.0602611311391257,
-0.148753952235178));
#48079=CARTESIAN_POINT('Ctrl Pts',(-0.0371572630349655,-0.169006729728073,
-0.140806660927225));
#48080=CARTESIAN_POINT('Ctrl Pts',(0.121976899919814,-0.12274184287718,
-0.132859369619274));
#48081=CARTESIAN_POINT('Ctrl Pts',(0.169235748100154,0.0360999609252447,
-0.124912078311322));
#48082=CARTESIAN_POINT('Ctrl Pts',(0.0612739492687115,0.161831550093002,
-0.116964787003371));
#48083=CARTESIAN_POINT('Ctrl Pts',(-0.102887124683252,0.139133409897374,
-0.109017495695419));
#48084=CARTESIAN_POINT('Ctrl Pts',(-0.17268218848071,-0.0111753462307528,
-0.101070204387468));
#48085=CARTESIAN_POINT('Ctrl Pts',(-0.0840947316560137,-0.151235134400324,
-0.093122913079516));
#48086=CARTESIAN_POINT('Ctrl Pts',(0.0816212678773405,-0.152582620718228,
-0.0851756217715646));
#48087=CARTESIAN_POINT('Ctrl Pts',(0.172479045841006,-0.013986821845635,
-0.0772283304636131));
#48088=CARTESIAN_POINT('Ctrl Pts',(0.105134810098645,0.137443586413713,
-0.0692810391556613));
#48089=CARTESIAN_POINT('Ctrl Pts',(-0.0586245811406043,0.162801200529421,
-0.0613337478477097));
#48090=CARTESIAN_POINT('Ctrl Pts',(-0.168638912927327,0.0388619839671219,
-0.0533864565397582));
#48091=CARTESIAN_POINT('Ctrl Pts',(-0.12393356787755,-0.120762648130661,
-0.0454391652318062));
#48092=CARTESIAN_POINT('Ctrl Pts',(0.0343531967590567,-0.16954605151339,
-0.0374918739238549));
#48093=CARTESIAN_POINT('Ctrl Pts',(0.161301394425332,-0.0629771683730991,
-0.0295445826159031));
#48094=CARTESIAN_POINT('Ctrl Pts',(0.139971593454551,0.10165914811014,-0.0215972913079518));
#48095=CARTESIAN_POINT('Ctrl Pts',(0.0406598484393165,0.148790668971504,
-0.0162990971026507));
#48096=CARTESIAN_POINT('Ctrl Pts',(-0.00798678478681935,0.146131905375825,
-0.0136500000000002));
#48097=CARTESIAN_POINT('Ctrl Pts',(-0.129787930238029,0.0433148218226557,
-2.94864852262806));
#48098=CARTESIAN_POINT('Ctrl Pts',(-0.144207233435665,0.000109022081449632,
-2.94599942552541));
#48099=CARTESIAN_POINT('Ctrl Pts',(-0.126253311240158,-0.101084246503596,
-2.94070123132011));
#48100=CARTESIAN_POINT('Ctrl Pts',(0.0169219107275231,-0.161002946168919,
-2.93275394001216));
#48101=CARTESIAN_POINT('Ctrl Pts',(0.14438368807171,-0.0728747486437721,
-2.92480664870421));
#48102=CARTESIAN_POINT('Ctrl Pts',(0.139514764084194,0.0819023268038132,
-2.91685935739625));
#48103=CARTESIAN_POINT('Ctrl Pts',(0.0066351667127898,0.161659351292547,
-2.90891206608831));
#48104=CARTESIAN_POINT('Ctrl Pts',(-0.132303943561717,0.0930925035302517,
-2.90096477478035));
#48105=CARTESIAN_POINT('Ctrl Pts',(-0.149909626174738,-0.0608298430199986,
-2.8930174834724));
#48106=CARTESIAN_POINT('Ctrl Pts',(-0.0300131822609338,-0.158974481534216,
-2.88507019216445));
#48107=CARTESIAN_POINT('Ctrl Pts',(0.11740708193013,-0.111302451803343,
-2.8771229008565));
#48108=CARTESIAN_POINT('Ctrl Pts',(0.157145337254098,0.0384504960783959,
-2.86917560954854));
#48109=CARTESIAN_POINT('Ctrl Pts',(0.0527511745255854,0.152939345598777,
-2.8612283182406));
#48110=CARTESIAN_POINT('Ctrl Pts',(-0.100025018952735,0.127153392495664,
-2.85328102693264));
#48111=CARTESIAN_POINT('Ctrl Pts',(-0.161060052911221,-0.0152551646415358,
-2.8453337356247));
#48112=CARTESIAN_POINT('Ctrl Pts',(-0.0743730558561778,-0.143672222913865,
-2.83738644431673));
#48113=CARTESIAN_POINT('Ctrl Pts',(0.0805277158933123,-0.140315099860671,
-2.8294391530088));
#48114=CARTESIAN_POINT('Ctrl Pts',(0.16156971197941,-0.00826314829488561,
-2.82149186170083));
#48115=CARTESIAN_POINT('Ctrl Pts',(0.0944223578173568,0.131367684903636,
-2.81354457039289));
#48116=CARTESIAN_POINT('Ctrl Pts',(-0.0593277612398802,0.150510014940419,
-2.80559727908493));
#48117=CARTESIAN_POINT('Ctrl Pts',(-0.158663349758915,0.0316068190134606,
-2.79764998777698));
#48118=CARTESIAN_POINT('Ctrl Pts',(-0.112475279434508,-0.116285686053977,
-2.78970269646903));
#48119=CARTESIAN_POINT('Ctrl Pts',(0.0368734361630542,-0.157522692542648,
-2.78175540516108));
#48120=CARTESIAN_POINT('Ctrl Pts',(0.152402387559763,-0.0542822391159111,
-2.77380811385312));
#48121=CARTESIAN_POINT('Ctrl Pts',(0.128150143997042,0.0987450745547089,
-2.76586082254518));
#48122=CARTESIAN_POINT('Ctrl Pts',(-0.0136394980791459,0.161204879614442,
-2.75791353123722));
#48123=CARTESIAN_POINT('Ctrl Pts',(-0.142919196291981,0.0758099761794772,
-2.74996623992927));
#48124=CARTESIAN_POINT('Ctrl Pts',(-0.141115541404577,-0.0791167056924326,
-2.74201894862132));
#48125=CARTESIAN_POINT('Ctrl Pts',(-0.00988281885907166,-0.16147872625534,
-2.73407165731337));
#48126=CARTESIAN_POINT('Ctrl Pts',(0.130414277611373,-0.0957348700431142,
-2.72612436600542));
#48127=CARTESIAN_POINT('Ctrl Pts',(0.151097345755275,0.0578155796543157,
-2.71817707469747));
#48128=CARTESIAN_POINT('Ctrl Pts',(0.0331961842888706,0.158338442879036,
-2.71022978338952));
#48129=CARTESIAN_POINT('Ctrl Pts',(-0.115152021785071,0.113635650322734,
-2.70228249208156));
#48130=CARTESIAN_POINT('Ctrl Pts',(-0.157884512716944,-0.035292064111602,
-2.69433520077361));
#48131=CARTESIAN_POINT('Ctrl Pts',(-0.0558076858302437,-0.151850424258141,
-2.68638790946566));
#48132=CARTESIAN_POINT('Ctrl Pts',(0.0974551172814357,-0.129133842430521,
-2.67844061815771));
#48133=CARTESIAN_POINT('Ctrl Pts',(0.161333541845059,0.0120223716829652,
-2.67049332684976));
#48134=CARTESIAN_POINT('Ctrl Pts',(0.0772392505677555,0.142151845984807,
-2.66254603554181));
#48135=CARTESIAN_POINT('Ctrl Pts',(-0.0776977281342388,0.141901769502529,
-2.65459874423385));
#48136=CARTESIAN_POINT('Ctrl Pts',(-0.161371510632747,0.0115015086517994,
-2.6466514529259));
#48137=CARTESIAN_POINT('Ctrl Pts',(-0.0970377528850418,-0.129447764214701,
-2.63870416161795));
#48138=CARTESIAN_POINT('Ctrl Pts',(0.0562975830174607,-0.151669480422257,
-2.63075687031));
#48139=CARTESIAN_POINT('Ctrl Pts',(0.157997616309539,-0.0347822136395501,
-2.62280957900205));
#48140=CARTESIAN_POINT('Ctrl Pts',(0.114784594855777,0.114006780188545,
-2.6148622876941));
#48141=CARTESIAN_POINT('Ctrl Pts',(-0.0337071432447416,0.158230457369758,
-2.60691499638614));
#48142=CARTESIAN_POINT('Ctrl Pts',(-0.151283192814987,0.0573275214610534,
-2.59896770507819));
#48143=CARTESIAN_POINT('Ctrl Pts',(-0.130104556621024,-0.0961553612213634,
-2.59102041377024));
#48144=CARTESIAN_POINT('Ctrl Pts',(0.0104040364209517,-0.16144598220865,
-2.58307312246229));
#48145=CARTESIAN_POINT('Ctrl Pts',(0.141370202591794,-0.0786607587321608,
-2.57512583115434));
#48146=CARTESIAN_POINT('Ctrl Pts',(0.142673729628386,0.0762709382339727,
-2.56717853984639));
#48147=CARTESIAN_POINT('Ctrl Pts',(0.0131190419946609,0.161248069390943,
-2.55923124853843));
#48148=CARTESIAN_POINT('Ctrl Pts',(-0.128468235086874,0.0983308787656647,
-2.55128395723048));
#48149=CARTESIAN_POINT('Ctrl Pts',(-0.152226365000939,-0.0547739257655036,
-2.54333666592253));
#48150=CARTESIAN_POINT('Ctrl Pts',(-0.0363647457035736,-0.157640903369266,
-2.53538937461458));
#48151=CARTESIAN_POINT('Ctrl Pts',(0.112850075420815,-0.115921998010216,
-2.52744208330662));
#48152=CARTESIAN_POINT('Ctrl Pts',(0.158560492241468,0.0321188331872045,
-2.51949479199867));
#48153=CARTESIAN_POINT('Ctrl Pts',(0.0588415929153526,0.150700750125366,
-2.51154750069073));
#48154=CARTESIAN_POINT('Ctrl Pts',(-0.094845936916996,0.131062189038263,
-2.50360020938277));
#48155=CARTESIAN_POINT('Ctrl Pts',(-0.161542189476235,-0.00878465505231707,
-2.49565291807482));
#48156=CARTESIAN_POINT('Ctrl Pts',(-0.0800743577022627,-0.140574344685416,
-2.48770562676687));
#48157=CARTESIAN_POINT('Ctrl Pts',(0.0748364794314408,-0.14343134417369,
-2.47975833545891));
#48158=CARTESIAN_POINT('Ctrl Pts',(0.161108414952932,-0.0147352562420184,
-2.47181104415097));
#48159=CARTESIAN_POINT('Ctrl Pts',(0.0996141176576514,0.127475788714766,
-2.46386375284301));
#48160=CARTESIAN_POINT('Ctrl Pts',(-0.0532447610962578,0.152767943499173,
-2.45591646153507));
#48161=CARTESIAN_POINT('Ctrl Pts',(-0.157268339926687,0.0379436213594348,
-2.44796917022711));
#48162=CARTESIAN_POINT('Ctrl Pts',(-0.117047745421395,-0.111682023785981,
-2.44002187891916));
#48163=CARTESIAN_POINT('Ctrl Pts',(0.0305272936401855,-0.158874584147906,
-2.43207458761121));
#48164=CARTESIAN_POINT('Ctrl Pts',(0.150103154753057,-0.0603497479559275,
-2.42412729630326));
#48165=CARTESIAN_POINT('Ctrl Pts',(0.132006643393938,0.0935269760284694,
-2.4161800049953));
#48166=CARTESIAN_POINT('Ctrl Pts',(-0.00716439040280769,0.161622153974386,
-2.40823271368735));
#48167=CARTESIAN_POINT('Ctrl Pts',(-0.139764352287754,0.0814799053432716,
-2.4002854223794));
#48168=CARTESIAN_POINT('Ctrl Pts',(-0.144174536961678,-0.0733944959588244,
-2.39233813107145));
#48169=CARTESIAN_POINT('Ctrl Pts',(-0.0163499888865172,-0.160952561360715,
-2.3843908397635));
#48170=CARTESIAN_POINT('Ctrl Pts',(0.126470524887037,-0.100887340533693,
-2.37644354845554));
#48171=CARTESIAN_POINT('Ctrl Pts',(0.153294161462234,0.0517102427644136,
-2.3684962571476));
#48172=CARTESIAN_POINT('Ctrl Pts',(0.0395186818540962,0.156879963442368,
-2.36054896583964));
#48173=CARTESIAN_POINT('Ctrl Pts',(-0.110502742729481,0.118161723897488,
-2.35260167453169));
#48174=CARTESIAN_POINT('Ctrl Pts',(-0.159172701507709,-0.0289326846300512,
-2.34465438322374));
#48175=CARTESIAN_POINT('Ctrl Pts',(-0.0618518349405682,-0.149490466785172,
-2.33670709191578));
#48176=CARTESIAN_POINT('Ctrl Pts',(0.0921986111748694,-0.132937824724904,
-2.32875980060784));
#48177=CARTESIAN_POINT('Ctrl Pts',(0.16168586766282,0.00554340538704512,
-2.32081250929988));
#48178=CARTESIAN_POINT('Ctrl Pts',(0.0828772603299642,0.138940306842052,
-2.31286521799194));
#48179=CARTESIAN_POINT('Ctrl Pts',(-0.0719451328049027,0.144903233265683,
-2.30491792668398));
#48180=CARTESIAN_POINT('Ctrl Pts',(-0.160780524285084,0.0179630775697664,
-2.29697063537603));
#48181=CARTESIAN_POINT('Ctrl Pts',(-0.102150419373578,-0.125452544681112,
-2.28902334406807));
#48182=CARTESIAN_POINT('Ctrl Pts',(0.0501705250629579,-0.153804965979877,
-2.28107605276013));
#48183=CARTESIAN_POINT('Ctrl Pts',(0.15647581296685,-0.0410897688181301,
-2.27312876145218));
#48184=CARTESIAN_POINT('Ctrl Pts',(0.119263821430011,0.109312350825853,
-2.26518147014422));
#48185=CARTESIAN_POINT('Ctrl Pts',(-0.027335166491799,0.159454814345725,
-2.25723417883627));
#48186=CARTESIAN_POINT('Ctrl Pts',(-0.148862747826359,0.0633477028371972,
-2.24928688752832));
#48187=CARTESIAN_POINT('Ctrl Pts',(-0.133855639402594,-0.0908609759208357,
-2.24133959622037));
#48188=CARTESIAN_POINT('Ctrl Pts',(0.00392186299208866,-0.161733324135243,
-2.23339230491242));
#48189=CARTESIAN_POINT('Ctrl Pts',(0.138102291204558,-0.0842662821608703,
-2.22544501360447));
#48190=CARTESIAN_POINT('Ctrl Pts',(0.145617359816636,0.0704885357004696,
-2.21749772229651));
#48191=CARTESIAN_POINT('Ctrl Pts',(0.0195743600986712,0.16059232102405,
-2.20955043098856));
#48192=CARTESIAN_POINT('Ctrl Pts',(-0.124421950453024,0.103403227177053,
-2.20160313968061));
#48193=CARTESIAN_POINT('Ctrl Pts',(-0.154300305691649,-0.0486257628076713,
-2.19365584837266));
#48194=CARTESIAN_POINT('Ctrl Pts',(-0.042656724281636,-0.156055929136719,
-2.18570855706471));
#48195=CARTESIAN_POINT('Ctrl Pts',(0.108110967766809,-0.12035392720509,
-2.17776126575676));
#48196=CARTESIAN_POINT('Ctrl Pts',(0.15972089429603,0.0257348998529341,
-2.1698139744488));
#48197=CARTESIAN_POINT('Ctrl Pts',(0.0648372012390534,0.148220060992602,
-2.16186668314085));
#48198=CARTESIAN_POINT('Ctrl Pts',(-0.089514204763127,0.134759995142434,
-2.1539193918329));
#48199=CARTESIAN_POINT('Ctrl Pts',(-0.161764518619993,-0.00229992626103489,
-2.14597210052495));
#48200=CARTESIAN_POINT('Ctrl Pts',(-0.0856468311724065,-0.137250389636203,
-2.138024809217));
#48201=CARTESIAN_POINT('Ctrl Pts',(0.0690248511036805,-0.146316844810428,
-2.13007751790905));
#48202=CARTESIAN_POINT('Ctrl Pts',(0.160387970501104,-0.0211836744617428,
-2.1221302266011));
#48203=CARTESIAN_POINT('Ctrl Pts',(0.104645637976606,0.123378845827124,
-2.11418293529314));
#48204=CARTESIAN_POINT('Ctrl Pts',(-0.0470761113215489,0.154780130792054,
-2.10623564398519));
#48205=CARTESIAN_POINT('Ctrl Pts',(-0.155620354170519,0.0442193906901315,
-2.09828835267724));
#48206=CARTESIAN_POINT('Ctrl Pts',(-0.121431931614596,-0.106898714349201,
-2.09034106136929));
#48207=CARTESIAN_POINT('Ctrl Pts',(0.0241320456173179,-0.159970914604774,
-2.08239377006134));
#48208=CARTESIAN_POINT('Ctrl Pts',(0.147562470904876,-0.066320180379818,
-2.07444647875339));
#48209=CARTESIAN_POINT('Ctrl Pts',(0.135650801013122,0.0881584331171016,
-2.06649918744543));
#48210=CARTESIAN_POINT('Ctrl Pts',(-0.000677758276635096,0.161779447980522,
-2.05855189613748));
#48211=CARTESIAN_POINT('Ctrl Pts',(-0.136384687794117,0.0870187685529117,
-2.05060460482953));
#48212=CARTESIAN_POINT('Ctrl Pts',(-0.147001617915132,-0.067554226185322,
-2.04265731352158));
#48213=CARTESIAN_POINT('Ctrl Pts',(-0.0227908588453908,-0.160167493263313,
-2.03471002221363));
#48214=CARTESIAN_POINT('Ctrl Pts',(0.122323335685659,-0.10587752685012,
-2.02676273090567));
#48215=CARTESIAN_POINT('Ctrl Pts',(0.155244393035563,0.0455217264191934,
-2.01881543959773));
#48216=CARTESIAN_POINT('Ctrl Pts',(0.0457776109203872,0.15516913186451,
-2.01086814828977));
#48217=CARTESIAN_POINT('Ctrl Pts',(-0.105675712462875,0.122497726267175,
-2.00292085698182));
#48218=CARTESIAN_POINT('Ctrl Pts',(-0.160204850132875,-0.0225267649489869,
-1.99497356567387));
#48219=CARTESIAN_POINT('Ctrl Pts',(-0.0677964911486736,-0.146890043682654,
-1.98702627436592));
#48220=CARTESIAN_POINT('Ctrl Pts',(0.0867937973030992,-0.136527967445768,
-1.97907898305797));
#48221=CARTESIAN_POINT('Ctrl Pts',(0.161778110715712,-0.0009444778551103,
-1.97113169175001));
#48222=CARTESIAN_POINT('Ctrl Pts',(0.0883819563566127,0.135505272723026,
-1.96318440044206));
#48223=CARTESIAN_POINT('Ctrl Pts',(-0.0660768088140216,0.147671610278073,
-1.95523710913411));
#48224=CARTESIAN_POINT('Ctrl Pts',(-0.15993091147926,0.024395751650182,
-1.94728981782616));
#48225=CARTESIAN_POINT('Ctrl Pts',(-0.107098769933436,-0.12125552615823,
-1.93934252651821));
#48226=CARTESIAN_POINT('Ctrl Pts',(0.043962764391142,-0.155693045741462,
-1.93139523521026));
#48227=CARTESIAN_POINT('Ctrl Pts',(0.154702307588264,-0.0473312282962324,
-1.92344794390231));
#48228=CARTESIAN_POINT('Ctrl Pts',(0.123551203999137,0.10444208507842,-1.91550065259435));
#48229=CARTESIAN_POINT('Ctrl Pts',(-0.0209192192559613,0.160422677358549,
-1.9075533612864));
#48230=CARTESIAN_POINT('Ctrl Pts',(-0.146202846937255,0.0692659851052862,
-1.89960606997845));
#48231=CARTESIAN_POINT('Ctrl Pts',(-0.137391406242903,-0.0854204345327365,
-1.8916587786705));
#48232=CARTESIAN_POINT('Ctrl Pts',(-0.00256661902134908,-0.161760506960022,
-1.88371148736255));
#48233=CARTESIAN_POINT('Ctrl Pts',(0.134612232846497,-0.0897362575174868,
-1.87576419605459));
#48234=CARTESIAN_POINT('Ctrl Pts',(0.148326754532756,0.0645927475413762,
-1.86781690474665));
#48235=CARTESIAN_POINT('Ctrl Pts',(0.0259981915071029,0.159678248936804,
-1.85986961343869));
#48236=CARTESIAN_POINT('Ctrl Pts',(-0.120175524611116,0.108309244432814,
-1.85192232213074));
#48237=CARTESIAN_POINT('Ctrl Pts',(-0.15612604379855,-0.0423993819881522,
-1.84397503082279));
#48238=CARTESIAN_POINT('Ctrl Pts',(-0.0488800866043013,-0.154219928280103,
-1.83602773951484));
#48239=CARTESIAN_POINT('Ctrl Pts',(0.103197956234794,-0.124592258885236,
-1.82808044820689));
#48240=CARTESIAN_POINT('Ctrl Pts',(0.160624374379668,0.0193095701739912,
-1.82013315689893));
#48241=CARTESIAN_POINT('Ctrl Pts',(0.070728514494755,0.145500949765042,
-1.81218586559098));
#48242=CARTESIAN_POINT('Ctrl Pts',(-0.084038482895108,0.13824103058735,
-1.80423857428303));
#48243=CARTESIAN_POINT('Ctrl Pts',(-0.161726638483477,0.00418850211877394,
-1.79629128297508));
#48244=CARTESIAN_POINT('Ctrl Pts',(-0.0910815358630474,-0.133705657958041,
-1.78834399166713));
#48245=CARTESIAN_POINT('Ctrl Pts',(0.063102191587005,-0.14896698480563,
-1.78039670035917));
#48246=CARTESIAN_POINT('Ctrl Pts',(0.1594095310407,-0.0275980172937854,
-1.77244940905123));
#48247=CARTESIAN_POINT('Ctrl Pts',(0.109508828637277,0.119083439636481,
-1.76450211774327));
#48248=CARTESIAN_POINT('Ctrl Pts',(-0.0408317364054441,0.15654334366967,
-1.75655482643532));
#48249=CARTESIAN_POINT('Ctrl Pts',(-0.153722042442376,0.0504240301097478,
-1.74860753512737));
#48250=CARTESIAN_POINT('Ctrl Pts',(-0.125620786249326,-0.101943451026858,
-1.74066024381942));
#48251=CARTESIAN_POINT('Ctrl Pts',(0.0176979795503254,-0.160809920915969,
-1.73271295251147));
#48252=CARTESIAN_POINT('Ctrl Pts',(0.144784422740484,-0.0721839322624418,
-1.72476566120351));
#48253=CARTESIAN_POINT('Ctrl Pts',(0.139076755050945,0.0826480813429048,
-1.71681836989556));
#48254=CARTESIAN_POINT('Ctrl Pts',(0.00580996407003145,0.161676508691489,
-1.70887107858761));
#48255=CARTESIAN_POINT('Ctrl Pts',(-0.132785639212092,0.0924176561280391,
-1.70092378727966));
#48256=CARTESIAN_POINT('Ctrl Pts',(-0.149592236722726,-0.0616052908235646,
-1.69297649597171));
#48257=CARTESIAN_POINT('Ctrl Pts',(-0.0291950681506911,-0.159124784810037,
-1.68502920466376));
#48258=CARTESIAN_POINT('Ctrl Pts',(0.117979381041458,-0.110697401930842,
-1.67708191335581));
#48259=CARTESIAN_POINT('Ctrl Pts',(0.156944903396088,0.0392599852668939,
-1.66913462204785));
#48260=CARTESIAN_POINT('Ctrl Pts',(0.0519629035718947,0.153208700136586,
-1.6611873307399));
#48261=CARTESIAN_POINT('Ctrl Pts',(-0.1006786955928,0.126636682674872,-1.65324003943195));
#48262=CARTESIAN_POINT('Ctrl Pts',(-0.16097929831109,-0.016084609427433,
-1.645292748124));
#48263=CARTESIAN_POINT('Ctrl Pts',(-0.0736320920687726,-0.144053337909053,
-1.63734545681605));
#48264=CARTESIAN_POINT('Ctrl Pts',(0.0812493696784421,-0.139898495603134,
-1.6293981655081));
#48265=CARTESIAN_POINT('Ctrl Pts',(0.161610122624517,-0.00743084184010702,
-1.62145087420014));
#48266=CARTESIAN_POINT('Ctrl Pts',(0.0937444839680286,0.131852269114839,
-1.61350358289219));
#48267=CARTESIAN_POINT('Ctrl Pts',(-0.0601021957616684,0.150202447416113,
-1.60555629158424));
#48268=CARTESIAN_POINT('Ctrl Pts',(-0.158824038875523,0.0307891834972998,
-1.59760900027629));
#48269=CARTESIAN_POINT('Ctrl Pts',(-0.111874844804655,-0.116863459837105,
-1.58966170896834));
#48270=CARTESIAN_POINT('Ctrl Pts',(0.0376842866091804,-0.157330682601715,
-1.58171441766039));
#48271=CARTESIAN_POINT('Ctrl Pts',(0.152679952978355,-0.0534965522598539,
-1.57376712635243));
#48272=CARTESIAN_POINT('Ctrl Pts',(0.127639846015364,0.0994038171014477,
-1.56581983504448));
#48273=CARTESIAN_POINT('Ctrl Pts',(-0.0144696220267058,0.161132489534446,
-1.55787254373653));
#48274=CARTESIAN_POINT('Ctrl Pts',(-0.143307768779982,0.0750728483039466,
-1.54992525242858));
#48275=CARTESIAN_POINT('Ctrl Pts',(-0.140706169619418,-0.0798424885395985,
-1.54197796112063));
#48276=CARTESIAN_POINT('Ctrl Pts',(-0.00905097245273122,-0.161527486957557,
-1.53403066981268));
#48277=CARTESIAN_POINT('Ctrl Pts',(0.130905641514927,-0.095061885972925,
-1.52608337850473));
#48278=CARTESIAN_POINT('Ctrl Pts',(0.15079755553023,0.0585930575347549,
-1.51813608719677));
#48279=CARTESIAN_POINT('Ctrl Pts',(0.0323802030482504,0.158507323476609,
-1.51018879588882));
#48280=CARTESIAN_POINT('Ctrl Pts',(-0.115735788227241,0.113041038869003,
-1.50224150458087));
#48281=CARTESIAN_POINT('Ctrl Pts',(-0.15770064249716,-0.0361047988658983,
-1.49429421327292));
#48282=CARTESIAN_POINT('Ctrl Pts',(-0.0550248219680774,-0.152135854132237,
-1.48634692196497));
#48283=CARTESIAN_POINT('Ctrl Pts',(0.0981189437394838,-0.128630175404576,
-1.47839963065702));
#48284=CARTESIAN_POINT('Ctrl Pts',(0.161269479182942,0.0128531797321523,
-1.47045233934906));
#48285=CARTESIAN_POINT('Ctrl Pts',(0.0765060561025797,0.142547790318873,
-1.46250504804111));
#48286=CARTESIAN_POINT('Ctrl Pts',(-0.0784275793856785,0.141499695889663,
-1.45455775673316));
#48287=CARTESIAN_POINT('Ctrl Pts',(-0.161428609999475,0.0106701930067575,
-1.44661046542521));
#48288=CARTESIAN_POINT('Ctrl Pts',(-0.0963697296803828,-0.129945851594016,
-1.43866317411726));
#48289=CARTESIAN_POINT('Ctrl Pts',(0.057078027883893,-0.151377501228055,
-1.43071588280931));
#48290=CARTESIAN_POINT('Ctrl Pts',(0.158174670458443,-0.0339679668294594,
-1.42276859150135));
#48291=CARTESIAN_POINT('Ctrl Pts',(0.114195866865224,0.114596479597168,
-1.4148213001934));
#48292=CARTESIAN_POINT('Ctrl Pts',(-0.0345216808516293,0.158054745883641,
-1.40687400888545));
#48293=CARTESIAN_POINT('Ctrl Pts',(-0.151576458306368,0.056547559031861,
-1.3989267175775));
#48294=CARTESIAN_POINT('Ctrl Pts',(-0.129607571266712,-0.0968242046985573,
-1.39097942626955));
#48295=CARTESIAN_POINT('Ctrl Pts',(0.0112354450740637,-0.16139025348252,
-1.3830321349616));
#48296=CARTESIAN_POINT('Ctrl Pts',(0.141773478940156,-0.0779315713582716,
-1.37508484365364));
#48297=CARTESIAN_POINT('Ctrl Pts',(0.142278994626267,0.07700478448319,-1.36713755234569));
#48298=CARTESIAN_POINT('Ctrl Pts',(0.0122883406925415,0.161313501692165,
-1.35919026103774));
#48299=CARTESIAN_POINT('Ctrl Pts',(-0.128972995857213,0.0976678835891277,
-1.35124296972979));
#48300=CARTESIAN_POINT('Ctrl Pts',(-0.151942226197115,-0.0555572591425189,
-1.34329567842184));
#48301=CARTESIAN_POINT('Ctrl Pts',(-0.0355523151942074,-0.157826113268673,
-1.33534838711389));
#48302=CARTESIAN_POINT('Ctrl Pts',(0.113445648502268,-0.115339212677492,
-1.32740109580593));
#48303=CARTESIAN_POINT('Ctrl Pts',(0.158392957156713,0.0329350917459731,
-1.31945380449798));
#48304=CARTESIAN_POINT('Ctrl Pts',(0.0580646103427997,0.151001821746967,
-1.31150651319003));
#48305=CARTESIAN_POINT('Ctrl Pts',(-0.0955197301622941,0.13057193532642,
-1.30355922188208));
#48306=CARTESIAN_POINT('Ctrl Pts',(-0.161494800289547,-0.0096165807126814,
-1.29561193057413));
#48307=CARTESIAN_POINT('Ctrl Pts',(-0.0793492507380876,-0.140984912499416,
-1.28766463926618));
#48308=CARTESIAN_POINT('Ctrl Pts',(0.0755742468915394,-0.143043987472178,
-1.27971734795822));
#48309=CARTESIAN_POINT('Ctrl Pts',(0.161182173609555,-0.0139052528083161,
-1.27177005665028));
#48310=CARTESIAN_POINT('Ctrl Pts',(0.0989562171721762,0.127987172123371,
-1.26382276534232));
#48311=CARTESIAN_POINT('Ctrl Pts',(-0.0540309042211304,0.152491673655355,
-1.25587547403437));
#48312=CARTESIAN_POINT('Ctrl Pts',(-0.157461686954082,0.037133088839183,
-1.24792818272642));
#48313=CARTESIAN_POINT('Ctrl Pts',(-0.116470961344493,-0.112283410656488,
-1.23998089141847));
#48314=CARTESIAN_POINT('Ctrl Pts',(0.0313451910775401,-0.158715242309856,
-1.23203360011052));
#48315=CARTESIAN_POINT('Ctrl Pts',(0.150412002232682,-0.0595758233641786,
-1.22408630880256));
#48316=CARTESIAN_POINT('Ctrl Pts',(0.13152317061867,0.0942056512932029,
-1.21613901749462));
#48317=CARTESIAN_POINT('Ctrl Pts',(-0.00799674942183057,0.161583109092035,
-1.20819172618666));
#48318=CARTESIAN_POINT('Ctrl Pts',(-0.140182170285556,0.0807589516969816,
-1.20024443487871));
#48319=CARTESIAN_POINT('Ctrl Pts',(-0.143794597508774,-0.0741361104486446,
-1.19229714357076));
#48320=CARTESIAN_POINT('Ctrl Pts',(-0.0155207667765463,-0.161034638956444,
-1.18434985226281));
#48321=CARTESIAN_POINT('Ctrl Pts',(0.126988479515248,-0.10023460088996,
-1.17640256095485));
#48322=CARTESIAN_POINT('Ctrl Pts',(0.153025788356846,0.0524991165918986,
-1.1684552696469));
#48323=CARTESIAN_POINT('Ctrl Pts',(0.0387101288205123,0.157081428157065,
-1.16050797833895));
#48324=CARTESIAN_POINT('Ctrl Pts',(-0.111109882920702,0.117590999070983,
-1.152560687031));
#48325=CARTESIAN_POINT('Ctrl Pts',(-0.159021568937894,-0.029752138707914,
-1.14461339572305));
#48326=CARTESIAN_POINT('Ctrl Pts',(-0.0610810461463133,-0.149807059068777,
-1.1366661044151));
#48327=CARTESIAN_POINT('Ctrl Pts',(0.092882100219491,-0.132461181498507,
-1.12871881310715));
#48328=CARTESIAN_POINT('Ctrl Pts',(0.161655171010697,0.0063761140725619,
-1.12077152179919));
#48329=CARTESIAN_POINT('Ctrl Pts',(0.0821605324921188,0.139365333012824,
-1.11282423049124));
#48330=CARTESIAN_POINT('Ctrl Pts',(-0.0726905197564767,0.1445307492636,
-1.10487693918329));
#48331=CARTESIAN_POINT('Ctrl Pts',(-0.160870912567167,0.0171347201602809,
-1.09692964787534));
#48332=CARTESIAN_POINT('Ctrl Pts',(-0.101502906203354,-0.125977018449545,
-1.08898235656739));
#48333=CARTESIAN_POINT('Ctrl Pts',(0.0509620502732468,-0.153544516597341,
-1.08103506525943));
#48334=CARTESIAN_POINT('Ctrl Pts',(0.156685375111944,-0.0402832765697306,
-1.07308777395149));
#48335=CARTESIAN_POINT('Ctrl Pts',(0.118699213239233,0.10992518329096,-1.06514048264353));
#48336=CARTESIAN_POINT('Ctrl Pts',(-0.0281560948155716,0.159311906240246,
-1.05719319133558));
#48337=CARTESIAN_POINT('Ctrl Pts',(-0.149187053081172,0.0625801273418309,
-1.04924590002763));
#48338=CARTESIAN_POINT('Ctrl Pts',(-0.133385873650668,-0.0915492100217792,
-1.04129860871968));
#48339=CARTESIAN_POINT('Ctrl Pts',(0.00475483761677099,-0.161710978799839,
-1.03335131741172));
#48340=CARTESIAN_POINT('Ctrl Pts',(0.138534482812702,-0.0835538521971371,
-1.02540402610378));
#48341=CARTESIAN_POINT('Ctrl Pts',(0.145252368717955,0.0712376201665093,
-1.01745673479582));
#48342=CARTESIAN_POINT('Ctrl Pts',(0.0187469506794855,0.160691010904112,
-1.00950944348787));
#48343=CARTESIAN_POINT('Ctrl Pts',(-0.124952890626809,0.102761005586597,
-1.00156215217992));
#48344=CARTESIAN_POINT('Ctrl Pts',(-0.154047806219669,-0.0494198598143619,
-0.993614860871969));
#48345=CARTESIAN_POINT('Ctrl Pts',(-0.0418523739097306,-0.156273567641121,
-0.985667569564015));
#48346=CARTESIAN_POINT('Ctrl Pts',(0.108729430886627,-0.11979549242035,
-0.977720278256066));
#48347=CARTESIAN_POINT('Ctrl Pts',(0.159586225024031,0.0265572198797849,
-0.969772986948112));
#48348=CARTESIAN_POINT('Ctrl Pts',(0.0640729162208801,0.148552046610325,
-0.961825695640163));
#48349=CARTESIAN_POINT('Ctrl Pts',(-0.0902071147197211,0.134297154099061,
-0.95387840433221));
#48350=CARTESIAN_POINT('Ctrl Pts',(-0.161750526848092,-0.00313308307082268,
-0.945931113024258));
#48351=CARTESIAN_POINT('Ctrl Pts',(-0.0849387707162987,-0.137689703225653,
-0.937983821716307));
#48352=CARTESIAN_POINT('Ctrl Pts',(0.069777557765129,-0.145959383314327,
-0.930036530408354));
#48353=CARTESIAN_POINT('Ctrl Pts',(0.160494952056057,-0.0203572962273449,
-0.922089239100404));
#48354=CARTESIAN_POINT('Ctrl Pts',(0.104008772540114,0.123916199021204,
-0.914141947792451));
#48355=CARTESIAN_POINT('Ctrl Pts',(-0.0478727002796515,0.154535606618988,
-0.906194656484501));
#48356=CARTESIAN_POINT('Ctrl Pts',(-0.15584604715108,0.0434172630706667,
-0.898247365176548));
#48357=CARTESIAN_POINT('Ctrl Pts',(-0.120879726385485,-0.107522745938403,
-0.890300073868598));
#48358=CARTESIAN_POINT('Ctrl Pts',(0.024955674664485,-0.159844497707004,
-0.882352782560644));
#48359=CARTESIAN_POINT('Ctrl Pts',(0.147902103504972,-0.0655592626862832,
-0.874405491252694));
#48360=CARTESIAN_POINT('Ctrl Pts',(0.135194931216111,0.0888559492585357,
-0.866458199944742));
#48361=CARTESIAN_POINT('Ctrl Pts',(-0.00151101349915643,0.161773811178971,
-0.85851090863679));
#48362=CARTESIAN_POINT('Ctrl Pts',(-0.136831079192702,0.0863151487985995,
-0.85056361732884));
#48363=CARTESIAN_POINT('Ctrl Pts',(-0.146651721963705,-0.0683104793589116,
-0.842616326020886));
#48364=CARTESIAN_POINT('Ctrl Pts',(-0.0219655948865895,-0.160282755736362,
-0.834669034712937));
#48365=CARTESIAN_POINT('Ctrl Pts',(0.122867047870162,-0.105246081603238,
-0.826721743404984));
#48366=CARTESIAN_POINT('Ctrl Pts',(0.155007868747866,0.0463207272331561,
-0.818774452097032));
#48367=CARTESIAN_POINT('Ctrl Pts',(0.0449777867058173,0.155402856628216,
-0.810827160789081));
#48368=CARTESIAN_POINT('Ctrl Pts',(-0.106305249776236,0.121951806116908,
-0.802879869481129));
#48369=CARTESIAN_POINT('Ctrl Pts',(-0.160086698320322,-0.0233516202020928,
-0.794932578173178));
#48370=CARTESIAN_POINT('Ctrl Pts',(-0.0670390172886451,-0.14723728911569,
-0.786985286865226));
#48371=CARTESIAN_POINT('Ctrl Pts',(0.0874958494954061,-0.136079114731987,
-0.779037995557275));
#48372=CARTESIAN_POINT('Ctrl Pts',(0.16178082945128,-0.000111208002141897,
-0.771090704249321));
#48373=CARTESIAN_POINT('Ctrl Pts',(0.0876828480517711,0.135958697046912,
-0.763143412941372));
#48374=CARTESIAN_POINT('Ctrl Pts',(-0.066836532459887,0.147329315052716,
-0.755196121633419));
#48375=CARTESIAN_POINT('Ctrl Pts',(-0.160054443280973,0.0235716849457503,
-0.747248830325469));
#48376=CARTESIAN_POINT('Ctrl Pts',(-0.106472808366821,-0.121805542663896,
-0.739301539017515));
#48377=CARTESIAN_POINT('Ctrl Pts',(0.044764096722905,-0.155464545121215,
-0.731354247709567));
#48378=CARTESIAN_POINT('Ctrl Pts',(0.154944040634522,-0.0465337879074077,
-0.723406956401613));
#48379=CARTESIAN_POINT('Ctrl Pts',(0.12301162381898,0.105077064817125,-0.715459665093662));
#48380=CARTESIAN_POINT('Ctrl Pts',(-0.0217452177773267,0.160312802511157,
-0.70751237378571));
#48381=CARTESIAN_POINT('Ctrl Pts',(-0.146557670288339,0.0685120312413697,
-0.699565082477759));
#48382=CARTESIAN_POINT('Ctrl Pts',(-0.136949615743669,-0.0861269521858602,
-0.691617791169806));
#48383=CARTESIAN_POINT('Ctrl Pts',(-0.00173341832168038,-0.161771580959345,
-0.683670499861855));
#48384=CARTESIAN_POINT('Ctrl Pts',(0.135072644504701,-0.0890417309561679,
-0.675723208553904));
#48385=CARTESIAN_POINT('Ctrl Pts',(0.147992094450622,0.0653558652707012,
-0.667775917245952));
#48386=CARTESIAN_POINT('Ctrl Pts',(0.0251754049154316,0.159810037646288,
-0.659828625938));
#48387=CARTESIAN_POINT('Ctrl Pts',(-0.1207317901348,0.107688829485749,-0.65188133463005));
#48388=CARTESIAN_POINT('Ctrl Pts',(-0.155905589821069,-0.0432029652652273,
-0.643934043322096));
#48389=CARTESIAN_POINT('Ctrl Pts',(-0.0480851102223821,-0.154469645303101,
-0.635986752014146));
#48390=CARTESIAN_POINT('Ctrl Pts',(0.1038383145528,-0.124059072928981,-0.628039460706194));
#48391=CARTESIAN_POINT('Ctrl Pts',(0.160522787545149,0.0201366289109875,
-0.620092169398242));
#48392=CARTESIAN_POINT('Ctrl Pts',(0.0699781564356221,0.145863315357343,
-0.612144878090291));
#48393=CARTESIAN_POINT('Ctrl Pts',(-0.0847493949700018,0.137806346723881,
-0.604197586782338));
#48394=CARTESIAN_POINT('Ctrl Pts',(-0.161746066633085,0.00335545434920126,
-0.596250295474388));
#48395=CARTESIAN_POINT('Ctrl Pts',(-0.0903916608786185,-0.13417301065702,
-0.588303004166436));
#48396=CARTESIAN_POINT('Ctrl Pts',(0.0638686266697115,-0.148639993516177,
-0.580355712858485));
#48397=CARTESIAN_POINT('Ctrl Pts',(0.159549563406843,-0.026776593544546,
-0.572408421550533));
#48398=CARTESIAN_POINT('Ctrl Pts',(0.108894022691339,0.11964589824671,-0.564461130242582));
#48399=CARTESIAN_POINT('Ctrl Pts',(-0.0416374898290139,0.156330958501196,
-0.556513838934629));
#48400=CARTESIAN_POINT('Ctrl Pts',(-0.153979718333526,0.0496315976681452,
-0.548566547626678));
#48401=CARTESIAN_POINT('Ctrl Pts',(-0.125094048127839,-0.102589123537314,
-0.540619256318726));
#48402=CARTESIAN_POINT('Ctrl Pts',(0.01852601534372,-0.160716632308695,
-0.532671965010776));
#48403=CARTESIAN_POINT('Ctrl Pts',(0.145154294138808,-0.0714372454552122,
-0.524724673702822));
#48404=CARTESIAN_POINT('Ctrl Pts',(0.138649221529904,0.0833633163586695,
-0.516777382394872));
#48405=CARTESIAN_POINT('Ctrl Pts',(0.00497715299197124,0.161704289037918,
-0.50883009108692));
#48406=CARTESIAN_POINT('Ctrl Pts',(-0.133259885960394,0.0917325020861564,
-0.500882799778969));
#48407=CARTESIAN_POINT('Ctrl Pts',(-0.149272947104322,-0.0623749661960178,
-0.492935508471017));
#48408=CARTESIAN_POINT('Ctrl Pts',(-0.0283750898365281,-0.159273046752842,
-0.484988217163066));
#48409=CARTESIAN_POINT('Ctrl Pts',(0.118547976184055,-0.110088266803636,
-0.477040925855113));
#48410=CARTESIAN_POINT('Ctrl Pts',(0.15674060839156,0.0400678278199378,
-0.469093634547163));
#48411=CARTESIAN_POINT('Ctrl Pts',(0.0511730947482288,0.153474308987053,
-0.46114634323921));
#48412=CARTESIAN_POINT('Ctrl Pts',(-0.101329617374527,0.126116445350699,
-0.453199051931259));
#48413=CARTESIAN_POINT('Ctrl Pts',(-0.160894317311058,-0.0169135390197523,
-0.445251760623307));
#48414=CARTESIAN_POINT('Ctrl Pts',(-0.0728891515914287,-0.144430677923514,
-0.437304469315356));
#48415=CARTESIAN_POINT('Ctrl Pts',(0.0819688557195135,-0.139478155412228,
-0.429357178007404));
#48416=CARTESIAN_POINT('Ctrl Pts',(0.161646252374504,-0.00659835119118075,
-0.421409886699452));
#48417=CARTESIAN_POINT('Ctrl Pts',(0.0930641197596701,0.132333362227829,
-0.413462595391501));
#48418=CARTESIAN_POINT('Ctrl Pts',(-0.0608750340344286,0.149890891572741,
-0.405515304083549));
#48419=CARTESIAN_POINT('Ctrl Pts',(-0.158980515487525,0.0299707330655217,
-0.397568012775598));
#48420=CARTESIAN_POINT('Ctrl Pts',(-0.111271441743595,-0.117438134340879,
-0.389620721467646));
#48421=CARTESIAN_POINT('Ctrl Pts',(0.0384941370646189,-0.157134498302616,
-0.381673430159694));
#48422=CARTESIAN_POINT('Ctrl Pts',(0.152953468081658,-0.0527094464679463,
-0.373726138851743));
#48423=CARTESIAN_POINT('Ctrl Pts',(0.127126161797411,0.100059922705459,
-0.365778847543791));
#48424=CARTESIAN_POINT('Ctrl Pts',(-0.0152993620706074,0.161055824686338,
-0.35783155623584));
#48425=CARTESIAN_POINT('Ctrl Pts',(-0.143692539469735,0.0743337288577851,
-0.349884264927888));
#48426=CARTESIAN_POINT('Ctrl Pts',(-0.140293065023078,-0.0805661532629814,
-0.341936973619937));
#48427=CARTESIAN_POINT('Ctrl Pts',(-0.00821888593833973,-0.161571962478322,
-0.333989682311984));
#48428=CARTESIAN_POINT('Ctrl Pts',(0.13139353261958,-0.0943863800074581,
-0.326042391004034));
#48429=CARTESIAN_POINT('Ctrl Pts',(0.150493764788252,0.0593689810003615,
-0.318095099696081));
#48430=CARTESIAN_POINT('Ctrl Pts',(0.0315633627925462,0.158671999024367,
-0.310147808388131));
#48431=CARTESIAN_POINT('Ctrl Pts',(-0.116316484309744,0.112443428545168,
-0.302200517080177));
#48432=CARTESIAN_POINT('Ctrl Pts',(-0.157512588629431,-0.0369165757947868,
-0.294253225772227));
#48433=CARTESIAN_POINT('Ctrl Pts',(-0.0542404983500219,-0.152417247986887,
-0.286305934464274));
#48434=CARTESIAN_POINT('Ctrl Pts',(0.0987801671956758,-0.128123095942938,
-0.278358643156324));
#48435=CARTESIAN_POINT('Ctrl Pts',(0.161201138195067,0.0136836467989822,
-0.270411351848371));
#48436=CARTESIAN_POINT('Ctrl Pts',(0.0757708320050786,0.142939952995593,
-0.262464060540421));
#48437=CARTESIAN_POINT('Ctrl Pts',(-0.0791553500289386,0.141093868425444,
-0.254516769232468));
#48438=CARTESIAN_POINT('Ctrl Pts',(-0.16148142681772,0.00983859429043673,
-0.246569477924517));
#48439=CARTESIAN_POINT('Ctrl Pts',(-0.0956991498812775,-0.13044049163145,
-0.238622186616566));
#48440=CARTESIAN_POINT('Ctrl Pts',(0.0578569585295865,-0.151081506137494,
-0.230674895308614));
#48441=CARTESIAN_POINT('Ctrl Pts',(0.158347528374801,-0.0331528188732168,
-0.222727604000663));
#48442=CARTESIAN_POINT('Ctrl Pts',(0.113604109384946,0.115183138854537,
-0.21478031269271));
#48443=CARTESIAN_POINT('Ctrl Pts',(-0.0353353026649132,0.157874841386009,
-0.206833021384759));
#48444=CARTESIAN_POINT('Ctrl Pts',(-0.151865702554914,0.0557660963925229,
-0.198885730076807));
#48445=CARTESIAN_POINT('Ctrl Pts',(-0.129107147668427,-0.0974904794131229,
-0.190938438768856));
#48446=CARTESIAN_POINT('Ctrl Pts',(0.0120665558918105,-0.161330243433346,
-0.182991147460904));
#48447=CARTESIAN_POINT('Ctrl Pts',(0.142172993736196,-0.0772003161421253,
-0.175043856152953));
#48448=CARTESIAN_POINT('Ctrl Pts',(0.141880485927735,0.0777365871248822,
-0.167096564845001));
#48449=CARTESIAN_POINT('Ctrl Pts',(0.0114573118176813,0.161374655912202,
-0.15914927353705));
#48450=CARTESIAN_POINT('Ctrl Pts',(-0.129474332107829,0.0970022946962231,
-0.151201982229098));
#48451=CARTESIAN_POINT('Ctrl Pts',(-0.151654062184562,-0.0563391135504591,
-0.143254690921146));
#48452=CARTESIAN_POINT('Ctrl Pts',(-0.0347389307465692,-0.158007145849288,
-0.135307399613195));
#48453=CARTESIAN_POINT('Ctrl Pts',(0.114038191537599,-0.114753349174383,
-0.127360108305243));
#48454=CARTESIAN_POINT('Ctrl Pts',(0.15822125885756,0.0337504417737982,
-0.119412816997291));
#48455=CARTESIAN_POINT('Ctrl Pts',(0.0572860137252658,0.15129895347779,
-0.11146552568934));
#48456=CARTESIAN_POINT('Ctrl Pts',(-0.096190849571472,0.130078092307543,
-0.103518234381388));
#48457=CARTESIAN_POINT('Ctrl Pts',(-0.161443392134426,-0.0104480133107038,
-0.0955709430734366));
#48458=CARTESIAN_POINT('Ctrl Pts',(-0.0786215350791608,-0.141392191761692,
-0.0876236517654851));
#48459=CARTESIAN_POINT('Ctrl Pts',(0.0763090534835393,-0.142651978679687,
-0.0796763604575335));
#48460=CARTESIAN_POINT('Ctrl Pts',(0.161253470770041,-0.0130765076804255,
-0.071729069149582));
#48461=CARTESIAN_POINT('Ctrl Pts',(0.0982922472958529,0.128498248794366,
-0.0637817778416304));
#48462=CARTESIAN_POINT('Ctrl Pts',(-0.0548090762867236,0.152205495472761,
-0.0558344865336785));
#48463=CARTESIAN_POINT('Ctrl Pts',(-0.157663267928126,0.036332702127111,
-0.0478871952257271));
#48464=CARTESIAN_POINT('Ctrl Pts',(-0.115867512298235,-0.112902967751805,
-0.0399399039177751));
#48465=CARTESIAN_POINT('Ctrl Pts',(0.0321173634886005,-0.158511366575469,
-0.0319926126098238));
#48466=CARTESIAN_POINT('Ctrl Pts',(0.150803302304377,-0.0588783810225519,
-0.0240453213018721));
#48467=CARTESIAN_POINT('Ctrl Pts',(0.130861723774648,0.0950427942614887,
-0.0160980299939207));
#48468=CARTESIAN_POINT('Ctrl Pts',(0.0380135549211517,0.13910682119594,
-0.0107998357886196));
#48469=CARTESIAN_POINT('Ctrl Pts',(-0.00746697525422262,0.136621099781669,
-0.00815073868596909));
#48470=CARTESIAN_POINT('Ctrl Pts',(-0.120752812127176,0.0402994834133023,
-2.94314926131403));
#48471=CARTESIAN_POINT('Ctrl Pts',(-0.13416832315995,0.000101432566926213,
-2.94050016421138));
#48472=CARTESIAN_POINT('Ctrl Pts',(-0.117464253761176,-0.0940473201527993,
-2.93520197000608));
#48473=CARTESIAN_POINT('Ctrl Pts',(0.0157439008632371,-0.149794811235546,
-2.92725467869813));
#48474=CARTESIAN_POINT('Ctrl Pts',(0.13433249399984,-0.0678016115647968,
-2.91930738739018));
#48475=CARTESIAN_POINT('Ctrl Pts',(0.129802517580256,0.0762007396464412,
-2.91136009608222));
#48476=CARTESIAN_POINT('Ctrl Pts',(0.00617326309182846,0.150405521063703,
-2.90341280477427));
#48477=CARTESIAN_POINT('Ctrl Pts',(-0.123093674514204,0.0866119181392443,
-2.89546551346632));
#48478=CARTESIAN_POINT('Ctrl Pts',(-0.139473746844836,-0.0565952056747279,
-2.88751822215837));
#48479=CARTESIAN_POINT('Ctrl Pts',(-0.0279238304536315,-0.147907557093408,
-2.87957093085042));
#48480=CARTESIAN_POINT('Ctrl Pts',(0.109233850025249,-0.103554190495644,
-2.87162363954247));
#48481=CARTESIAN_POINT('Ctrl Pts',(0.146205747724809,0.0357737851326773,
-2.86367634823451));
#48482=CARTESIAN_POINT('Ctrl Pts',(0.0490789294142754,0.142292553953765,
-2.85572905692656));
#48483=CARTESIAN_POINT('Ctrl Pts',(-0.0930618301676024,0.118301676336187,
-2.84778176561861));
#48484=CARTESIAN_POINT('Ctrl Pts',(-0.14984794252219,-0.0141931844243834,
-2.83983447431066));
#48485=CARTESIAN_POINT('Ctrl Pts',(-0.069195614913156,-0.133670557112622,
-2.83188718300271));
#48486=CARTESIAN_POINT('Ctrl Pts',(0.0749218215473602,-0.130547138405,-2.82393989169476));
#48487=CARTESIAN_POINT('Ctrl Pts',(0.150322121943934,-0.00768791359722427,
-2.81599260038681));
#48488=CARTESIAN_POINT('Ctrl Pts',(0.0878491953235926,0.122222593007361,
-2.80804530907885));
#48489=CARTESIAN_POINT('Ctrl Pts',(-0.0551976905231906,0.140032339864175,
-2.80009801777091));
#48490=CARTESIAN_POINT('Ctrl Pts',(-0.147618084592067,0.0294065270266016,
-2.79215072646295));
#48491=CARTESIAN_POINT('Ctrl Pts',(-0.104645372351645,-0.10819051952984,
-2.784203435155));
#48492=CARTESIAN_POINT('Ctrl Pts',(0.0343065114091399,-0.146556833624553,
-2.77625614384705));
#48493=CARTESIAN_POINT('Ctrl Pts',(0.141792975964607,-0.0505034097530179,
-2.76830885253909));
#48494=CARTESIAN_POINT('Ctrl Pts',(0.119229039509039,0.0918709884218048,
-2.76036156123115));
#48495=CARTESIAN_POINT('Ctrl Pts',(-0.0126899916351106,0.149982687191073,
-2.75241426992319));
#48496=CARTESIAN_POINT('Ctrl Pts',(-0.132969952040698,0.0705325047882228,
-2.74446697861524));
#48497=CARTESIAN_POINT('Ctrl Pts',(-0.131291857634228,-0.0736090380752462,
-2.73651968730729));
#48498=CARTESIAN_POINT('Ctrl Pts',(-0.00919483165182608,-0.150237470142918,
-2.72857239599934));
#48499=CARTESIAN_POINT('Ctrl Pts',(0.121335556659434,-0.0890703377050207,
-2.72062510469138));
#48500=CARTESIAN_POINT('Ctrl Pts',(0.14057878395503,0.053790778658821,-2.71267781338343));
#48501=CARTESIAN_POINT('Ctrl Pts',(0.0308852494790753,0.147315795932769,
-2.70473052207548));
#48502=CARTESIAN_POINT('Ctrl Pts',(-0.107135774699351,0.105724964634277,
-2.69678323076753));
#48503=CARTESIAN_POINT('Ctrl Pts',(-0.146893465878803,-0.0328352257365663,
-2.68883593945958));
#48504=CARTESIAN_POINT('Ctrl Pts',(-0.0519226633012332,-0.141279437296261,
-2.68088864815163));
#48505=CARTESIAN_POINT('Ctrl Pts',(0.0906708308417741,-0.120144258296409,
-2.67294135684367));
#48506=CARTESIAN_POINT('Ctrl Pts',(0.150102392668563,0.0111854406376042,
-2.66499406553573));
#48507=CARTESIAN_POINT('Ctrl Pts',(0.0718622809959905,0.132256020419261,
-2.65704677422777));
#48508=CARTESIAN_POINT('Ctrl Pts',(-0.0722888418891832,0.132023352879024,
-2.64909948291982));
#48509=CARTESIAN_POINT('Ctrl Pts',(-0.150137718279179,0.0107008372108558,
-2.64115219161187));
#48510=CARTESIAN_POINT('Ctrl Pts',(-0.0902825210470809,-0.120436326581624,
-2.63320490030392));
#48511=CARTESIAN_POINT('Ctrl Pts',(0.0523784565548806,-0.141111089769806,
-2.62525760899597));
#48512=CARTESIAN_POINT('Ctrl Pts',(0.146998695824624,-0.0323608682354538,
-2.61731031768802));
#48513=CARTESIAN_POINT('Ctrl Pts',(0.106793926001398,0.106070258490779,
-2.60936302638006));
#48514=CARTESIAN_POINT('Ctrl Pts',(-0.031360638297492,0.147215327777602,
-2.60141573507211));
#48515=CARTESIAN_POINT('Ctrl Pts',(-0.140751693369979,0.0533366963785367,
-2.59346844376416));
#48516=CARTESIAN_POINT('Ctrl Pts',(-0.121047396732009,-0.0894615566123041,
-2.58552115245621));
#48517=CARTESIAN_POINT('Ctrl Pts',(0.00967976492882044,-0.150207005555719,
-2.57757386114826));
#48518=CARTESIAN_POINT('Ctrl Pts',(0.131528790717594,-0.073184831621452,
-2.56962656984031));
#48519=CARTESIAN_POINT('Ctrl Pts',(0.132741573409056,0.0709613772131088,
-2.56167927853235));
#48520=CARTESIAN_POINT('Ctrl Pts',(0.012205766825665,0.150022870334127,
-2.5537319872244));
#48521=CARTESIAN_POINT('Ctrl Pts',(-0.119524986855898,0.0914856266535366,
-2.54578469591645));
#48522=CARTESIAN_POINT('Ctrl Pts',(-0.141629207123113,-0.0509608678965643,
-2.5378374046085));
#48523=CARTESIAN_POINT('Ctrl Pts',(-0.0338332331669371,-0.146666815267001,
-2.52989011330055));
#48524=CARTESIAN_POINT('Ctrl Pts',(0.104994077113604,-0.107852149436882,
-2.5219428219926));
#48525=CARTESIAN_POINT('Ctrl Pts',(0.147522387446294,0.0298828976044573,
-2.51399553068464));
#48526=CARTESIAN_POINT('Ctrl Pts',(0.0547453665494287,0.140209797120107,
-2.5060482393767));
#48527=CARTESIAN_POINT('Ctrl Pts',(-0.0882432871882518,0.121938364075071,
-2.49810094806874));
#48528=CARTESIAN_POINT('Ctrl Pts',(-0.150296515405261,-0.00817311593757486,
-2.49015365676079));
#48529=CARTESIAN_POINT('Ctrl Pts',(-0.0745000236469882,-0.130788336038391,
-2.48220636545284));
#48530=CARTESIAN_POINT('Ctrl Pts',(0.0696267775013432,-0.133446447018537,
-2.47425907414489));
#48531=CARTESIAN_POINT('Ctrl Pts',(0.149892937865947,-0.0137094691731059,
-2.46631178283693));
#48532=CARTESIAN_POINT('Ctrl Pts',(0.09267953354884,0.11860162911302,-2.45836449152898));
#48533=CARTESIAN_POINT('Ctrl Pts',(-0.0495381552169006,0.142133083920666,
-2.45041720022103));
#48534=CARTESIAN_POINT('Ctrl Pts',(-0.146320187631405,0.0353021962291781,
-2.44246990891308));
#48535=CARTESIAN_POINT('Ctrl Pts',(-0.108899528537508,-0.103907338775475,
-2.43452261760512));
#48536=CARTESIAN_POINT('Ctrl Pts',(0.0284021522411427,-0.147814614010807,
-2.42657532629718));
#48537=CARTESIAN_POINT('Ctrl Pts',(0.139653803033537,-0.0561485321746081,
-2.41862803498922));
#48538=CARTESIAN_POINT('Ctrl Pts',(0.122817070740355,0.087016145064302,
-2.41068074368128));
#48539=CARTESIAN_POINT('Ctrl Pts',(-0.00666564515458532,0.150370913217171,
-2.40273345237332));
#48540=CARTESIAN_POINT('Ctrl Pts',(-0.130034730833038,0.075807724832447,
-2.39478616106537));
#48541=CARTESIAN_POINT('Ctrl Pts',(-0.134137902833708,-0.0682851769454208,
-2.38683886975742));
#48542=CARTESIAN_POINT('Ctrl Pts',(-0.0152117930586876,-0.149747933939112,
-2.37889157844947));
#48543=CARTESIAN_POINT('Ctrl Pts',(0.117666346194914,-0.0938641216878506,
-2.37094428714152));
#48544=CARTESIAN_POINT('Ctrl Pts',(0.142622669498577,0.0481104615670283,
-2.36299699583356));
#48545=CARTESIAN_POINT('Ctrl Pts',(0.0367676097206484,0.145958847770606,
-2.35504970452561));
#48546=CARTESIAN_POINT('Ctrl Pts',(-0.102810152745931,0.109935957991238,
-2.34710241321766));
#48547=CARTESIAN_POINT('Ctrl Pts',(-0.148091978088299,-0.026918551093764,
-2.33915512190971));
#48548=CARTESIAN_POINT('Ctrl Pts',(-0.0575460521683576,-0.139083767014448,
-2.33120783060176));
#48549=CARTESIAN_POINT('Ctrl Pts',(0.0857802536273329,-0.123683428375524,
-2.32326053929381));
#48550=CARTESIAN_POINT('Ctrl Pts',(0.150430191510887,0.0051575041532583,
-2.31531324798585));
#48551=CARTESIAN_POINT('Ctrl Pts',(0.0771078036908864,0.129268050875151,
-2.3073659566779));
#48552=CARTESIAN_POINT('Ctrl Pts',(-0.0669367104408037,0.134815871329962,
-2.29941866536995));
#48553=CARTESIAN_POINT('Ctrl Pts',(-0.1495878731335,0.0167125874265122,
-2.291471374062));
#48554=CARTESIAN_POINT('Ctrl Pts',(-0.0950392719624149,-0.116719232142552,
-2.28352408275405));
#48555=CARTESIAN_POINT('Ctrl Pts',(0.0466779304989097,-0.14309791462992,
-2.27557679144609));
#48556=CARTESIAN_POINT('Ctrl Pts',(0.145582832016662,-0.0382293262967235,
-2.26762950013815));
#48557=CARTESIAN_POINT('Ctrl Pts',(0.110961333587,0.101702629345004,-2.25968220883019));
#48558=CARTESIAN_POINT('Ctrl Pts',(-0.0254322433356824,0.148354451790324,
-2.25173491752225));
#48559=CARTESIAN_POINT('Ctrl Pts',(-0.138499746378915,0.0589377860126174,
-2.24378762621429));
#48560=CARTESIAN_POINT('Ctrl Pts',(-0.124537349869914,-0.0845357371439527,
-2.23584033490634));
#48561=CARTESIAN_POINT('Ctrl Pts',(0.00364884457439508,-0.150474344326084,
-2.22789304359839));
#48562=CARTESIAN_POINT('Ctrl Pts',(0.128488373252985,-0.0784001295017715,
-2.21994575229044));
#48563=CARTESIAN_POINT('Ctrl Pts',(0.135480284338815,0.0655815135733136,
-2.21199846098248));
#48564=CARTESIAN_POINT('Ctrl Pts',(0.0182117013744718,0.14941277154293,
-2.20405116967453));
#48565=CARTESIAN_POINT('Ctrl Pts',(-0.115760382186509,0.0962048662133375,
-2.19610387836658));
#48566=CARTESIAN_POINT('Ctrl Pts',(-0.143558771529671,-0.0452407060509069,
-2.18815658705863));
#48567=CARTESIAN_POINT('Ctrl Pts',(-0.0396871989844945,-0.145192178177263,
-2.18020929575068));
#48568=CARTESIAN_POINT('Ctrl Pts',(0.100584879932131,-0.111975552225169,
-2.17226200444273));
#48569=CARTESIAN_POINT('Ctrl Pts',(0.148602008725634,0.0239433784124045,
-2.16431471313477));
#48570=CARTESIAN_POINT('Ctrl Pts',(0.0603235937711138,0.137901799849134,
-2.15636742182682));
#48571=CARTESIAN_POINT('Ctrl Pts',(-0.0832827207479992,0.125378749363293,
-2.14842013051887));
#48572=CARTESIAN_POINT('Ctrl Pts',(-0.150503367223278,-0.00213981811093342,
-2.14047283921092));
#48573=CARTESIAN_POINT('Ctrl Pts',(-0.0796845723241252,-0.127695776361688,
-2.13252554790297));
#48574=CARTESIAN_POINT('Ctrl Pts',(0.0642197226054989,-0.136131075054764,
-2.12457825659501));
#48575=CARTESIAN_POINT('Ctrl Pts',(0.149222646773545,-0.0197089841694217,
-2.11663096528707));
#48576=CARTESIAN_POINT('Ctrl Pts',(0.0973607872422648,0.11478989273738,
-2.10868367397911));
#48577=CARTESIAN_POINT('Ctrl Pts',(-0.0437989327332868,0.14400519385952,
-2.10073638267116));
#48578=CARTESIAN_POINT('Ctrl Pts',(-0.144786925531932,0.0411410811975513,
-2.09278909136321));
#48579=CARTESIAN_POINT('Ctrl Pts',(-0.11297851192793,-0.0994570168949558,
-2.08484180005526));
#48580=CARTESIAN_POINT('Ctrl Pts',(0.0224521060265546,-0.148834624002835,
-2.07689450874731));
#48581=CARTESIAN_POINT('Ctrl Pts',(0.137289987547526,-0.0617033361034314,
-2.06894721743936));
#48582=CARTESIAN_POINT('Ctrl Pts',(0.126207542254494,0.0820213304279625,
-2.0609999261314));
#48583=CARTESIAN_POINT('Ctrl Pts',(-0.000630576492705186,0.150517257284272,
-2.05305263482345));
#48584=CARTESIAN_POINT('Ctrl Pts',(-0.126890339895417,0.0809610030095871,
-2.0451053435155));
#48585=CARTESIAN_POINT('Ctrl Pts',(-0.136768178042001,-0.0628514744629297,
-2.03715805220755));
#48586=CARTESIAN_POINT('Ctrl Pts',(-0.021204285262339,-0.149017517942039,
-2.0292107608996));
#48587=CARTESIAN_POINT('Ctrl Pts',(0.11380786137609,-0.0985069188234697,
-2.02126346959164));
#48588=CARTESIAN_POINT('Ctrl Pts',(0.144437136732523,0.0423527555137007,
-2.0133161782837));
#48589=CARTESIAN_POINT('Ctrl Pts',(0.0425908267507145,0.144367114828078,
-2.00536888697574));
#48590=CARTESIAN_POINT('Ctrl Pts',(-0.0983191536380268,0.113970111849532,
-1.99742159566779));
#48591=CARTESIAN_POINT('Ctrl Pts',(-0.14905227423289,-0.0209585761228194,
-1.98947430435984));
#48592=CARTESIAN_POINT('Ctrl Pts',(-0.0630768742790228,-0.136664370990691,
-1.98152701305189));
#48593=CARTESIAN_POINT('Ctrl Pts',(0.0807516930143136,-0.127023645209918,
-1.97357972174394));
#48594=CARTESIAN_POINT('Ctrl Pts',(0.150516013112444,-0.000878728528827487,
-1.96563243043598));
#48595=CARTESIAN_POINT('Ctrl Pts',(0.0822292932154056,0.126072144839324,
-1.95768513912803));
#48596=CARTESIAN_POINT('Ctrl Pts',(-0.061476906720437,0.137391529240996,
-1.94973784782008));
#48597=CARTESIAN_POINT('Ctrl Pts',(-0.148797405673741,0.0226974543034491,
-1.94179055651213));
#48598=CARTESIAN_POINT('Ctrl Pts',(-0.0996431457155294,-0.112814386844085,
-1.93384326520418));
#48599=CARTESIAN_POINT('Ctrl Pts',(0.040902319802603,-0.14485455671762,
-1.92589597389623));
#48600=CARTESIAN_POINT('Ctrl Pts',(0.143932788276891,-0.0440362898747423,
-1.91794868258827));
#48601=CARTESIAN_POINT('Ctrl Pts',(0.114950252286431,0.0971714045714007,
-1.91000139128032));
#48602=CARTESIAN_POINT('Ctrl Pts',(-0.019462938872886,0.149254937531471,
-1.90205409997237));
#48603=CARTESIAN_POINT('Ctrl Pts',(-0.136025013083223,0.0644440701911498,
-1.89410680866442));
#48604=CARTESIAN_POINT('Ctrl Pts',(-0.127826976171915,-0.0794739361667551,
-1.88615951735647));
#48605=CARTESIAN_POINT('Ctrl Pts',(-0.00238794519582686,-0.150499634832894,
-1.87821222604852));
#48606=CARTESIAN_POINT('Ctrl Pts',(0.125241273461417,-0.0834893154173368,
-1.87026493474057));
#48607=CARTESIAN_POINT('Ctrl Pts',(0.138001065974934,0.0600961575882769,
-1.86231764343261));
#48608=CARTESIAN_POINT('Ctrl Pts',(0.0241883411573577,0.14856233210053,
-1.85437035212466));
#48609=CARTESIAN_POINT('Ctrl Pts',(-0.111809569033394,0.100769353672927,
-1.84642306081671));
#48610=CARTESIAN_POINT('Ctrl Pts',(-0.145257411844003,-0.0394477714386299,
-1.83847576950876));
#48611=CARTESIAN_POINT('Ctrl Pts',(-0.0454773252309796,-0.143483989549109,
-1.83052847820081));
#48612=CARTESIAN_POINT('Ctrl Pts',(0.0960138850991289,-0.115918834687312,
-1.82258118689285));
#48613=CARTESIAN_POINT('Ctrl Pts',(0.149442593521154,0.0179653446603165,
-1.8146338955849));
#48614=CARTESIAN_POINT('Ctrl Pts',(0.0658047863707909,0.135371978111378,
-1.80668660427695));
#48615=CARTESIAN_POINT('Ctrl Pts',(-0.0781881883613825,0.12861745436704,
-1.798739312969));
#48616=CARTESIAN_POINT('Ctrl Pts',(-0.150468124092429,0.00389692175933637,
-1.79079202166105));
#48617=CARTESIAN_POINT('Ctrl Pts',(-0.0847409429224701,-0.124397809304279,
-1.7828447303531));
#48618=CARTESIAN_POINT('Ctrl Pts',(0.0587093658982245,-0.138596726956018,
-1.77489743904515));
#48619=CARTESIAN_POINT('Ctrl Pts',(0.148312320858622,-0.0256767959181446,
-1.76695014773719));
#48620=CARTESIAN_POINT('Ctrl Pts',(0.101885429457528,0.110793508976599,
-1.75900285642924));
#48621=CARTESIAN_POINT('Ctrl Pts',(-0.0379892566739397,0.14564566160533,
-1.75105556512129));
#48622=CARTESIAN_POINT('Ctrl Pts',(-0.143020763770612,0.0469137879259792,
-1.74310827381334));
#48623=CARTESIAN_POINT('Ctrl Pts',(-0.116875761663,-0.0948467116076595,
-1.73516098250539));
#48624=CARTESIAN_POINT('Ctrl Pts',(0.0164659440654498,-0.149615223333477,
-1.72721369119744));
#48625=CARTESIAN_POINT('Ctrl Pts',(0.13470533173662,-0.0671588860004383,
-1.71926639988949));
#48626=CARTESIAN_POINT('Ctrl Pts',(0.129395000314167,0.0768945788777685,
-1.71131910858153));
#48627=CARTESIAN_POINT('Ctrl Pts',(0.00540550649454605,0.150421484059394,
-1.70337181727358));
#48628=CARTESIAN_POINT('Ctrl Pts',(-0.123541837176675,0.0859840498819692,
-1.69542452596563));
#48629=CARTESIAN_POINT('Ctrl Pts',(-0.139178452291639,-0.0573166710896298,
-1.68747723465768));
#48630=CARTESIAN_POINT('Ctrl Pts',(-0.0271626689244233,-0.148047397086186,
-1.67952994334973));
#48631=CARTESIAN_POINT('Ctrl Pts',(0.109766308836665,-0.10299126084997,
-1.67158265204177));
#48632=CARTESIAN_POINT('Ctrl Pts',(0.146019266963803,0.0365269221595056,
-1.66363536073383));
#48633=CARTESIAN_POINT('Ctrl Pts',(0.0483455335260618,0.142543157517902,
-1.65568806942587));
#48634=CARTESIAN_POINT('Ctrl Pts',(-0.0936700014541382,0.117820936996251,
-1.64774077811792));
#48635=CARTESIAN_POINT('Ctrl Pts',(-0.149772809610831,-0.0149648878502536,
-1.63979348680997));
#48636=CARTESIAN_POINT('Ctrl Pts',(-0.0685062329278706,-0.134025140989014,
-1.63184619550202));
#48637=CARTESIAN_POINT('Ctrl Pts',(0.0755932377859644,-0.130159535832484,
-1.62389890419406));
#48638=CARTESIAN_POINT('Ctrl Pts',(0.150359719423358,-0.006913547716038,
-1.61595161288612));
#48639=CARTESIAN_POINT('Ctrl Pts',(0.0872185113037171,0.122673443145027,
-1.60800432157816));
#48640=CARTESIAN_POINT('Ctrl Pts',(-0.0559182131953897,0.139746183490383,
-1.60005703027021));
#48641=CARTESIAN_POINT('Ctrl Pts',(-0.147767587420821,0.0286458107744018,
-1.59210973896226));
#48642=CARTESIAN_POINT('Ctrl Pts',(-0.104086736660943,-0.108728071896675,
-1.58416244765431));
#48643=CARTESIAN_POINT('Ctrl Pts',(0.0350609149303666,-0.146378190354091,
-1.57621515634636));
#48644=CARTESIAN_POINT('Ctrl Pts',(0.142051218813405,-0.0497724180718481,
-1.5682678650384));
#48645=CARTESIAN_POINT('Ctrl Pts',(0.118754265651428,0.0924838729546011,
-1.56032057373045));
#48646=CARTESIAN_POINT('Ctrl Pts',(-0.0134623269431637,0.149915336508204,
-1.5523732824225));
#48647=CARTESIAN_POINT('Ctrl Pts',(-0.133331474260487,0.0698466916798358,
-1.54442599111455));
#48648=CARTESIAN_POINT('Ctrl Pts',(-0.130910984049351,-0.074284295933417,
-1.5364786998066));
#48649=CARTESIAN_POINT('Ctrl Pts',(-0.00842089379304925,-0.150282836394643,
-1.52853140849865));
#48650=CARTESIAN_POINT('Ctrl Pts',(0.121792714524754,-0.0884442030648959,
-1.52058411719069));
#48651=CARTESIAN_POINT('Ctrl Pts',(0.140299863467925,0.0545141328278685,
-1.51263682588274));
#48652=CARTESIAN_POINT('Ctrl Pts',(0.0301260723408991,0.147472919996872,
-1.50468953457479));
#48653=CARTESIAN_POINT('Ctrl Pts',(-0.107678902549438,0.105171746742371,
-1.49674224326684));
#48654=CARTESIAN_POINT('Ctrl Pts',(-0.146722395687109,-0.0335913823908467,
-1.48879495195889));
#48655=CARTESIAN_POINT('Ctrl Pts',(-0.0511942980927276,-0.141544997120653,
-1.48084766065094));
#48656=CARTESIAN_POINT('Ctrl Pts',(0.0912884453720831,-0.119675653784055,
-1.47290036934298));
#48657=CARTESIAN_POINT('Ctrl Pts',(0.150042789694782,0.0119584124239118,
-1.46495307803503));
#48658=CARTESIAN_POINT('Ctrl Pts',(0.071180127475677,0.132624401297949,
-1.45700578672708));
#48659=CARTESIAN_POINT('Ctrl Pts',(-0.0729678849318161,0.131649269408037,
-1.44905849541913));
#48660=CARTESIAN_POINT('Ctrl Pts',(-0.150190842703695,0.00992739316471041,
-1.44111120411118));
#48661=CARTESIAN_POINT('Ctrl Pts',(-0.0896610019244564,-0.120899739871496,
-1.43316391280323));
#48662=CARTESIAN_POINT('Ctrl Pts',(0.0531045711647607,-0.140839436552763,
-1.42521662149528));
#48663=CARTESIAN_POINT('Ctrl Pts',(0.147163424442606,-0.0316033047863433,
-1.41726933018732));
#48664=CARTESIAN_POINT('Ctrl Pts',(0.106246181998494,0.106618906286998,
-1.40932203887937));
#48665=CARTESIAN_POINT('Ctrl Pts',(-0.0321184722997344,0.147051848353647,
-1.40137474757142));
#48666=CARTESIAN_POINT('Ctrl Pts',(-0.141024543339304,0.0526110306212836,
-1.39342745626347));
#48667=CARTESIAN_POINT('Ctrl Pts',(-0.120585008750252,-0.0900838389046252,
-1.38548016495552));
#48668=CARTESIAN_POINT('Ctrl Pts',(0.0104532955083284,-0.15015515635538,
-1.37753287364757));
#48669=CARTESIAN_POINT('Ctrl Pts',(0.131903993196282,-0.0725064062408852,
-1.36958558233961));
#48670=CARTESIAN_POINT('Ctrl Pts',(0.132374317675311,0.0716441371438625,
-1.36163829103166));
#48671=CARTESIAN_POINT('Ctrl Pts',(0.0114328943552846,0.15008374760031,
-1.35369099972371));
#48672=CARTESIAN_POINT('Ctrl Pts',(-0.119994608972208,0.0908687855355161,
-1.34574370841576));
#48673=CARTESIAN_POINT('Ctrl Pts',(-0.141364848491819,-0.0516896699348911,
-1.33779641710781));
#48674=CARTESIAN_POINT('Ctrl Pts',(-0.0330773595777369,-0.146839131877228,
-1.32984912579986));
#48675=CARTESIAN_POINT('Ctrl Pts',(0.105548189690026,-0.107309934396826,
-1.3219018344919));
#48676=CARTESIAN_POINT('Ctrl Pts',(0.147366515227844,0.0306423327554257,
-1.31395454318395));
#48677=CARTESIAN_POINT('Ctrl Pts',(0.054022473207671,0.140489909800025,
-1.306007251876));
#48678=CARTESIAN_POINT('Ctrl Pts',(-0.0888701746731883,0.121482239116054,
-1.29805996056805));
#48679=CARTESIAN_POINT('Ctrl Pts',(-0.150252425191737,-0.00894712753314866,
-1.2901126692601));
#48680=CARTESIAN_POINT('Ctrl Pts',(-0.0738253946205713,-0.131170322391194,
-1.28216537795214));
#48681=CARTESIAN_POINT('Ctrl Pts',(0.0703131856699568,-0.133086055948905,
-1.2742180866442));
#48682=CARTESIAN_POINT('Ctrl Pts',(0.149961561852704,-0.0129372459894017,
-1.26627079533624));
#48683=CARTESIAN_POINT('Ctrl Pts',(0.0920674324576578,0.119077412836136,
-1.25832350402829));
#48684=CARTESIAN_POINT('Ctrl Pts',(-0.0502695714039735,0.14187604645589,
-1.25037621272034));
#48685=CARTESIAN_POINT('Ctrl Pts',(-0.146500074907761,0.0345480885015839,
-1.24242892141239));
#48686=CARTESIAN_POINT('Ctrl Pts',(-0.108362896979023,-0.104466860417102,
-1.23448163010444));
#48687=CARTESIAN_POINT('Ctrl Pts',(0.0291631121810312,-0.147666364670528,
-1.22653433879648));
#48688=CARTESIAN_POINT('Ctrl Pts',(0.139941150259236,-0.0554284839339382,
-1.21858704748853));
#48689=CARTESIAN_POINT('Ctrl Pts',(0.122367254666599,0.0876475747094732,
-1.21063975618058));
#48690=CARTESIAN_POINT('Ctrl Pts',(-0.00744005994078389,0.150334586423651,
-1.20269246487263));
#48691=CARTESIAN_POINT('Ctrl Pts',(-0.130423462651932,0.0751369599928877,
-1.19474517356468));
#48692=CARTESIAN_POINT('Ctrl Pts',(-0.133784412664846,-0.0689751643348171,
-1.18679788225673));
#48693=CARTESIAN_POINT('Ctrl Pts',(-0.0144402968072766,-0.149824297746429,
-1.17885059094878));
#48694=CARTESIAN_POINT('Ctrl Pts',(0.118148243685659,-0.0932568221691426,
-1.17090329964082));
#48695=CARTESIAN_POINT('Ctrl Pts',(0.142372979044962,0.0488444183602959,
-1.16295600833287));
#48696=CARTESIAN_POINT('Ctrl Pts',(0.0360153436788049,0.146146287625756,
-1.15500871702492));
#48697=CARTESIAN_POINT('Ctrl Pts',(-0.103375027193893,0.109404963871639,
-1.14706142571697));
#48698=CARTESIAN_POINT('Ctrl Pts',(-0.147951366532389,-0.0276809593094551,
-1.13911413440902));
#48699=CARTESIAN_POINT('Ctrl Pts',(-0.0568289214282981,-0.139378319893695,
-1.13116684310107));
#48700=CARTESIAN_POINT('Ctrl Pts',(0.086416161943652,-0.123239966415207,
-1.12321955179311));
#48701=CARTESIAN_POINT('Ctrl Pts',(0.150401631789964,0.0059322442641027,
-1.11527226048516));
#48702=CARTESIAN_POINT('Ctrl Pts',(0.076440970482352,0.129663489073867,
-1.10732496917721));
#48703=CARTESIAN_POINT('Ctrl Pts',(-0.0676302076740239,0.134469317604654,
-1.09937767786926));
#48704=CARTESIAN_POINT('Ctrl Pts',(-0.149671969083137,0.0159418956799199,
-1.09143038656131));
#48705=CARTESIAN_POINT('Ctrl Pts',(-0.0944368350790274,-0.117207194947022,
-1.08348309525336));
#48706=CARTESIAN_POINT('Ctrl Pts',(0.0474143541003698,-0.142855596293381,
-1.0755358039454));
#48707=CARTESIAN_POINT('Ctrl Pts',(0.145777805603875,-0.037478977579594,
-1.06758851263745));
#48708=CARTESIAN_POINT('Ctrl Pts',(0.110436030296767,0.102272799802216,
-1.0596412213295));
#48709=CARTESIAN_POINT('Ctrl Pts',(-0.0261960231684342,0.148221492157014,
-1.05169393002155));
#48710=CARTESIAN_POINT('Ctrl Pts',(-0.138801475294959,0.0582236448793441,
-1.0437466387136));
#48711=CARTESIAN_POINT('Ctrl Pts',(-0.12410028661232,-0.0851760601920076,
-1.03579934740565));
#48712=CARTESIAN_POINT('Ctrl Pts',(0.00442383211119069,-0.150453554549384,
-1.02785205609769));
#48713=CARTESIAN_POINT('Ctrl Pts',(0.12889047807094,-0.0777372949731165,
-1.01990476478974));
#48714=CARTESIAN_POINT('Ctrl Pts',(0.135140701902402,0.066278450920486,
-1.01195747348179));
#48715=CARTESIAN_POINT('Ctrl Pts',(0.017441891624336,0.149504591179195,
-1.00401018217384));
#48716=CARTESIAN_POINT('Ctrl Pts',(-0.116254361240943,0.0956073525391913,
-0.996062890865889));
#48717=CARTESIAN_POINT('Ctrl Pts',(-0.143323849674872,-0.0459795224145226,
-0.988115599557936));
#48718=CARTESIAN_POINT('Ctrl Pts',(-0.0389388430382602,-0.145394665892303,
-0.980168308249987));
#48719=CARTESIAN_POINT('Ctrl Pts',(0.101160289069005,-0.11145599258258,
-0.972221016942033));
#48720=CARTESIAN_POINT('Ctrl Pts',(0.14847671438377,0.0247084530655609,
-0.964273725634083));
#48721=CARTESIAN_POINT('Ctrl Pts',(0.0596125140502044,0.138210674463686,
-0.95632643432613));
#48722=CARTESIAN_POINT('Ctrl Pts',(-0.0839273941444871,0.12494812875433,
-0.94837914301818));
#48723=CARTESIAN_POINT('Ctrl Pts',(-0.150490349481178,-0.00291497515011473,
-0.940431851710227));
#48724=CARTESIAN_POINT('Ctrl Pts',(-0.0790258031221334,-0.128104507367988,
-0.932484560402276));
#48725=CARTESIAN_POINT('Ctrl Pts',(0.0649200299908625,-0.135798498051631,
-0.924537269094323));
#48726=CARTESIAN_POINT('Ctrl Pts',(0.14932218086414,-0.0189401338186902,
-0.916589977786373));
#48727=CARTESIAN_POINT('Ctrl Pts',(0.0967682568562582,0.115289838373093,
-0.90864268647842));
#48728=CARTESIAN_POINT('Ctrl Pts',(-0.044540067572435,0.143777692107419,
-0.90069539517047));
#48729=CARTESIAN_POINT('Ctrl Pts',(-0.144996907015034,0.0403947932680219,
-0.892748103862517));
#48730=CARTESIAN_POINT('Ctrl Pts',(-0.112464748173748,-0.100037606855164,
-0.884800812554567));
#48731=CARTESIAN_POINT('Ctrl Pts',(0.02321839857327,-0.148717007550534,
-0.876853521246614));
#48732=CARTESIAN_POINT('Ctrl Pts',(0.137605976803818,-0.0609953892926366,
-0.868906229938663));
#48733=CARTESIAN_POINT('Ctrl Pts',(0.125783407592265,0.0826702893521688,
-0.860958938630711));
#48734=CARTESIAN_POINT('Ctrl Pts',(-0.00140582509366957,0.150512012885679,
-0.85301164732276));
#48735=CARTESIAN_POINT('Ctrl Pts',(-0.127305655992913,0.0803063653722841,
-0.845064356014808));
#48736=CARTESIAN_POINT('Ctrl Pts',(-0.136442639912152,-0.0635550814718675,
-0.837117064706856));
#48737=CARTESIAN_POINT('Ctrl Pts',(-0.0204364716174977,-0.149124756478997,
-0.829169773398905));
#48738=CARTESIAN_POINT('Ctrl Pts',(0.114313723324471,-0.0979194313034393,
-0.821222482090953));
#48739=CARTESIAN_POINT('Ctrl Pts',(0.144217077958002,0.0430961343086391,
-0.813275190783001));
#48740=CARTESIAN_POINT('Ctrl Pts',(0.0418466818757667,0.14458456896599,
-0.805327899475051));
#48741=CARTESIAN_POINT('Ctrl Pts',(-0.0989048660443189,0.113462195641756,
-0.797380608167098));
#48742=CARTESIAN_POINT('Ctrl Pts',(-0.14894234749627,-0.0217260095137962,
-0.789433316859148));
#48743=CARTESIAN_POINT('Ctrl Pts',(-0.0623721315610867,-0.136987443116585,
-0.781486025551194));
#48744=CARTESIAN_POINT('Ctrl Pts',(0.0814048722146108,-0.126606039140381,
-0.773538734243244));
#48745=CARTESIAN_POINT('Ctrl Pts',(0.150518542584674,-0.000103466315906723,
-0.765591442935292));
#48746=CARTESIAN_POINT('Ctrl Pts',(0.081578852965405,0.126494004268746,
-0.75764415162734));
#48747=CARTESIAN_POINT('Ctrl Pts',(-0.0621837426065592,0.137073062716691,
-0.749696860319388));
#48748=CARTESIAN_POINT('Ctrl Pts',(-0.148912337874421,0.0219307545667479,
-0.741749569011437));
#48749=CARTESIAN_POINT('Ctrl Pts',(-0.0990607601322656,-0.113326114241646,
-0.733802277703485));
#48750=CARTESIAN_POINT('Ctrl Pts',(0.0416478678079634,-0.144641963047185,
-0.725854986395535));
#48751=CARTESIAN_POINT('Ctrl Pts',(0.144157693205001,-0.0432943628767713,
-0.717907695087582));
#48752=CARTESIAN_POINT('Ctrl Pts',(0.114448234695099,0.0977621805314748,
-0.709960403779631));
#48753=CARTESIAN_POINT('Ctrl Pts',(-0.0202314359441068,0.14915271156346,
-0.702013112471679));
#48754=CARTESIAN_POINT('Ctrl Pts',(-0.136355135594409,0.0637426024266583,
-0.694065821163728));
#48755=CARTESIAN_POINT('Ctrl Pts',(-0.127415940684595,-0.0801312699671765,
-0.686118529855775));
#48756=CARTESIAN_POINT('Ctrl Pts',(-0.00161274732213549,-0.150509937921613,
-0.678171238547825));
#48757=CARTESIAN_POINT('Ctrl Pts',(0.125669633805575,-0.0828431379552073,
-0.670223947239872));
#48758=CARTESIAN_POINT('Ctrl Pts',(0.137689703077396,0.0608061512805342,
-0.662276655931922));
#48759=CARTESIAN_POINT('Ctrl Pts',(0.0234228324190441,0.148684946408714,
-0.654329364623969));
#48760=CARTESIAN_POINT('Ctrl Pts',(-0.112327110426889,0.100192128584226,
-0.646382073316018));
#48761=CARTESIAN_POINT('Ctrl Pts',(-0.145052304653554,-0.0401954136909352,
-0.638434782008066));
#48762=CARTESIAN_POINT('Ctrl Pts',(-0.0447376907093767,-0.143716322653641,
-0.630487490700114));
#48763=CARTESIAN_POINT('Ctrl Pts',(0.0966096652115508,-0.115422766189367,
-0.622540199392163));
#48764=CARTESIAN_POINT('Ctrl Pts',(0.149348078600385,0.0187348281408182,
-0.614592908084211));
#48765=CARTESIAN_POINT('Ctrl Pts',(0.0651066640910347,0.135709117814648,
-0.60664561677626));
#48766=CARTESIAN_POINT('Ctrl Pts',(-0.0788496106682267,0.128213030790797,
-0.598698325468307));
#48767=CARTESIAN_POINT('Ctrl Pts',(-0.150486199761679,0.00312186616959324,
-0.590751034160356));
#48768=CARTESIAN_POINT('Ctrl Pts',(-0.0840990932201657,-0.124832627492329,
-0.582803742852406));
#48769=CARTESIAN_POINT('Ctrl Pts',(0.059422446008062,-0.138292498992215,
-0.574856451544453));
#48770=CARTESIAN_POINT('Ctrl Pts',(0.148442604945667,-0.024912555148708,
-0.566909160236502));
#48771=CARTESIAN_POINT('Ctrl Pts',(0.101313422902309,0.111316812328195,
-0.55896186892855));
#48772=CARTESIAN_POINT('Ctrl Pts',(-0.0387389179991394,0.145448061518017,
-0.551014577620599));
#48773=CARTESIAN_POINT('Ctrl Pts',(-0.1432605016909,0.0461765202496334,
-0.543067286312647));
#48774=CARTESIAN_POINT('Ctrl Pts',(-0.116385692137217,-0.0954474359678359,
-0.535119995004695));
#48775=CARTESIAN_POINT('Ctrl Pts',(0.0172363365850853,-0.149528428963252,
-0.527172703696744));
#48776=CARTESIAN_POINT('Ctrl Pts',(0.135049454733197,-0.0664641794003264,
-0.519225412388791));
#48777=CARTESIAN_POINT('Ctrl Pts',(0.128997229313045,0.0775600231862417,
-0.511278121080841));
#48778=CARTESIAN_POINT('Ctrl Pts',(0.00463067111916099,0.1504473304917,
-0.503330829772888));
#48779=CARTESIAN_POINT('Ctrl Pts',(-0.123983069488452,0.0853465924762928,
-0.495383538464938));
#48780=CARTESIAN_POINT('Ctrl Pts',(-0.138881389851128,-0.0580327659181574,
-0.487436247156985));
#48781=CARTESIAN_POINT('Ctrl Pts',(-0.0263997729668648,-0.148185337852268,
-0.479488955849035));
#48782=CARTESIAN_POINT('Ctrl Pts',(0.110295321529175,-0.102424530342436,
-0.471541664541082));
#48783=CARTESIAN_POINT('Ctrl Pts',(0.145829193847951,0.0372785271805361,
-0.463594373233131));
#48784=CARTESIAN_POINT('Ctrl Pts',(0.0476107068258777,0.14279027614874,
-0.455647081925179));
#48785=CARTESIAN_POINT('Ctrl Pts',(-0.0942756096603422,0.117336915718215,
-0.447699790617227));
#48786=CARTESIAN_POINT('Ctrl Pts',(-0.149693744518164,-0.0157361119474745,
-0.439752499309277));
#48787=CARTESIAN_POINT('Ctrl Pts',(-0.0678150118588708,-0.134376212677966,
-0.431805208001324));
#48788=CARTESIAN_POINT('Ctrl Pts',(0.0762626371868661,-0.129768457401624,
-0.423857916693373));
#48789=CARTESIAN_POINT('Ctrl Pts',(0.150393334019911,-0.00613901046328226,
-0.415910625385421));
#48790=CARTESIAN_POINT('Ctrl Pts',(0.0865855102898376,0.123121045215435,
-0.40796333407747));
#48791=CARTESIAN_POINT('Ctrl Pts',(-0.0566372507405924,0.139456316442247,
-0.400016042769518));
#48792=CARTESIAN_POINT('Ctrl Pts',(-0.147913170996249,0.027884336336504,
-0.392068751461567));
#48793=CARTESIAN_POINT('Ctrl Pts',(-0.103525339184802,-0.109262740738849,
-0.384121460153615));
#48794=CARTESIAN_POINT('Ctrl Pts',(0.0358143880747286,-0.146195663321201,
-0.376174168845663));
#48795=CARTESIAN_POINT('Ctrl Pts',(0.14230569330747,-0.0490401062332962,
-0.368226877537712));
#48796=CARTESIAN_POINT('Ctrl Pts',(0.118276341288589,0.0930943041140431,
-0.36027958622976));
#48797=CARTESIAN_POINT('Ctrl Pts',(-0.0142343050728087,0.149844008642945,
-0.352332294921809));
#48798=CARTESIAN_POINT('Ctrl Pts',(-0.133689459342201,0.069159025642954,
-0.344385003613857));
#48799=CARTESIAN_POINT('Ctrl Pts',(-0.13052663751097,-0.0749575831198715,
-0.336437712305905));
#48800=CARTESIAN_POINT('Ctrl Pts',(-0.00764673254121637,-0.150324215775555,
-0.328490420997954));
#48801=CARTESIAN_POINT('Ctrl Pts',(0.122246641348232,-0.087815722089899,
-0.320543129690002));
#48802=CARTESIAN_POINT('Ctrl Pts',(0.140017220957756,0.0552360407918496,
-0.312595838382051));
#48803=CARTESIAN_POINT('Ctrl Pts',(0.0293660959875197,0.14762613174348,
-0.304648547074098));
#48804=CARTESIAN_POINT('Ctrl Pts',(-0.108219173781323,0.104615738745118,
-0.296701255766147));
#48805=CARTESIAN_POINT('Ctrl Pts',(-0.14654743308991,-0.0343466478982285,
-0.288753964458195));
#48806=CARTESIAN_POINT('Ctrl Pts',(-0.0504645747484669,-0.141806801890957,
-0.280806673150244));
#48807=CARTESIAN_POINT('Ctrl Pts',(0.0919036381071333,-0.119203874390914,
-0.272859381842292));
#48808=CARTESIAN_POINT('Ctrl Pts',(0.149979206228629,0.0127310669651685,
-0.264912090534341));
#48809=CARTESIAN_POINT('Ctrl Pts',(0.0704960856148191,0.132989263777368,
-0.256964799226389));
#48810=CARTESIAN_POINT('Ctrl Pts',(-0.0736449922067076,0.131271693408073,
-0.249017507918438));
#48811=CARTESIAN_POINT('Ctrl Pts',(-0.150239982707076,0.00915368575314346,
-0.241070216610486));
#48812=CARTESIAN_POINT('Ctrl Pts',(-0.0890371041833558,-0.121359945804369,
-0.233122925302535));
#48813=CARTESIAN_POINT('Ctrl Pts',(0.0538292769655777,-0.140564047003862,
-0.225175633994583));
#48814=CARTESIAN_POINT('Ctrl Pts',(0.147324248946552,-0.0308449029238937,
-0.217228342686632));
#48815=CARTESIAN_POINT('Ctrl Pts',(0.105695619402189,0.107164725570485,
-0.209281051378679));
#48816=CARTESIAN_POINT('Ctrl Pts',(-0.0328754542608603,0.146884467812456,
-0.201333760070728));
#48817=CARTESIAN_POINT('Ctrl Pts',(-0.141293652002486,0.0518839690902201,
-0.193386468762776));
#48818=CARTESIAN_POINT('Ctrl Pts',(-0.120119421876057,-0.090703731257369,
-0.185439177454825));
#48819=CARTESIAN_POINT('Ctrl Pts',(0.0112265489861225,-0.150099323874037,
-0.177491886146873));
#48820=CARTESIAN_POINT('Ctrl Pts',(0.132275695981123,-0.0718260569698057,
-0.169544594838922));
#48821=CARTESIAN_POINT('Ctrl Pts',(0.132003550949032,0.0723249957317478,
-0.16159730353097));
#48822=CARTESIAN_POINT('Ctrl Pts',(0.0106597171159664,0.150140644601668,
-0.153650012223019));
#48823=CARTESIAN_POINT('Ctrl Pts',(-0.120461044964925,0.0902495312613209,
-0.145702720915067));
#48824=CARTESIAN_POINT('Ctrl Pts',(-0.141096744864573,-0.0524170959617924,
-0.137755429607115));
#48825=CARTESIAN_POINT('Ctrl Pts',(-0.032320598458173,-0.147007561970503,
-0.129808138299163));
#48826=CARTESIAN_POINT('Ctrl Pts',(0.106099483155384,-0.106764855471587,
-0.121860846991212));
#48827=CARTESIAN_POINT('Ctrl Pts',(0.147206769614965,0.0314009226223516,
-0.11391355568326));
#48828=CARTESIAN_POINT('Ctrl Pts',(0.05329807818182,0.140766356862578,-0.105966264375309));
#48829=CARTESIAN_POINT('Ctrl Pts',(-0.0894945744596918,0.121022774717712,
-0.0980189730673573));
#48830=CARTESIAN_POINT('Ctrl Pts',(-0.150204595788142,-0.00972068039065458,
-0.0900716817594055));
#48831=CARTESIAN_POINT('Ctrl Pts',(-0.0731483385023079,-0.131549249123061,
-0.0821243904514539));
#48832=CARTESIAN_POINT('Ctrl Pts',(0.0709968390897382,-0.132721336641146,
-0.0741770991435026));
#48833=CARTESIAN_POINT('Ctrl Pts',(0.150027895699077,-0.012166193515216,
-0.0662298078355508));
#48834=CARTESIAN_POINT('Ctrl Pts',(0.0914496844930611,0.119552911175019,
-0.0582825165275994));
#48835=CARTESIAN_POINT('Ctrl Pts',(-0.0509935714328428,0.1416097904161,
-0.0503352252196474));
#48836=CARTESIAN_POINT('Ctrl Pts',(-0.146687622928925,0.0338034202871001,
-0.042387933911696));
#48837=CARTESIAN_POINT('Ctrl Pts',(-0.10780145671892,-0.10504328737295,
-0.034440642603744));
#48838=CARTESIAN_POINT('Ctrl Pts',(0.0298815302181444,-0.147476681637548,
-0.0264933512957927));
#48839=CARTESIAN_POINT('Ctrl Pts',(0.140305210183422,-0.0547795936720048,
-0.018546059987841));
#48840=CARTESIAN_POINT('Ctrl Pts',(0.121751854094744,0.0884264404128374,
-0.0105987686798896));
#48841=CARTESIAN_POINT('Ctrl Pts',(0.0353672614029874,0.129422973420375,
-0.00530057447458853));
#48842=CARTESIAN_POINT('Ctrl Pts',(-0.00694716572162589,0.127110294187514,
-0.00265147737193801));
#48843=CARTESIAN_POINT('Ctrl Pts',(-0.111717694016322,0.037284145003949,
-2.93765));
#48844=CARTESIAN_POINT('Ctrl Pts',(-0.124129412884235,9.3843052402752E-5,
-2.93500090289735));
#48845=CARTESIAN_POINT('Ctrl Pts',(-0.108675196282194,-0.0870103938020027,
-2.92970270869205));
#48846=CARTESIAN_POINT('Ctrl Pts',(0.0145658909989512,-0.138586676302172,
-2.92175541738409));
#48847=CARTESIAN_POINT('Ctrl Pts',(0.12428129992797,-0.0627284744858215,
-2.91380812607615));
#48848=CARTESIAN_POINT('Ctrl Pts',(0.120090271076318,0.0704991524890691,
-2.9058608347682));
#48849=CARTESIAN_POINT('Ctrl Pts',(0.00571135947086689,0.139151690834859,
-2.89791354346024));
#48850=CARTESIAN_POINT('Ctrl Pts',(-0.113883405466689,0.0801313327482367,
-2.8899662521523));
#48851=CARTESIAN_POINT('Ctrl Pts',(-0.129037867514933,-0.0523605683294571,
-2.88201896084434));
#48852=CARTESIAN_POINT('Ctrl Pts',(-0.0258344786463291,-0.136840632652599,
-2.87407166953639));
#48853=CARTESIAN_POINT('Ctrl Pts',(0.101060618120367,-0.0958059291879449,
-2.86612437822844));
#48854=CARTESIAN_POINT('Ctrl Pts',(0.13526615819552,0.0330970741869585,
-2.85817708692048));
#48855=CARTESIAN_POINT('Ctrl Pts',(0.0454066843029653,0.131645762308753,
-2.85022979561253));
#48856=CARTESIAN_POINT('Ctrl Pts',(-0.0860986413824693,0.10944996017671,
-2.84228250430459));
#48857=CARTESIAN_POINT('Ctrl Pts',(-0.138635832133158,-0.0131312042072307,
-2.83433521299663));
#48858=CARTESIAN_POINT('Ctrl Pts',(-0.064018173970134,-0.123668891311378,
-2.82638792168868));
#48859=CARTESIAN_POINT('Ctrl Pts',(0.0693159272014078,-0.120779176949328,
-2.81844063038073));
#48860=CARTESIAN_POINT('Ctrl Pts',(0.139074531908459,-0.00711267889956292,
-2.81049333907277));
#48861=CARTESIAN_POINT('Ctrl Pts',(0.0812760328298283,0.113077501111085,
-2.80254604776482));
#48862=CARTESIAN_POINT('Ctrl Pts',(-0.0510676198065011,0.129554664787932,
-2.79459875645687));
#48863=CARTESIAN_POINT('Ctrl Pts',(-0.13657281942522,0.0272062350397427,
-2.78665146514892));
#48864=CARTESIAN_POINT('Ctrl Pts',(-0.0968154652687815,-0.100095353005703,
-2.77870417384097));
#48865=CARTESIAN_POINT('Ctrl Pts',(0.0317395866552255,-0.135590974706457,
-2.77075688253302));
#48866=CARTESIAN_POINT('Ctrl Pts',(0.131183564369451,-0.0467245803901248,
-2.76280959122507));
#48867=CARTESIAN_POINT('Ctrl Pts',(0.110307935021035,0.0849969022889005,
-2.75486229991711));
#48868=CARTESIAN_POINT('Ctrl Pts',(-0.0117404851910752,0.138760494767705,
-2.74691500860916));
#48869=CARTESIAN_POINT('Ctrl Pts',(-0.123020707789416,0.0652550333969683,
-2.73896771730121));
#48870=CARTESIAN_POINT('Ctrl Pts',(-0.12146817386388,-0.0681013704580597,
-2.73102042599325));
#48871=CARTESIAN_POINT('Ctrl Pts',(-0.00850684444458044,-0.138996214030495,
-2.72307313468531));
#48872=CARTESIAN_POINT('Ctrl Pts',(0.112256835707494,-0.0824058053669272,
-2.71512584337735));
#48873=CARTESIAN_POINT('Ctrl Pts',(0.130060222154785,0.0497659776633264,
-2.70717855206941));
#48874=CARTESIAN_POINT('Ctrl Pts',(0.02857431466928,0.136293148986501,-2.69923126076145));
#48875=CARTESIAN_POINT('Ctrl Pts',(-0.0991195276136302,0.0978142789458203,
-2.6912839694535));
#48876=CARTESIAN_POINT('Ctrl Pts',(-0.135902419040663,-0.0303783873615306,
-2.68333667814555));
#48877=CARTESIAN_POINT('Ctrl Pts',(-0.0480376407722225,-0.130708450334381,
-2.67538938683759));
#48878=CARTESIAN_POINT('Ctrl Pts',(0.0838865444021125,-0.111154674162296,
-2.66744209552965));
#48879=CARTESIAN_POINT('Ctrl Pts',(0.138871243492067,0.0103485095922432,
-2.65949480422169));
#48880=CARTESIAN_POINT('Ctrl Pts',(0.0664853114242254,0.122360194853714,
-2.65154751291374));
#48881=CARTESIAN_POINT('Ctrl Pts',(-0.0668799556441275,0.12214493625552,
-2.64360022160579));
#48882=CARTESIAN_POINT('Ctrl Pts',(-0.13890392592561,0.00990016576991218,
-2.63565293029784));
#48883=CARTESIAN_POINT('Ctrl Pts',(-0.0835272892091199,-0.111424888948546,
-2.62770563898989));
#48884=CARTESIAN_POINT('Ctrl Pts',(0.0484593300923006,-0.130552699117355,
-2.61975834768194));
#48885=CARTESIAN_POINT('Ctrl Pts',(0.135999775339708,-0.0299395228313577,
-2.61181105637398));
#48886=CARTESIAN_POINT('Ctrl Pts',(0.0988032571470193,0.0981337367930133,
-2.60386376506603));
#48887=CARTESIAN_POINT('Ctrl Pts',(-0.0290141333502425,0.136200198185447,
-2.59591647375808));
#48888=CARTESIAN_POINT('Ctrl Pts',(-0.130220193924971,0.0493458712960201,
-2.58796918245013));
#48889=CARTESIAN_POINT('Ctrl Pts',(-0.111990236842994,-0.082767752003245,
-2.58002189114218));
#48890=CARTESIAN_POINT('Ctrl Pts',(0.00895549343668939,-0.138968028902788,
-2.57207459983422));
#48891=CARTESIAN_POINT('Ctrl Pts',(0.121687378843393,-0.0677089045107432,
-2.56412730852628));
#48892=CARTESIAN_POINT('Ctrl Pts',(0.122809417189726,0.0656518161922446,
-2.55618001721832));
#48893=CARTESIAN_POINT('Ctrl Pts',(0.011292491656669,0.138797671277311,
-2.54823272591037));
#48894=CARTESIAN_POINT('Ctrl Pts',(-0.110581738624922,0.0846403745414082,
-2.54028543460242));
#48895=CARTESIAN_POINT('Ctrl Pts',(-0.131032049245288,-0.0471478100276249,
-2.53233814329447));
#48896=CARTESIAN_POINT('Ctrl Pts',(-0.0313017206303005,-0.135692727164734,
-2.52439085198651));
#48897=CARTESIAN_POINT('Ctrl Pts',(0.0971380788063926,-0.0997823008635477,
-2.51644356067857));
#48898=CARTESIAN_POINT('Ctrl Pts',(0.136484282651119,0.0276469620217102,
-2.50849626937061));
#48899=CARTESIAN_POINT('Ctrl Pts',(0.0506491401835047,0.129718844114848,
-2.50054897806267));
#48900=CARTESIAN_POINT('Ctrl Pts',(-0.0816406374595077,0.112814539111879,
-2.49260168675471));
#48901=CARTESIAN_POINT('Ctrl Pts',(-0.139050841334286,-0.00756157682283278,
-2.48465439544676));
#48902=CARTESIAN_POINT('Ctrl Pts',(-0.0689256895917136,-0.121002327391366,
-2.47670710413881));
#48903=CARTESIAN_POINT('Ctrl Pts',(0.0644170755712456,-0.123461549863384,
-2.46875981283085));
#48904=CARTESIAN_POINT('Ctrl Pts',(0.138677460778961,-0.0126836821041933,
-2.46081252152291));
#48905=CARTESIAN_POINT('Ctrl Pts',(0.0857449494400285,0.109727469511273,
-2.45286523021495));
#48906=CARTESIAN_POINT('Ctrl Pts',(-0.0458315493375432,0.131498224342159,
-2.444917938907));
#48907=CARTESIAN_POINT('Ctrl Pts',(-0.135372035336123,0.0326607710989214,
-2.43697064759905));
#48908=CARTESIAN_POINT('Ctrl Pts',(-0.10075131165362,-0.0961326537649701,
-2.4290233562911));
#48909=CARTESIAN_POINT('Ctrl Pts',(0.0262770108420999,-0.136754643873708,
-2.42107606498315));
#48910=CARTESIAN_POINT('Ctrl Pts',(0.129204451314017,-0.0519473163932888,
-2.41312877367519));
#48911=CARTESIAN_POINT('Ctrl Pts',(0.113627498086771,0.0805053141001346,
-2.40518148236725));
#48912=CARTESIAN_POINT('Ctrl Pts',(-0.00616689990636303,0.139119672459956,
-2.39723419105929));
#48913=CARTESIAN_POINT('Ctrl Pts',(-0.120305109378322,0.0701355443216227,
-2.38928689975134));
#48914=CARTESIAN_POINT('Ctrl Pts',(-0.124101268705739,-0.0631758579320174,
-2.38133960844339));
#48915=CARTESIAN_POINT('Ctrl Pts',(-0.0140735972308577,-0.138543306517508,
-2.37339231713544));
#48916=CARTESIAN_POINT('Ctrl Pts',(0.10886216750279,-0.086840902842008,
-2.36544502582749));
#48917=CARTESIAN_POINT('Ctrl Pts',(0.13195117753492,0.044510680369643,-2.35749773451953));
#48918=CARTESIAN_POINT('Ctrl Pts',(0.0340165375872002,0.135037732098843,
-2.34955044321158));
#48919=CARTESIAN_POINT('Ctrl Pts',(-0.0951175627623812,0.101710192084987,
-2.34160315190363));
#48920=CARTESIAN_POINT('Ctrl Pts',(-0.13701125466889,-0.0249044175574768,
-2.33365586059568));
#48921=CARTESIAN_POINT('Ctrl Pts',(-0.0532402693961469,-0.128677067243725,
-2.32570856928773));
#48922=CARTESIAN_POINT('Ctrl Pts',(0.0793618960797965,-0.114429032026143,
-2.31776127797978));
#48923=CARTESIAN_POINT('Ctrl Pts',(0.139174515358953,0.00477160291947143,
-2.30981398667182));
#48924=CARTESIAN_POINT('Ctrl Pts',(0.0713383470518088,0.11959579490825,
-2.30186669536388));
#48925=CARTESIAN_POINT('Ctrl Pts',(-0.0619282880767048,0.124728509394241,
-2.29391940405591));
#48926=CARTESIAN_POINT('Ctrl Pts',(-0.138395221981915,0.0154620972832579,
-2.28597211274797));
#48927=CARTESIAN_POINT('Ctrl Pts',(-0.0879281245512522,-0.107985919603993,
-2.27802482144002));
#48928=CARTESIAN_POINT('Ctrl Pts',(0.0431853359348615,-0.132390863279962,
-2.27007753013206));
#48929=CARTESIAN_POINT('Ctrl Pts',(0.134689851066473,-0.0353688837753169,
-2.26213023882412));
#48930=CARTESIAN_POINT('Ctrl Pts',(0.102658845743989,0.0940929078641549,
-2.25418294751616));
#48931=CARTESIAN_POINT('Ctrl Pts',(-0.0235293201795658,0.137254089234922,
-2.24623565620821));
#48932=CARTESIAN_POINT('Ctrl Pts',(-0.128136744931471,0.0545278691880376,
-2.23828836490026));
#48933=CARTESIAN_POINT('Ctrl Pts',(-0.115219060337234,-0.0782104983670698,
-2.23034107359231));
#48934=CARTESIAN_POINT('Ctrl Pts',(0.00337582615670157,-0.139215364516925,
-2.22239378228436));
#48935=CARTESIAN_POINT('Ctrl Pts',(0.118874455301411,-0.0725339768426726,
-2.21444649097641));
#48936=CARTESIAN_POINT('Ctrl Pts',(0.125343208860993,0.0606744914461575,
-2.20649919966845));
#48937=CARTESIAN_POINT('Ctrl Pts',(0.0168490426502724,0.138233222061811,
-2.19855190836051));
#48938=CARTESIAN_POINT('Ctrl Pts',(-0.107098813919995,0.0890065052496212,
-2.19060461705255));
#48939=CARTESIAN_POINT('Ctrl Pts',(-0.132817237367694,-0.0418556492941425,
-2.1826573257446));
#48940=CARTESIAN_POINT('Ctrl Pts',(-0.0367176736873534,-0.134328427217807,
-2.17471003443665));
#48941=CARTESIAN_POINT('Ctrl Pts',(0.093058792097453,-0.103597177245249,
-2.16676274312869));
#48942=CARTESIAN_POINT('Ctrl Pts',(0.137483123155237,0.022151856971875,
-2.15881545182074));
#48943=CARTESIAN_POINT('Ctrl Pts',(0.0558099863031745,0.127583538705665,
-2.1508681605128));
#48944=CARTESIAN_POINT('Ctrl Pts',(-0.0770512367328716,0.115997503584152,
-2.14292086920484));
#48945=CARTESIAN_POINT('Ctrl Pts',(-0.139242215826564,-0.00197970996083189,
-2.13497357789689));
#48946=CARTESIAN_POINT('Ctrl Pts',(-0.0737223134758439,-0.118141163087173,
-2.12702628658893));
#48947=CARTESIAN_POINT('Ctrl Pts',(0.0594145941073171,-0.125945305299099,
-2.11907899528099));
#48948=CARTESIAN_POINT('Ctrl Pts',(0.138057323045987,-0.0182342938771007,
-2.11113170397303));
#48949=CARTESIAN_POINT('Ctrl Pts',(0.0900759365079238,0.106200939647636,
-2.10318441266508));
#48950=CARTESIAN_POINT('Ctrl Pts',(-0.0405217541450246,0.133230256926986,
-2.09523712135713));
#48951=CARTESIAN_POINT('Ctrl Pts',(-0.133953496893346,0.0380627717049713,
-2.08728983004918));
#48952=CARTESIAN_POINT('Ctrl Pts',(-0.104525092241263,-0.0920153194407107,
-2.07934253874123));
#48953=CARTESIAN_POINT('Ctrl Pts',(0.0207721664357911,-0.137698333400896,
-2.07139524743328));
#48954=CARTESIAN_POINT('Ctrl Pts',(0.127017504190175,-0.0570864918270448,
-2.06344795612532));
#48955=CARTESIAN_POINT('Ctrl Pts',(0.116764283495866,0.0758842277388233,
-2.05550066481737));
#48956=CARTESIAN_POINT('Ctrl Pts',(-0.000583394708775192,0.139255066588021,
-2.04755337350942));
#48957=CARTESIAN_POINT('Ctrl Pts',(-0.117395991996717,0.0749032374662622,
-2.03960608220147));
#48958=CARTESIAN_POINT('Ctrl Pts',(-0.12653473816887,-0.058148722740537,
-2.03165879089352));
#48959=CARTESIAN_POINT('Ctrl Pts',(-0.0196177116792869,-0.137867542620766,
-2.02371149958557));
#48960=CARTESIAN_POINT('Ctrl Pts',(0.105292387066522,-0.0911363107968193,
-2.01576420827761));
#48961=CARTESIAN_POINT('Ctrl Pts',(0.133629880429484,0.039183784608208,
-2.00781691696966));
#48962=CARTESIAN_POINT('Ctrl Pts',(0.0394040425810417,0.133565097791645,
-1.99986962566171));
#48963=CARTESIAN_POINT('Ctrl Pts',(-0.0909625948131785,0.105442497431889,
-1.99192233435376));
#48964=CARTESIAN_POINT('Ctrl Pts',(-0.137899698332905,-0.019390387296652,
-1.98397504304581));
#48965=CARTESIAN_POINT('Ctrl Pts',(-0.058357257409372,-0.126438698298729,
-1.97602775173786));
#48966=CARTESIAN_POINT('Ctrl Pts',(0.0747095887255279,-0.117519322974067,
-1.9680804604299));
#48967=CARTESIAN_POINT('Ctrl Pts',(0.139253915509176,-0.000812979202544665,
-1.96013316912196));
#48968=CARTESIAN_POINT('Ctrl Pts',(0.0760766300741984,0.116639016955623,
-1.952185877814));
#48969=CARTESIAN_POINT('Ctrl Pts',(-0.0568770046268523,0.127111448203918,
-1.94423858650605));
#48970=CARTESIAN_POINT('Ctrl Pts',(-0.137663899868222,0.0209991569567163,
-1.9362912951981));
#48971=CARTESIAN_POINT('Ctrl Pts',(-0.0921875214976232,-0.104373247529939,
-1.92834400389015));
#48972=CARTESIAN_POINT('Ctrl Pts',(0.037841875214064,-0.134016067693779,
-1.92039671258219));
#48973=CARTESIAN_POINT('Ctrl Pts',(0.133163268965518,-0.0407413514532521,
-1.91244942127425));
#48974=CARTESIAN_POINT('Ctrl Pts',(0.106349300573725,0.0899007240643813,
-1.90450212996629));
#48975=CARTESIAN_POINT('Ctrl Pts',(-0.0180066584898106,0.138087197704393,
-1.89655483865834));
#48976=CARTESIAN_POINT('Ctrl Pts',(-0.125847179229191,0.0596221552770135,
-1.88860754735039));
#48977=CARTESIAN_POINT('Ctrl Pts',(-0.118262546100927,-0.0735274378007737,
-1.88066025604244));
#48978=CARTESIAN_POINT('Ctrl Pts',(-0.00220927137030462,-0.139238762705767,
-1.87271296473448));
#48979=CARTESIAN_POINT('Ctrl Pts',(0.115870314076337,-0.077242373317187,
-1.86476567342653));
#48980=CARTESIAN_POINT('Ctrl Pts',(0.127675377417112,0.0555995676351779,
-1.85681838211858));
#48981=CARTESIAN_POINT('Ctrl Pts',(0.0223784908076123,0.137446415264255,
-1.84887109081063));
#48982=CARTESIAN_POINT('Ctrl Pts',(-0.103443613455673,0.0932294629130393,
-1.84092379950268));
#48983=CARTESIAN_POINT('Ctrl Pts',(-0.134388779889457,-0.0364961608891077,
-1.83297650819473));
#48984=CARTESIAN_POINT('Ctrl Pts',(-0.0420745638576578,-0.132748050818114,
-1.82502921688678));
#48985=CARTESIAN_POINT('Ctrl Pts',(0.0888298139634637,-0.107245410489387,
-1.81708192557882));
#48986=CARTESIAN_POINT('Ctrl Pts',(0.13826081266264,0.0166211191466418,
-1.80913463427087));
#48987=CARTESIAN_POINT('Ctrl Pts',(0.0608810582468267,0.125243006457714,
-1.80118734296292));
#48988=CARTESIAN_POINT('Ctrl Pts',(-0.072337893827657,0.118993878146731,
-1.79324005165497));
#48989=CARTESIAN_POINT('Ctrl Pts',(-0.139209609701381,0.00360534139989891,
-1.78529276034702));
#48990=CARTESIAN_POINT('Ctrl Pts',(-0.078400349981893,-0.115089960650516,
-1.77734546903907));
#48991=CARTESIAN_POINT('Ctrl Pts',(0.054316540209444,-0.128226469106407,
-1.76939817773111));
#48992=CARTESIAN_POINT('Ctrl Pts',(0.137215110676543,-0.0237555745425038,
-1.76145088642316));
#48993=CARTESIAN_POINT('Ctrl Pts',(0.0942620302777797,0.102503578316717,
-1.75350359511521));
#48994=CARTESIAN_POINT('Ctrl Pts',(-0.0351467769424353,0.13474797954099,
-1.74555630380726));
#48995=CARTESIAN_POINT('Ctrl Pts',(-0.132319485098849,0.0434035457422106,
-1.73760901249931));
#48996=CARTESIAN_POINT('Ctrl Pts',(-0.108130737076674,-0.0877499721884613,
-1.72966172119136));
#48997=CARTESIAN_POINT('Ctrl Pts',(0.0152339085805741,-0.138420525750985,
-1.72171442988341));
#48998=CARTESIAN_POINT('Ctrl Pts',(0.124626240732756,-0.062133839738435,
-1.71376713857545));
#48999=CARTESIAN_POINT('Ctrl Pts',(0.11971324557739,0.0711410764126323,
-1.7058198472675));
#49000=CARTESIAN_POINT('Ctrl Pts',(0.00500104891906081,0.139166459427298,
-1.69787255595955));
#49001=CARTESIAN_POINT('Ctrl Pts',(-0.114298035141258,0.0795504436358992,
-1.6899252646516));
#49002=CARTESIAN_POINT('Ctrl Pts',(-0.128764667860552,-0.0530280513556949,
-1.68197797334364));
#49003=CARTESIAN_POINT('Ctrl Pts',(-0.0251302696981556,-0.136970009362336,
-1.6740306820357));
#49004=CARTESIAN_POINT('Ctrl Pts',(0.101553236631872,-0.0952851197690979,
-1.66608339072774));
#49005=CARTESIAN_POINT('Ctrl Pts',(0.135093630531518,0.0337938590521173,
-1.65813609941979));
#49006=CARTESIAN_POINT('Ctrl Pts',(0.0447281634802288,0.131877614899218,
-1.65018880811184));
#49007=CARTESIAN_POINT('Ctrl Pts',(-0.0866613073154762,0.109005191317629,
-1.64224151680389));
#49008=CARTESIAN_POINT('Ctrl Pts',(-0.138566320910571,-0.0138451662730742,
-1.63429422549594));
#49009=CARTESIAN_POINT('Ctrl Pts',(-0.0633803737869685,-0.123996944068975,
-1.62634693418799));
#49010=CARTESIAN_POINT('Ctrl Pts',(0.0699371058934867,-0.120420576061834,
-1.61839964288003));
#49011=CARTESIAN_POINT('Ctrl Pts',(0.139109316222199,-0.00639625359196896,
-1.61045235157208));
#49012=CARTESIAN_POINT('Ctrl Pts',(0.0806925386394054,0.113494617175214,
-1.60250506026413));
#49013=CARTESIAN_POINT('Ctrl Pts',(-0.051734230629111,0.129289919564653,
-1.59455776895618));
#49014=CARTESIAN_POINT('Ctrl Pts',(-0.136711135966119,0.0265024380515037,
-1.58661047764823));
#49015=CARTESIAN_POINT('Ctrl Pts',(-0.0962986285172303,-0.100592683956246,
-1.57866318634028));
#49016=CARTESIAN_POINT('Ctrl Pts',(0.0324375432515528,-0.135425698106468,
-1.57071589503233));
#49017=CARTESIAN_POINT('Ctrl Pts',(0.131422484648456,-0.0460482838838423,
-1.56276860372437));
#49018=CARTESIAN_POINT('Ctrl Pts',(0.109868685287492,0.0855639288077546,
-1.55482131241642));
#49019=CARTESIAN_POINT('Ctrl Pts',(-0.0124550318596216,0.138698183481963,
-1.54687402110847));
#49020=CARTESIAN_POINT('Ctrl Pts',(-0.123355179740992,0.0646205350557252,
-1.53892672980052));
#49021=CARTESIAN_POINT('Ctrl Pts',(-0.121115798479285,-0.0687261033272357,
-1.53097943849257));
#49022=CARTESIAN_POINT('Ctrl Pts',(-0.00779081513336725,-0.139038185831728,
-1.52303214718461));
#49023=CARTESIAN_POINT('Ctrl Pts',(0.112679787534581,-0.0818265201568669,
-1.51508485587666));
#49024=CARTESIAN_POINT('Ctrl Pts',(0.129802171405619,0.0504352081209822,
-1.50713756456871));
#49025=CARTESIAN_POINT('Ctrl Pts',(0.0278719416335478,0.136438516517136,
-1.49919027326076));
#49026=CARTESIAN_POINT('Ctrl Pts',(-0.0996220168716355,0.0973024546157401,
-1.49124298195281));
#49027=CARTESIAN_POINT('Ctrl Pts',(-0.135744148877059,-0.0310779659157952,
-1.48329569064486));
#49028=CARTESIAN_POINT('Ctrl Pts',(-0.0473637742173777,-0.130954140109069,
-1.47534839933691));
#49029=CARTESIAN_POINT('Ctrl Pts',(0.0844579470046824,-0.110721132163533,
-1.46740110802895));
#49030=CARTESIAN_POINT('Ctrl Pts',(0.138816100206623,0.0110636451156712,
-1.459453816721));
#49031=CARTESIAN_POINT('Ctrl Pts',(0.0658541988487744,0.122701012277025,
-1.45150652541305));
#49032=CARTESIAN_POINT('Ctrl Pts',(-0.0675081904779539,0.121798842926412,
-1.4435592341051));
#49033=CARTESIAN_POINT('Ctrl Pts',(-0.138953075407915,0.00918459332266326,
-1.43561194279715));
#49034=CARTESIAN_POINT('Ctrl Pts',(-0.0829522741685301,-0.111853628148976,
-1.4276646514892));
#49035=CARTESIAN_POINT('Ctrl Pts',(0.0491311144456285,-0.130301371877472,
-1.41971736018124));
#49036=CARTESIAN_POINT('Ctrl Pts',(0.136152178426768,-0.0292386427432272,
-1.41177006887329));
#49037=CARTESIAN_POINT('Ctrl Pts',(0.0982964971317635,0.0986413329768289,
-1.40382277756534));
#49038=CARTESIAN_POINT('Ctrl Pts',(-0.0297152637478395,0.136048950823653,
-1.39587548625739));
#49039=CARTESIAN_POINT('Ctrl Pts',(-0.130472628372239,0.0486745022107058,
-1.38792819494944));
#49040=CARTESIAN_POINT('Ctrl Pts',(-0.111562446233792,-0.0833434731106928,
-1.37998090364148));
#49041=CARTESIAN_POINT('Ctrl Pts',(0.00967114594259312,-0.13892005922824,
-1.37203361233354));
#49042=CARTESIAN_POINT('Ctrl Pts',(0.122034507452407,-0.0670812411234985,
-1.36408632102558));
#49043=CARTESIAN_POINT('Ctrl Pts',(0.122469640724355,0.0662834898045348,
-1.35613902971763));
#49044=CARTESIAN_POINT('Ctrl Pts',(0.0105774480180276,0.138853993508456,
-1.34819173840968));
#49045=CARTESIAN_POINT('Ctrl Pts',(-0.111016222087204,0.0840696874819043,
-1.34024444710173));
#49046=CARTESIAN_POINT('Ctrl Pts',(-0.130787470786524,-0.0478220807272631,
-1.33229715579378));
#49047=CARTESIAN_POINT('Ctrl Pts',(-0.0306024039612664,-0.135852150485784,
-1.32434986448582));
#49048=CARTESIAN_POINT('Ctrl Pts',(0.097650730877784,-0.0992806561161591,
-1.31640257317787));
#49049=CARTESIAN_POINT('Ctrl Pts',(0.136340073298976,0.0283495737648783,
-1.30845528186992));
#49050=CARTESIAN_POINT('Ctrl Pts',(0.0499803360725424,0.129977997853083,
-1.30050799056197));
#49051=CARTESIAN_POINT('Ctrl Pts',(-0.0822206191840827,0.112392542905687,
-1.29256069925402));
#49052=CARTESIAN_POINT('Ctrl Pts',(-0.139010050093927,-0.00827767435361591,
-1.28461340794607));
#49053=CARTESIAN_POINT('Ctrl Pts',(-0.0683015385030549,-0.121355732282971,
-1.27666611663811));
#49054=CARTESIAN_POINT('Ctrl Pts',(0.0650521244483742,-0.123128124425631,
-1.26871882533016));
#49055=CARTESIAN_POINT('Ctrl Pts',(0.138740950095853,-0.0119692391704875,
-1.26077153402221));
#49056=CARTESIAN_POINT('Ctrl Pts',(0.0851786477431396,0.110167653548901,
-1.25282424271426));
#49057=CARTESIAN_POINT('Ctrl Pts',(-0.0465082385868169,0.131260419256424,
-1.24487695140631));
#49058=CARTESIAN_POINT('Ctrl Pts',(-0.135538462861439,0.0319630881639851,
-1.23692966009836));
#49059=CARTESIAN_POINT('Ctrl Pts',(-0.100254832613553,-0.0966503101777165,
-1.22898236879041));
#49060=CARTESIAN_POINT('Ctrl Pts',(0.0269810332845223,-0.136617487031199,
-1.22103507748245));
#49061=CARTESIAN_POINT('Ctrl Pts',(0.12947029828579,-0.0512811445036981,
-1.2130877861745));
#49062=CARTESIAN_POINT('Ctrl Pts',(0.113211338714528,0.0810894981257437,
-1.20514049486655));
#49063=CARTESIAN_POINT('Ctrl Pts',(-0.00688337045973726,0.139086063755268,
-1.1971932035586));
#49064=CARTESIAN_POINT('Ctrl Pts',(-0.120664755018308,0.0695149682887939,
-1.18924591225065));
#49065=CARTESIAN_POINT('Ctrl Pts',(-0.123774227820918,-0.0638142182209893,
-1.18129862094269));
#49066=CARTESIAN_POINT('Ctrl Pts',(-0.0133598268380069,-0.138613956536415,
-1.17335132963475));
#49067=CARTESIAN_POINT('Ctrl Pts',(0.10930800785607,-0.0862790434483248,
-1.16540403832679));
#49068=CARTESIAN_POINT('Ctrl Pts',(0.131720169733078,0.0451897201286931,
-1.15745674701884));
#49069=CARTESIAN_POINT('Ctrl Pts',(0.0333205585370974,0.135211147094447,
-1.14950945571089));
#49070=CARTESIAN_POINT('Ctrl Pts',(-0.0956401714670842,0.101218928672295,
-1.14156216440294));
#49071=CARTESIAN_POINT('Ctrl Pts',(-0.136881164126884,-0.0256097799109962,
-1.13361487309499));
#49072=CARTESIAN_POINT('Ctrl Pts',(-0.0525767967102828,-0.128949580718614,
-1.12566758178704));
#49073=CARTESIAN_POINT('Ctrl Pts',(0.0799502236678128,-0.114018751331906,
-1.11772029047908));
#49074=CARTESIAN_POINT('Ctrl Pts',(0.13914809256923,0.00548837445564355,
-1.10977299917113));
#49075=CARTESIAN_POINT('Ctrl Pts',(0.0707214084725853,0.11996164513491,
-1.10182570786318));
#49076=CARTESIAN_POINT('Ctrl Pts',(-0.0625698955915714,0.124407885945709,
-1.09387841655523));
#49077=CARTESIAN_POINT('Ctrl Pts',(-0.138473025599107,0.0147490711995586,
-1.08593112524728));
#49078=CARTESIAN_POINT('Ctrl Pts',(-0.0873707639547012,-0.108437371444499,
-1.07798383393932));
#49079=CARTESIAN_POINT('Ctrl Pts',(0.043866657927493,-0.132166675989422,
-1.07003654263137));
#49080=CARTESIAN_POINT('Ctrl Pts',(0.134870236095805,-0.0346746785894572,
-1.06208925132342));
#49081=CARTESIAN_POINT('Ctrl Pts',(0.102172847354302,0.0946204163134727,
-1.05414196001547));
#49082=CARTESIAN_POINT('Ctrl Pts',(-0.0242359515212969,0.137131078073783,
-1.04619466870752));
#49083=CARTESIAN_POINT('Ctrl Pts',(-0.128415897508745,0.0538671624168572,
-1.03824737739957));
#49084=CARTESIAN_POINT('Ctrl Pts',(-0.114814699573973,-0.078802910362236,
-1.03030008609162));
#49085=CARTESIAN_POINT('Ctrl Pts',(0.00409282660561049,-0.13919613029893,
-1.02235279478367));
#49086=CARTESIAN_POINT('Ctrl Pts',(0.119246473329177,-0.0719207377490957,
-1.01440550347571));
#49087=CARTESIAN_POINT('Ctrl Pts',(0.12502903508685,0.0613192816744626,
-1.00645821216776));
#49088=CARTESIAN_POINT('Ctrl Pts',(0.0161368325691865,0.138318171454277,
-0.998510920859808));
#49089=CARTESIAN_POINT('Ctrl Pts',(-0.107555831855076,0.0884536994917849,
-0.990563629551857));
#49090=CARTESIAN_POINT('Ctrl Pts',(-0.132599893130074,-0.0425391850146832,
-0.982616338243906));
#49091=CARTESIAN_POINT('Ctrl Pts',(-0.0360253121667897,-0.134515764143485,
-0.974669046935953));
#49092=CARTESIAN_POINT('Ctrl Pts',(0.0935911472513838,-0.103116492744809,
-0.966721755628004));
#49093=CARTESIAN_POINT('Ctrl Pts',(0.13736720374351,0.0228596862513367,
-0.958774464320049));
#49094=CARTESIAN_POINT('Ctrl Pts',(0.0551521118795285,0.127869302317047,
-0.950827173012101));
#49095=CARTESIAN_POINT('Ctrl Pts',(-0.077647673569253,0.115599103409599,
-0.942879881704147));
#49096=CARTESIAN_POINT('Ctrl Pts',(-0.139230172114263,-0.00269686722940675,
-0.934932590396197));
#49097=CARTESIAN_POINT('Ctrl Pts',(-0.0731128355279682,-0.118519311510323,
-0.926985299088244));
#49098=CARTESIAN_POINT('Ctrl Pts',(0.0600625022165961,-0.125637612788934,
-0.919038007780293));
#49099=CARTESIAN_POINT('Ctrl Pts',(0.138149409672222,-0.0175229714100354,
-0.911090716472342));
#49100=CARTESIAN_POINT('Ctrl Pts',(0.0895277411724023,0.106663477724982,
-0.903143425164389));
#49101=CARTESIAN_POINT('Ctrl Pts',(-0.0412074348652185,0.133019777595849,
-0.895196133856439));
#49102=CARTESIAN_POINT('Ctrl Pts',(-0.134147766878989,0.0373723234653771,
-0.887248842548486));
#49103=CARTESIAN_POINT('Ctrl Pts',(-0.104049769962011,-0.0925524677719242,
-0.879301551240536));
#49104=CARTESIAN_POINT('Ctrl Pts',(0.0214811224820551,-0.137589517394064,
-0.871354259932582));
#49105=CARTESIAN_POINT('Ctrl Pts',(0.127309850102664,-0.0564315158989901,
-0.863406968624633));
#49106=CARTESIAN_POINT('Ctrl Pts',(0.116371883968419,0.0764846294458023,
-0.855459677316679));
#49107=CARTESIAN_POINT('Ctrl Pts',(-0.0013006366881828,0.139250214592387,
-0.847512386008729));
#49108=CARTESIAN_POINT('Ctrl Pts',(-0.117780232793124,0.074297581945969,
-0.839565094700777));
#49109=CARTESIAN_POINT('Ctrl Pts',(-0.126233557860599,-0.0587996835848236,
-0.831617803392825));
#49110=CARTESIAN_POINT('Ctrl Pts',(-0.0189073483484057,-0.137966757221631,
-0.823670512084875));
#49111=CARTESIAN_POINT('Ctrl Pts',(0.105760398778781,-0.0905927810036414,
-0.81572322077692));
#49112=CARTESIAN_POINT('Ctrl Pts',(0.133426287168139,0.0398715413841222,
-0.807775929468972));
#49113=CARTESIAN_POINT('Ctrl Pts',(0.038715577045716,0.133766281303764,
-0.799828638161018));
#49114=CARTESIAN_POINT('Ctrl Pts',(-0.0915044823124013,0.104972585166604,
-0.791881346853068));
#49115=CARTESIAN_POINT('Ctrl Pts',(-0.137797996672218,-0.0201003988254995,
-0.783934055545116));
#49116=CARTESIAN_POINT('Ctrl Pts',(-0.0577052458335282,-0.126737597117481,
-0.775986764237163));
#49117=CARTESIAN_POINT('Ctrl Pts',(0.0753138949338155,-0.117132963548775,
-0.768039472929213));
#49118=CARTESIAN_POINT('Ctrl Pts',(0.139256255718067,-9.57246296715326E-5,
-0.760092181621259));
#49119=CARTESIAN_POINT('Ctrl Pts',(0.075474857879039,0.117029311490581,
-0.75214489031331));
#49120=CARTESIAN_POINT('Ctrl Pts',(-0.0575309527532313,0.126816810380666,
-0.744197599005357));
#49121=CARTESIAN_POINT('Ctrl Pts',(-0.13777023246787,0.0202898241877454,
-0.736250307697407));
#49122=CARTESIAN_POINT('Ctrl Pts',(-0.0916487118977105,-0.104846685819395,
-0.728303016389454));
#49123=CARTESIAN_POINT('Ctrl Pts',(0.0385316388930217,-0.133819380973154,
-0.720355725081504));
#49124=CARTESIAN_POINT('Ctrl Pts',(0.13337134577548,-0.0400549378461348,
-0.712408433773551));
#49125=CARTESIAN_POINT('Ctrl Pts',(0.105884845571219,0.0904472962458246,
-0.7044611424656));
#49126=CARTESIAN_POINT('Ctrl Pts',(-0.018717654110887,0.137992620615763,
-0.696513851157648));
#49127=CARTESIAN_POINT('Ctrl Pts',(-0.126152600900479,0.058973173611947,
-0.688566559849696));
#49128=CARTESIAN_POINT('Ctrl Pts',(-0.117882265625521,-0.0741355877484928,
-0.680619268541745));
#49129=CARTESIAN_POINT('Ctrl Pts',(-0.00149207632259066,-0.13924829488388,
-0.672671977233793));
#49130=CARTESIAN_POINT('Ctrl Pts',(0.116266623106448,-0.0766445449542468,
-0.664724685925842));
#49131=CARTESIAN_POINT('Ctrl Pts',(0.12738731170417,0.0562564372903673,
-0.65677739461789));
#49132=CARTESIAN_POINT('Ctrl Pts',(0.0216702599226566,0.13755985517114,
-0.648830103309939));
#49133=CARTESIAN_POINT('Ctrl Pts',(-0.103922430718979,0.0926954276827039,
-0.640882812001986));
#49134=CARTESIAN_POINT('Ctrl Pts',(-0.134199019486038,-0.0371878621166431,
-0.632935520694035));
#49135=CARTESIAN_POINT('Ctrl Pts',(-0.0413902711963712,-0.13296300000418,
-0.624988229386083));
#49136=CARTESIAN_POINT('Ctrl Pts',(0.0893810158703018,-0.106786459449753,
-0.617040938078132));
#49137=CARTESIAN_POINT('Ctrl Pts',(0.138173369655621,0.0173330273706489,
-0.60909364677018));
#49138=CARTESIAN_POINT('Ctrl Pts',(0.0602351717464476,0.125554920271953,
-0.60114635546223));
#49139=CARTESIAN_POINT('Ctrl Pts',(-0.072949826366452,0.118619714857712,
-0.593199064154276));
#49140=CARTESIAN_POINT('Ctrl Pts',(-0.139226332890273,0.00288827798998521,
-0.585251772846326));
#49141=CARTESIAN_POINT('Ctrl Pts',(-0.0778065255617132,-0.115492244327638,
-0.577304481538374));
#49142=CARTESIAN_POINT('Ctrl Pts',(0.0549762653464128,-0.127945004468253,
-0.569357190230422));
#49143=CARTESIAN_POINT('Ctrl Pts',(0.137335646484491,-0.02304851675287,
-0.561409898922471));
#49144=CARTESIAN_POINT('Ctrl Pts',(0.0937328231132788,0.102987726409681,
-0.553462607614519));
#49145=CARTESIAN_POINT('Ctrl Pts',(-0.0358403461692648,0.134565164534837,
-0.545515316306567));
#49146=CARTESIAN_POINT('Ctrl Pts',(-0.132541285048275,0.0427214428311217,
-0.537568024998616));
#49147=CARTESIAN_POINT('Ctrl Pts',(-0.107677336146595,-0.0883057483983573,
-0.529620733690664));
#49148=CARTESIAN_POINT('Ctrl Pts',(0.0159466578264506,-0.13834022561781,
-0.521673442382713));
#49149=CARTESIAN_POINT('Ctrl Pts',(0.124944615327587,-0.0614911133454406,
-0.513726151074761));
#49150=CARTESIAN_POINT('Ctrl Pts',(0.119345237096187,0.071756730013814,
-0.50577885976681));
#49151=CARTESIAN_POINT('Ctrl Pts',(0.00428418924635087,0.139190371945483,
-0.497831568458857));
#49152=CARTESIAN_POINT('Ctrl Pts',(-0.11470625301651,0.0789606828664291,
-0.489884277150907));
#49153=CARTESIAN_POINT('Ctrl Pts',(-0.128489832597935,-0.053690565640297,
-0.481936985842954));
#49154=CARTESIAN_POINT('Ctrl Pts',(-0.0244244560972015,-0.137097628951694,
-0.473989694535004));
#49155=CARTESIAN_POINT('Ctrl Pts',(0.102042666874295,-0.0947607938812361,
-0.466042403227051));
#49156=CARTESIAN_POINT('Ctrl Pts',(0.134917779304342,0.0344892265411343,
-0.4580951119191));
#49157=CARTESIAN_POINT('Ctrl Pts',(0.0440483189035268,0.132106243310428,
-0.450147820611148));
#49158=CARTESIAN_POINT('Ctrl Pts',(-0.0872216019461573,0.108557386085731,
-0.442200529303197));
#49159=CARTESIAN_POINT('Ctrl Pts',(-0.13849317172527,-0.0145586848751967,
-0.434253237995245));
#49160=CARTESIAN_POINT('Ctrl Pts',(-0.0627408721263131,-0.124321747432419,
-0.426305946687293));
#49161=CARTESIAN_POINT('Ctrl Pts',(0.0705564186542189,-0.120058759391021,
-0.418358655379342));
#49162=CARTESIAN_POINT('Ctrl Pts',(0.139140415665318,-0.0056796697353837,
-0.41041136407139));
#49163=CARTESIAN_POINT('Ctrl Pts',(0.0801069008200053,0.113908728203041,
-0.402464072763439));
#49164=CARTESIAN_POINT('Ctrl Pts',(-0.0523994674467565,0.129021741311752,
-0.394516781455487));
#49165=CARTESIAN_POINT('Ctrl Pts',(-0.136845826504972,0.0257979396074864,
-0.386569490147535));
#49166=CARTESIAN_POINT('Ctrl Pts',(-0.0957792366260094,-0.101087347136819,
-0.378622198839584));
#49167=CARTESIAN_POINT('Ctrl Pts',(0.0331346390848385,-0.135256828339786,
-0.370674907531632));
#49168=CARTESIAN_POINT('Ctrl Pts',(0.131657918533283,-0.0453707659986463,
-0.362727616223681));
#49169=CARTESIAN_POINT('Ctrl Pts',(0.109426520779767,0.086128685522627,
-0.354780324915729));
#49170=CARTESIAN_POINT('Ctrl Pts',(-0.0131692480750101,0.138632192599552,
-0.346833033607777));
#49171=CARTESIAN_POINT('Ctrl Pts',(-0.123686379214668,0.0639843224281227,
-0.338885742299826));
#49172=CARTESIAN_POINT('Ctrl Pts',(-0.120760209998862,-0.0693490129767615,
-0.330938450991875));
#49173=CARTESIAN_POINT('Ctrl Pts',(-0.00707457914409293,-0.139076469072788,
-0.322991159683922));
#49174=CARTESIAN_POINT('Ctrl Pts',(0.113099750076884,-0.08124506417234,
-0.315043868375971));
#49175=CARTESIAN_POINT('Ctrl Pts',(0.12954067712726,0.0511031005833377,
-0.307096577068019));
#49176=CARTESIAN_POINT('Ctrl Pts',(0.0271688291824932,0.136580264462594,
-0.299149285760068));
#49177=CARTESIAN_POINT('Ctrl Pts',(-0.100121863252902,0.0967880489450682,
-0.291201994452116));
#49178=CARTESIAN_POINT('Ctrl Pts',(-0.135582277550388,-0.0317767200016701,
-0.283254703144164));
#49179=CARTESIAN_POINT('Ctrl Pts',(-0.0466886511469119,-0.131196355795028,
-0.275307411836213));
#49180=CARTESIAN_POINT('Ctrl Pts',(0.0850271090185907,-0.11028465283889,
-0.267360120528261));
#49181=CARTESIAN_POINT('Ctrl Pts',(0.138757274262191,0.0117784871313546,
-0.25941282922031));
#49182=CARTESIAN_POINT('Ctrl Pts',(0.0652213392245596,0.123038574559143,
-0.251465537912358));
#49183=CARTESIAN_POINT('Ctrl Pts',(-0.0681346343844765,0.121449518390703,
-0.243518246604407));
#49184=CARTESIAN_POINT('Ctrl Pts',(-0.138998538596432,0.00846877721585035,
-0.235570955296455));
#49185=CARTESIAN_POINT('Ctrl Pts',(-0.082375058485434,-0.112279399977289,
-0.227623663988504));
#49186=CARTESIAN_POINT('Ctrl Pts',(0.0498015954015689,-0.130046587870231,
-0.219676372680552));
#49187=CARTESIAN_POINT('Ctrl Pts',(0.136300969518302,-0.0285369869745706,
-0.2117290813726));
#49188=CARTESIAN_POINT('Ctrl Pts',(0.0977871294194325,0.099146312286434,
-0.203781790064648));
#49189=CARTESIAN_POINT('Ctrl Pts',(-0.0304156058568074,0.135894094238902,
-0.195834498756697));
#49190=CARTESIAN_POINT('Ctrl Pts',(-0.130721601450057,0.0480018417879172,
-0.187887207448745));
#49191=CARTESIAN_POINT('Ctrl Pts',(-0.111131696083687,-0.0839169831016152,
-0.179939916140794));
#49192=CARTESIAN_POINT('Ctrl Pts',(0.0103865420804345,-0.138868404314727,
-0.171992624832842));
#49193=CARTESIAN_POINT('Ctrl Pts',(0.12237839822605,-0.0664517977974861,
-0.164045333524891));
#49194=CARTESIAN_POINT('Ctrl Pts',(0.122126615970329,0.0669134043386132,
-0.156098042216939));
#49195=CARTESIAN_POINT('Ctrl Pts',(0.00986212241425144,0.138906633291134,
-0.148150750908988));
#49196=CARTESIAN_POINT('Ctrl Pts',(-0.111447757822021,0.0834967678264184,
-0.140203459601036));
#49197=CARTESIAN_POINT('Ctrl Pts',(-0.130539427544584,-0.0484950783731256,
-0.132256168293084));
#49198=CARTESIAN_POINT('Ctrl Pts',(-0.0299022661697765,-0.136007978091718,
-0.124308876985132));
#49199=CARTESIAN_POINT('Ctrl Pts',(0.0981607747731693,-0.0987763617687909,
-0.116361585677181));
#49200=CARTESIAN_POINT('Ctrl Pts',(0.136192280372371,0.0290514034709051,
-0.108414294369229));
#49201=CARTESIAN_POINT('Ctrl Pts',(0.0493101426383743,0.130233760247366,
-0.100467003061278));
#49202=CARTESIAN_POINT('Ctrl Pts',(-0.0827982993479119,0.111967457127882,
-0.0925197117533262));
#49203=CARTESIAN_POINT('Ctrl Pts',(-0.138965799441858,-0.00899334747060546,
-0.0845724204453746));
#49204=CARTESIAN_POINT('Ctrl Pts',(-0.0676751419254551,-0.12170630648443,
-0.0766251291374228));
#49205=CARTESIAN_POINT('Ctrl Pts',(0.0656846246959371,-0.122790694602604,
-0.0686778378294716));
#49206=CARTESIAN_POINT('Ctrl Pts',(0.138802320628112,-0.0112558793500066,
-0.0607305465215197));
#49207=CARTESIAN_POINT('Ctrl Pts',(0.0846071216902694,0.110607573555673,
-0.0527832552135683));
#49208=CARTESIAN_POINT('Ctrl Pts',(-0.0471780665789619,0.131014085359439,
-0.0448359639056163));
#49209=CARTESIAN_POINT('Ctrl Pts',(-0.135711977929724,0.0312741384470892,
-0.036888672597665));
#49210=CARTESIAN_POINT('Ctrl Pts',(-0.0997354011396044,-0.097183606994095,
-0.028941381289713));
#49211=CARTESIAN_POINT('Ctrl Pts',(0.027645696947688,-0.136441996699627,
-0.0209940899817616));
#49212=CARTESIAN_POINT('Ctrl Pts',(0.129807118062467,-0.0506808063214575,
-0.0130467986738099));
#49213=CARTESIAN_POINT('Ctrl Pts',(0.112641984414841,0.0818100865641861,
-0.00509950736585856));
#49214=CARTESIAN_POINT('Ctrl Pts',(0.0327209678848226,0.11973912564481,
0.000198686839442543));
#49215=CARTESIAN_POINT('Ctrl Pts',(-0.00642735618902915,0.117599488593358,
0.00284778394209306));
#49216=CARTESIAN_POINT('Ctrl Pts',(-0.00798678478681931,0.146131905375825,
-0.0136500000000002));
#49217=CARTESIAN_POINT('Ctrl Pts',(0.0406598484393165,0.148790668971504,
-0.0162990971026507));
#49218=CARTESIAN_POINT('Ctrl Pts',(0.0903157209469338,0.125224908540822,
-0.0189481942053012));
#49219=CARTESIAN_POINT('Ctrl Pts',(0.118698624029206,0.0860026422449412,
-0.0215972913079517));
#49220=CARTESIAN_POINT('Ctrl Pts',(0.147081527111478,0.0467803759490603,
-0.0242463884106022));
#49221=CARTESIAN_POINT('Ctrl Pts',(0.154191460768405,-0.00809839621201944,
-0.0268954855132527));
#49222=CARTESIAN_POINT('Ctrl Pts',(0.136588394652489,-0.0532992628159412,
-0.0295445826159032));
#49223=CARTESIAN_POINT('Ctrl Pts',(0.118985328536573,-0.0985001294198629,
-0.0321936797185537));
#49224=CARTESIAN_POINT('Ctrl Pts',(0.0766692626478151,-0.134023090466627,
-0.0348427768212043));
#49225=CARTESIAN_POINT('Ctrl Pts',(0.0291301022640015,-0.143654003759554,
-0.0374918739238548));
#49226=CARTESIAN_POINT('Ctrl Pts',(-0.0184090581198122,-0.153284917052481,
-0.0401409710265053));
#49227=CARTESIAN_POINT('Ctrl Pts',(-0.071171312998681,-0.137023782591571,
-0.0427900681291558));
#49228=CARTESIAN_POINT('Ctrl Pts',(-0.105003331279745,-0.102289110011485,
-0.0454391652318063));
#49229=CARTESIAN_POINT('Ctrl Pts',(-0.13116431054537,-0.075430143407223,
-0.0474876086264428));
#49230=CARTESIAN_POINT('Ctrl Pts',(-0.146006285598076,-0.0375252474656216,
-0.0495360520210795));
#49231=CARTESIAN_POINT('Ctrl Pts',(-0.146359156828661,0.000134286233873571,
-0.051584495415716));
#49232=CARTESIAN_POINT('Origin',(0.277715786349443,-0.0489687861020744,
0.04));
#49233=CARTESIAN_POINT('',(0.271097754137541,-0.0461628389679574,0.04));
#49234=CARTESIAN_POINT('',(0.27053717987482,-0.0493420135926708,0.04));
#49235=CARTESIAN_POINT('Origin',(0.,0.,0.04));
#49236=CARTESIAN_POINT('',(0.264913285560284,-0.0467113597924043,0.04));
#49237=CARTESIAN_POINT('',(0.29173382438227,-0.044332558140659,0.04));
#49238=CARTESIAN_POINT('',(0.264913285560284,-0.0467113597924043,0.04));
#49239=CARTESIAN_POINT('Origin',(0.264913285560284,-0.0467113597924043,
0.04));
#49240=CARTESIAN_POINT('',(0.27053717987482,-0.0493420135926708,0.285));
#49241=CARTESIAN_POINT('',(0.27053717987482,-0.0493420135926708,0.1425));
#49242=CARTESIAN_POINT('',(0.264913285560284,-0.0467113597924043,0.291));
#49243=CARTESIAN_POINT('',(0.264913285560284,-0.0467113597924043,0.04));
#49244=CARTESIAN_POINT('Ctrl Pts',(0.27053717987482,-0.0493420135926707,
0.285));
#49245=CARTESIAN_POINT('Ctrl Pts',(0.267694218594527,-0.048012179410566,
0.288035430631103));
#49246=CARTESIAN_POINT('Ctrl Pts',(0.264913285560284,-0.0467113597924043,
0.291));
#49247=CARTESIAN_POINT('Origin',(0.29173382438227,-0.044332558140659,0.04));
#49248=CARTESIAN_POINT('',(0.271097754137541,-0.0461628389679574,0.285));
#49249=CARTESIAN_POINT('',(0.271097754137541,-0.0461628389679574,0.1425));
#49250=CARTESIAN_POINT('Ctrl Pts',(0.264913285560284,-0.0467113597924043,
0.291));
#49251=CARTESIAN_POINT('Ctrl Pts',(0.267971414323715,-0.0464401243111941,
0.288035430631094));
#49252=CARTESIAN_POINT('Ctrl Pts',(0.271097754137541,-0.0461628389679575,
0.285));
#49253=CARTESIAN_POINT('Origin',(0.264993319061626,-0.0964496804178388,
0.04));
#49254=CARTESIAN_POINT('',(0.25896307723613,-0.0925371526922802,0.04));
#49255=CARTESIAN_POINT('',(0.257858961475997,-0.0955706858117092,0.04));
#49256=CARTESIAN_POINT('Origin',(0.,0.,0.04));
#49257=CARTESIAN_POINT('',(0.252777314991409,-0.0920034185546051,0.04));
#49258=CARTESIAN_POINT('',(0.279603464135123,-0.0943180939355711,0.04));
#49259=CARTESIAN_POINT('',(0.252777314991409,-0.0920034185546051,0.04));
#49260=CARTESIAN_POINT('Origin',(0.252777314991409,-0.0920034185546051,
0.04));
#49261=CARTESIAN_POINT('',(0.257858961475997,-0.0955706858117092,0.285));
#49262=CARTESIAN_POINT('',(0.257858961475997,-0.0955706858117092,0.1425));
#49263=CARTESIAN_POINT('',(0.252777314991409,-0.0920034185546051,0.291));
#49264=CARTESIAN_POINT('',(0.252777314991409,-0.0920034185546051,0.04));
#49265=CARTESIAN_POINT('Ctrl Pts',(0.257858961475997,-0.0955706858117092,
0.285));
#49266=CARTESIAN_POINT('Ctrl Pts',(0.255290114447966,-0.0937673797534469,
0.28803543063111));
#49267=CARTESIAN_POINT('Ctrl Pts',(0.252777314991409,-0.0920034185546051,
0.291));
#49268=CARTESIAN_POINT('Origin',(0.279603464135123,-0.0943180939355711,
0.04));
#49269=CARTESIAN_POINT('',(0.25896307723613,-0.0925371526922802,0.285));
#49270=CARTESIAN_POINT('',(0.25896307723613,-0.0925371526922802,0.1425));
#49271=CARTESIAN_POINT('Ctrl Pts',(0.252777314991409,-0.0920034185546051,
0.291));
#49272=CARTESIAN_POINT('Ctrl Pts',(0.255836083454352,-0.0922673422366557,
0.288035430631118));
#49273=CARTESIAN_POINT('Ctrl Pts',(0.25896307723613,-0.0925371526922802,
0.285));
#49274=CARTESIAN_POINT('Origin',(0.244219163867212,-0.141,0.04));
#49275=CARTESIAN_POINT('',(0.238959938274539,-0.136099771858106,0.04));
#49276=CARTESIAN_POINT('',(0.237345829015656,-0.138895491103459,0.04));
#49277=CARTESIAN_POINT('Origin',(0.,0.,0.04));
#49278=CARTESIAN_POINT('',(0.232960833618014,-0.1345,0.04));
#49279=CARTESIAN_POINT('',(0.258977494116409,-0.141437822173509,0.04));
#49280=CARTESIAN_POINT('',(0.232960833618014,-0.1345,0.04));
#49281=CARTESIAN_POINT('Origin',(0.232960833618014,-0.1345,0.04));
#49282=CARTESIAN_POINT('',(0.237345829015656,-0.138895491103459,0.285));
#49283=CARTESIAN_POINT('',(0.237345829015656,-0.138895491103459,0.1425));
#49284=CARTESIAN_POINT('',(0.232960833618014,-0.1345,0.291));
#49285=CARTESIAN_POINT('',(0.232960833618014,-0.1345,0.04));
#49286=CARTESIAN_POINT('Ctrl Pts',(0.237345829015656,-0.138895491103459,
0.285));
#49287=CARTESIAN_POINT('Ctrl Pts',(0.235129149356958,-0.136673505711122,
0.288035430631088));
#49288=CARTESIAN_POINT('Ctrl Pts',(0.232960833618014,-0.1345,0.291));
#49289=CARTESIAN_POINT('Origin',(0.258977494116409,-0.141437822173509,0.04));
#49290=CARTESIAN_POINT('',(0.238959938274539,-0.136099771858106,0.285));
#49291=CARTESIAN_POINT('',(0.238959938274539,-0.136099771858106,0.1425));
#49292=CARTESIAN_POINT('Ctrl Pts',(0.232960833618014,-0.1345,0.291));
#49293=CARTESIAN_POINT('Ctrl Pts',(0.235927302648582,-0.135291063657789,
0.288035430631094));
#49294=CARTESIAN_POINT('Ctrl Pts',(0.238959938274539,-0.136099771858106,
0.285));
#49295=CARTESIAN_POINT('Origin',(0.216024532959552,-0.181266105931604,0.04));
#49296=CARTESIAN_POINT('',(0.211696122508039,-0.175527068325832,0.04));
#49297=CARTESIAN_POINT('',(0.209621063643459,-0.17800002718254,0.04));
#49298=CARTESIAN_POINT('Origin',(0.,0.,0.04));
#49299=CARTESIAN_POINT('',(0.206065955199005,-0.172909867005679,0.04));
#49300=CARTESIAN_POINT('',(0.230482623987904,-0.184260033755696,0.04));
#49301=CARTESIAN_POINT('',(0.206065955199005,-0.172909867005679,0.04));
#49302=CARTESIAN_POINT('Origin',(0.206065955199005,-0.172909867005679,0.04));
#49303=CARTESIAN_POINT('',(0.209621063643459,-0.17800002718254,0.285));
#49304=CARTESIAN_POINT('',(0.209621063643459,-0.17800002718254,0.1425));
#49305=CARTESIAN_POINT('',(0.206065955199005,-0.172909867005679,0.291));
#49306=CARTESIAN_POINT('',(0.206065955199005,-0.172909867005679,0.04));
#49307=CARTESIAN_POINT('Ctrl Pts',(0.209621063643459,-0.17800002718254,
0.285));
#49308=CARTESIAN_POINT('Ctrl Pts',(0.207823904043776,-0.175426876357833,
0.288035430631146));
#49309=CARTESIAN_POINT('Ctrl Pts',(0.206065955199005,-0.172909867005679,
0.291));
#49310=CARTESIAN_POINT('Origin',(0.230482623987904,-0.184260033755696,0.04));
#49311=CARTESIAN_POINT('',(0.211696122508039,-0.175527068325832,0.285));
#49312=CARTESIAN_POINT('',(0.211696122508039,-0.175527068325832,0.1425));
#49313=CARTESIAN_POINT('Ctrl Pts',(0.206065955199005,-0.172909867005679,
0.291));
#49314=CARTESIAN_POINT('Ctrl Pts',(0.208849990136834,-0.174204034570282,
0.288035430631042));
#49315=CARTESIAN_POINT('Ctrl Pts',(0.211696122508039,-0.175527068325832,
0.285));
#49316=CARTESIAN_POINT('Origin',(0.181266105931604,-0.216024532959552,0.04));
#49317=CARTESIAN_POINT('',(0.17800002718254,-0.209621063643459,0.04));
#49318=CARTESIAN_POINT('',(0.175527068325832,-0.211696122508039,0.04));
#49319=CARTESIAN_POINT('Origin',(0.,0.,0.04));
#49320=CARTESIAN_POINT('',(0.172909867005679,-0.206065955199005,0.04));
#49321=CARTESIAN_POINT('',(0.194984655959362,-0.221483597452293,0.04));
#49322=CARTESIAN_POINT('',(0.172909867005679,-0.206065955199005,0.04));
#49323=CARTESIAN_POINT('Origin',(0.172909867005679,-0.206065955199005,0.04));
#49324=CARTESIAN_POINT('',(0.175527068325832,-0.211696122508039,0.285));
#49325=CARTESIAN_POINT('',(0.175527068325832,-0.211696122508039,0.1425));
#49326=CARTESIAN_POINT('',(0.172909867005679,-0.206065955199005,0.291));
#49327=CARTESIAN_POINT('',(0.172909867005679,-0.206065955199005,0.04));
#49328=CARTESIAN_POINT('Ctrl Pts',(0.175527068325832,-0.211696122508039,
0.285));
#49329=CARTESIAN_POINT('Ctrl Pts',(0.174204034570244,-0.208849990136752,
0.288035430631129));
#49330=CARTESIAN_POINT('Ctrl Pts',(0.172909867005679,-0.206065955199005,
0.291));
#49331=CARTESIAN_POINT('Origin',(0.194984655959362,-0.221483597452293,0.04));
#49332=CARTESIAN_POINT('',(0.17800002718254,-0.209621063643459,0.285));
#49333=CARTESIAN_POINT('',(0.17800002718254,-0.209621063643459,0.1425));
#49334=CARTESIAN_POINT('Ctrl Pts',(0.172909867005679,-0.206065955199005,
0.291));
#49335=CARTESIAN_POINT('Ctrl Pts',(0.175426876357872,-0.207823904043804,
0.2880354306311));
#49336=CARTESIAN_POINT('Ctrl Pts',(0.17800002718254,-0.209621063643459,
0.285));
#49337=CARTESIAN_POINT('Origin',(0.141,-0.244219163867212,0.04));
#49338=CARTESIAN_POINT('',(0.138895491103459,-0.237345829015656,0.04));
#49339=CARTESIAN_POINT('',(0.136099771858106,-0.238959938274539,0.04));
#49340=CARTESIAN_POINT('Origin',(0.,0.,0.04));
#49341=CARTESIAN_POINT('',(0.1345,-0.232960833618014,0.04));
#49342=CARTESIAN_POINT('',(0.153562177826491,-0.251977494116409,0.04));
#49343=CARTESIAN_POINT('',(0.1345,-0.232960833618014,0.04));
#49344=CARTESIAN_POINT('Origin',(0.1345,-0.232960833618014,0.04));
#49345=CARTESIAN_POINT('',(0.136099771858106,-0.238959938274539,0.285));
#49346=CARTESIAN_POINT('',(0.136099771858106,-0.238959938274539,0.1425));
#49347=CARTESIAN_POINT('',(0.1345,-0.232960833618014,0.291));
#49348=CARTESIAN_POINT('',(0.1345,-0.232960833618014,0.04));
#49349=CARTESIAN_POINT('Ctrl Pts',(0.136099771858106,-0.238959938274539,
0.285));
#49350=CARTESIAN_POINT('Ctrl Pts',(0.135291063657772,-0.23592730264852,
0.288035430631155));
#49351=CARTESIAN_POINT('Ctrl Pts',(0.1345,-0.232960833618014,0.291));
#49352=CARTESIAN_POINT('Origin',(0.153562177826491,-0.251977494116409,0.04));
#49353=CARTESIAN_POINT('',(0.138895491103459,-0.237345829015656,0.285));
#49354=CARTESIAN_POINT('',(0.138895491103459,-0.237345829015656,0.1425));
#49355=CARTESIAN_POINT('Ctrl Pts',(0.1345,-0.232960833618014,0.291));
#49356=CARTESIAN_POINT('Ctrl Pts',(0.136673505711114,-0.23512914935695,
0.288035430631099));
#49357=CARTESIAN_POINT('Ctrl Pts',(0.138895491103459,-0.237345829015656,
0.285));
#49358=CARTESIAN_POINT('Origin',(0.0964496804178385,-0.264993319061626,
0.04));
#49359=CARTESIAN_POINT('',(0.0955706858117088,-0.257858961475997,0.04));
#49360=CARTESIAN_POINT('',(0.0925371526922799,-0.25896307723613,0.04));
#49361=CARTESIAN_POINT('Origin',(0.,0.,0.04));
#49362=CARTESIAN_POINT('',(0.0920034185546048,-0.252777314991409,0.04));
#49363=CARTESIAN_POINT('',(0.107473790626574,-0.274815182128563,0.04));
#49364=CARTESIAN_POINT('',(0.0920034185546048,-0.252777314991409,0.04));
#49365=CARTESIAN_POINT('Origin',(0.0920034185546048,-0.252777314991409,
0.04));
#49366=CARTESIAN_POINT('',(0.0925371526922799,-0.25896307723613,0.285));
#49367=CARTESIAN_POINT('',(0.0925371526922799,-0.25896307723613,0.1425));
#49368=CARTESIAN_POINT('',(0.0920034185546048,-0.252777314991409,0.291));
#49369=CARTESIAN_POINT('',(0.0920034185546048,-0.252777314991409,0.04));
#49370=CARTESIAN_POINT('Ctrl Pts',(0.0925371526922799,-0.25896307723613,
0.285));
#49371=CARTESIAN_POINT('Ctrl Pts',(0.0922673422366487,-0.255836083454274,
0.288035430631194));
#49372=CARTESIAN_POINT('Ctrl Pts',(0.0920034185546048,-0.252777314991409,
0.291));
#49373=CARTESIAN_POINT('Origin',(0.107473790626574,-0.274815182128563,0.04));
#49374=CARTESIAN_POINT('',(0.0955706858117089,-0.257858961475997,0.285));
#49375=CARTESIAN_POINT('',(0.0955706858117089,-0.257858961475997,0.1425));
#49376=CARTESIAN_POINT('Ctrl Pts',(0.0920034185546048,-0.252777314991409,
0.291));
#49377=CARTESIAN_POINT('Ctrl Pts',(0.0937673797534969,-0.255290114448038,
0.288035430631026));
#49378=CARTESIAN_POINT('Ctrl Pts',(0.0955706858117088,-0.257858961475997,
0.285));
#49379=CARTESIAN_POINT('Origin',(0.0489687861020743,-0.277715786349443,
0.04));
#49380=CARTESIAN_POINT('',(0.0493420135926707,-0.27053717987482,0.04));
#49381=CARTESIAN_POINT('',(0.0461628389679573,-0.271097754137541,0.04));
#49382=CARTESIAN_POINT('Origin',(0.,0.,0.04));
#49383=CARTESIAN_POINT('',(0.0467113597924042,-0.264913285560284,0.04));
#49384=CARTESIAN_POINT('',(0.0581198666828298,-0.289302749894933,0.04));
#49385=CARTESIAN_POINT('',(0.0467113597924042,-0.264913285560284,0.04));
#49386=CARTESIAN_POINT('Origin',(0.0467113597924042,-0.264913285560284,
0.04));
#49387=CARTESIAN_POINT('',(0.0461628389679573,-0.271097754137541,0.285));
#49388=CARTESIAN_POINT('',(0.0461628389679573,-0.271097754137541,0.1425));
#49389=CARTESIAN_POINT('',(0.0467113597924042,-0.264913285560284,0.291));
#49390=CARTESIAN_POINT('',(0.0467113597924042,-0.264913285560284,0.04));
#49391=CARTESIAN_POINT('Ctrl Pts',(0.0461628389679573,-0.271097754137541,
0.285));
#49392=CARTESIAN_POINT('Ctrl Pts',(0.0464401243112015,-0.26797141432363,
0.288035430631177));
#49393=CARTESIAN_POINT('Ctrl Pts',(0.0467113597924042,-0.264913285560284,
0.291));
#49394=CARTESIAN_POINT('Origin',(0.0581198666828298,-0.289302749894933,
0.04));
#49395=CARTESIAN_POINT('',(0.0493420135926707,-0.27053717987482,0.285));
#49396=CARTESIAN_POINT('',(0.0493420135926707,-0.27053717987482,0.1425));
#49397=CARTESIAN_POINT('Ctrl Pts',(0.0467113597924042,-0.264913285560284,
0.291));
#49398=CARTESIAN_POINT('Ctrl Pts',(0.0480121794105309,-0.267694218594452,
0.288035430631183));
#49399=CARTESIAN_POINT('Ctrl Pts',(0.0493420135926707,-0.27053717987482,
0.285));
#49400=CARTESIAN_POINT('Origin',(-4.85722573273506E-17,-0.282,0.04));
#49401=CARTESIAN_POINT('',(0.00161410925888288,-0.274995262961565,0.04));
#49402=CARTESIAN_POINT('',(-0.00161410925888299,-0.274995262961565,0.04));
#49403=CARTESIAN_POINT('Origin',(0.,0.,0.04));
#49404=CARTESIAN_POINT('',(-6.24500451351651E-17,-0.269,0.04));
#49405=CARTESIAN_POINT('',(0.00699999999999995,-0.295,0.04));
#49406=CARTESIAN_POINT('',(-6.24500451351651E-17,-0.269,0.04));
#49407=CARTESIAN_POINT('Origin',(-6.24500451351651E-17,-0.269,0.04));
#49408=CARTESIAN_POINT('',(-0.00161410925888297,-0.274995262961565,0.285));
#49409=CARTESIAN_POINT('',(-0.00161410925888297,-0.274995262961565,0.1425));
#49410=CARTESIAN_POINT('',(-6.2450045135165E-17,-0.269,0.291));
#49411=CARTESIAN_POINT('',(-6.24500451351651E-17,-0.269,0.04));
#49412=CARTESIAN_POINT('Ctrl Pts',(-0.00161410925888296,-0.274995262961565,
0.285));
#49413=CARTESIAN_POINT('Ctrl Pts',(-0.000798153291622722,-0.271964569368884,
0.288035430631116));
#49414=CARTESIAN_POINT('Ctrl Pts',(-6.24500451351651E-17,-0.269,0.291));
#49415=CARTESIAN_POINT('Origin',(0.00699999999999995,-0.295,0.04));
#49416=CARTESIAN_POINT('',(0.00161410925888286,-0.274995262961565,0.285));
#49417=CARTESIAN_POINT('',(0.00161410925888286,-0.274995262961565,0.1425));
#49418=CARTESIAN_POINT('Ctrl Pts',(-6.2450045135165E-17,-0.269,0.291));
#49419=CARTESIAN_POINT('Ctrl Pts',(0.000798153291617013,-0.271964569368863,
0.288035430631137));
#49420=CARTESIAN_POINT('Ctrl Pts',(0.00161410925888284,-0.274995262961565,
0.285));
#49421=CARTESIAN_POINT('Origin',(-0.0489687861020744,-0.277715786349443,
0.04));
#49422=CARTESIAN_POINT('',(-0.0461628389679574,-0.271097754137541,0.04));
#49423=CARTESIAN_POINT('',(-0.0493420135926708,-0.27053717987482,0.04));
#49424=CARTESIAN_POINT('Origin',(0.,0.,0.04));
#49425=CARTESIAN_POINT('',(-0.0467113597924043,-0.264913285560284,0.04));
#49426=CARTESIAN_POINT('',(-0.044332558140659,-0.29173382438227,0.04));
#49427=CARTESIAN_POINT('',(-0.0467113597924043,-0.264913285560284,0.04));
#49428=CARTESIAN_POINT('Origin',(-0.0467113597924043,-0.264913285560284,
0.04));
#49429=CARTESIAN_POINT('',(-0.0493420135926708,-0.27053717987482,0.285));
#49430=CARTESIAN_POINT('',(-0.0493420135926708,-0.27053717987482,0.1425));
#49431=CARTESIAN_POINT('',(-0.0467113597924043,-0.264913285560284,0.291));
#49432=CARTESIAN_POINT('',(-0.0467113597924043,-0.264913285560284,0.04));
#49433=CARTESIAN_POINT('Ctrl Pts',(-0.0493420135926708,-0.27053717987482,
0.285));
#49434=CARTESIAN_POINT('Ctrl Pts',(-0.0480121794105265,-0.267694218594442,
0.288035430631193));
#49435=CARTESIAN_POINT('Ctrl Pts',(-0.0467113597924043,-0.264913285560284,
0.291));
#49436=CARTESIAN_POINT('Origin',(-0.044332558140659,-0.29173382438227,0.04));
#49437=CARTESIAN_POINT('',(-0.0461628389679574,-0.271097754137541,0.285));
#49438=CARTESIAN_POINT('',(-0.0461628389679574,-0.271097754137541,0.1425));
#49439=CARTESIAN_POINT('Ctrl Pts',(-0.0467113597924043,-0.264913285560284,
0.291));
#49440=CARTESIAN_POINT('Ctrl Pts',(-0.046440124311189,-0.267971414323772,
0.288035430631039));
#49441=CARTESIAN_POINT('Ctrl Pts',(-0.0461628389679575,-0.271097754137541,
0.285));
#49442=CARTESIAN_POINT('Origin',(-0.0964496804178388,-0.264993319061626,
0.04));
#49443=CARTESIAN_POINT('',(-0.0925371526922802,-0.25896307723613,0.04));
#49444=CARTESIAN_POINT('',(-0.0955706858117092,-0.257858961475997,0.04));
#49445=CARTESIAN_POINT('Origin',(0.,0.,0.04));
#49446=CARTESIAN_POINT('',(-0.0920034185546051,-0.252777314991409,0.04));
#49447=CARTESIAN_POINT('',(-0.0943180939355711,-0.279603464135123,0.04));
#49448=CARTESIAN_POINT('',(-0.0920034185546051,-0.252777314991409,0.04));
#49449=CARTESIAN_POINT('Origin',(-0.0920034185546051,-0.252777314991409,
0.04));
#49450=CARTESIAN_POINT('',(-0.0955706858117092,-0.257858961475997,0.285));
#49451=CARTESIAN_POINT('',(-0.0955706858117092,-0.257858961475997,0.1425));
#49452=CARTESIAN_POINT('',(-0.0920034185546051,-0.252777314991409,0.291));
#49453=CARTESIAN_POINT('',(-0.0920034185546051,-0.252777314991409,0.04));
#49454=CARTESIAN_POINT('Ctrl Pts',(-0.0955706858117091,-0.257858961475997,
0.285));
#49455=CARTESIAN_POINT('Ctrl Pts',(-0.0937673797534664,-0.255290114447994,
0.288035430631078));
#49456=CARTESIAN_POINT('Ctrl Pts',(-0.0920034185546051,-0.252777314991409,
0.291));
#49457=CARTESIAN_POINT('Origin',(-0.0943180939355711,-0.279603464135123,
0.04));
#49458=CARTESIAN_POINT('',(-0.0925371526922802,-0.25896307723613,0.285));
#49459=CARTESIAN_POINT('',(-0.0925371526922802,-0.25896307723613,0.1425));
#49460=CARTESIAN_POINT('Ctrl Pts',(-0.0920034185546051,-0.252777314991409,
0.291));
#49461=CARTESIAN_POINT('Ctrl Pts',(-0.0922673422366578,-0.255836083454375,
0.288035430631095));
#49462=CARTESIAN_POINT('Ctrl Pts',(-0.0925371526922802,-0.25896307723613,
0.285));
#49463=CARTESIAN_POINT('Origin',(-0.141,-0.244219163867212,0.04));
#49464=CARTESIAN_POINT('',(-0.136099771858106,-0.238959938274539,0.04));
#49465=CARTESIAN_POINT('',(-0.138895491103459,-0.237345829015656,0.04));
#49466=CARTESIAN_POINT('Origin',(0.,0.,0.04));
#49467=CARTESIAN_POINT('',(-0.1345,-0.232960833618014,0.04));
#49468=CARTESIAN_POINT('',(-0.141437822173509,-0.258977494116409,0.04));
#49469=CARTESIAN_POINT('',(-0.1345,-0.232960833618014,0.04));
#49470=CARTESIAN_POINT('Origin',(-0.1345,-0.232960833618014,0.04));
#49471=CARTESIAN_POINT('',(-0.138895491103459,-0.237345829015656,0.285));
#49472=CARTESIAN_POINT('',(-0.138895491103459,-0.237345829015656,0.1425));
#49473=CARTESIAN_POINT('',(-0.1345,-0.232960833618014,0.291));
#49474=CARTESIAN_POINT('',(-0.1345,-0.232960833618014,0.04));
#49475=CARTESIAN_POINT('Ctrl Pts',(-0.138895491103459,-0.237345829015656,
0.285));
#49476=CARTESIAN_POINT('Ctrl Pts',(-0.136673505711122,-0.235129149356958,
0.288035430631088));
#49477=CARTESIAN_POINT('Ctrl Pts',(-0.1345,-0.232960833618014,0.291));
#49478=CARTESIAN_POINT('Origin',(-0.141437822173509,-0.258977494116409,
0.04));
#49479=CARTESIAN_POINT('',(-0.136099771858106,-0.238959938274539,0.285));
#49480=CARTESIAN_POINT('',(-0.136099771858106,-0.238959938274539,0.1425));
#49481=CARTESIAN_POINT('Ctrl Pts',(-0.1345,-0.232960833618014,0.291));
#49482=CARTESIAN_POINT('Ctrl Pts',(-0.135291063657789,-0.235927302648582,
0.288035430631094));
#49483=CARTESIAN_POINT('Ctrl Pts',(-0.136099771858106,-0.238959938274539,
0.285));
#49484=CARTESIAN_POINT('Origin',(-0.181266105931604,-0.216024532959552,
0.04));
#49485=CARTESIAN_POINT('',(-0.175527068325832,-0.211696122508039,0.04));
#49486=CARTESIAN_POINT('',(-0.17800002718254,-0.209621063643459,0.04));
#49487=CARTESIAN_POINT('Origin',(0.,0.,0.04));
#49488=CARTESIAN_POINT('',(-0.172909867005679,-0.206065955199005,0.04));
#49489=CARTESIAN_POINT('',(-0.184260033755696,-0.230482623987904,0.04));
#49490=CARTESIAN_POINT('',(-0.172909867005679,-0.206065955199005,0.04));
#49491=CARTESIAN_POINT('Origin',(-0.172909867005679,-0.206065955199005,
0.04));
#49492=CARTESIAN_POINT('',(-0.17800002718254,-0.209621063643459,0.285));
#49493=CARTESIAN_POINT('',(-0.17800002718254,-0.209621063643459,0.1425));
#49494=CARTESIAN_POINT('',(-0.172909867005679,-0.206065955199005,0.291));
#49495=CARTESIAN_POINT('',(-0.172909867005679,-0.206065955199005,0.04));
#49496=CARTESIAN_POINT('Ctrl Pts',(-0.17800002718254,-0.209621063643459,
0.285));
#49497=CARTESIAN_POINT('Ctrl Pts',(-0.175426876357765,-0.207823904043728,
0.288035430631226));
#49498=CARTESIAN_POINT('Ctrl Pts',(-0.172909867005679,-0.206065955199005,
0.291));
#49499=CARTESIAN_POINT('Origin',(-0.184260033755696,-0.230482623987904,
0.04));
#49500=CARTESIAN_POINT('',(-0.175527068325832,-0.211696122508039,0.285));
#49501=CARTESIAN_POINT('',(-0.175527068325832,-0.211696122508039,0.1425));
#49502=CARTESIAN_POINT('Ctrl Pts',(-0.172909867005679,-0.206065955199005,
0.291));
#49503=CARTESIAN_POINT('Ctrl Pts',(-0.174204034570293,-0.208849990136858,
0.288035430631017));
#49504=CARTESIAN_POINT('Ctrl Pts',(-0.175527068325832,-0.211696122508039,
0.285));
#49505=CARTESIAN_POINT('Origin',(-0.216024532959552,-0.181266105931604,
0.04));
#49506=CARTESIAN_POINT('',(-0.209621063643459,-0.17800002718254,0.04));
#49507=CARTESIAN_POINT('',(-0.211696122508039,-0.175527068325832,0.04));
#49508=CARTESIAN_POINT('Origin',(0.,0.,0.04));
#49509=CARTESIAN_POINT('',(-0.206065955199005,-0.172909867005679,0.04));
#49510=CARTESIAN_POINT('',(-0.221483597452293,-0.194984655959362,0.04));
#49511=CARTESIAN_POINT('',(-0.206065955199005,-0.172909867005679,0.04));
#49512=CARTESIAN_POINT('Origin',(-0.206065955199005,-0.172909867005679,
0.04));
#49513=CARTESIAN_POINT('',(-0.211696122508039,-0.175527068325832,0.285));
#49514=CARTESIAN_POINT('',(-0.211696122508039,-0.175527068325832,0.1425));
#49515=CARTESIAN_POINT('',(-0.206065955199005,-0.172909867005679,0.291));
#49516=CARTESIAN_POINT('',(-0.206065955199005,-0.172909867005679,0.04));
#49517=CARTESIAN_POINT('Ctrl Pts',(-0.211696122508039,-0.175527068325832,
0.285));
#49518=CARTESIAN_POINT('Ctrl Pts',(-0.208849990136656,-0.174204034570199,
0.288035430631232));
#49519=CARTESIAN_POINT('Ctrl Pts',(-0.206065955199005,-0.172909867005679,
0.291));
#49520=CARTESIAN_POINT('Origin',(-0.221483597452293,-0.194984655959362,
0.04));
#49521=CARTESIAN_POINT('',(-0.209621063643459,-0.17800002718254,0.285));
#49522=CARTESIAN_POINT('',(-0.209621063643459,-0.17800002718254,0.1425));
#49523=CARTESIAN_POINT('Ctrl Pts',(-0.206065955199005,-0.172909867005679,
0.291));
#49524=CARTESIAN_POINT('Ctrl Pts',(-0.207823904043843,-0.175426876357928,
0.288035430631034));
#49525=CARTESIAN_POINT('Ctrl Pts',(-0.209621063643459,-0.17800002718254,
0.285));
#49526=CARTESIAN_POINT('Origin',(-0.244219163867212,-0.141,0.04));
#49527=CARTESIAN_POINT('',(-0.237345829015656,-0.138895491103459,0.04));
#49528=CARTESIAN_POINT('',(-0.238959938274539,-0.136099771858106,0.04));
#49529=CARTESIAN_POINT('Origin',(0.,0.,0.04));
#49530=CARTESIAN_POINT('',(-0.232960833618014,-0.1345,0.04));
#49531=CARTESIAN_POINT('',(-0.25197749411641,-0.153562177826491,0.04));
#49532=CARTESIAN_POINT('',(-0.232960833618014,-0.1345,0.04));
#49533=CARTESIAN_POINT('Origin',(-0.232960833618014,-0.1345,0.04));
#49534=CARTESIAN_POINT('',(-0.238959938274539,-0.136099771858106,0.285));
#49535=CARTESIAN_POINT('',(-0.238959938274539,-0.136099771858106,0.1425));
#49536=CARTESIAN_POINT('',(-0.232960833618014,-0.1345,0.291));
#49537=CARTESIAN_POINT('',(-0.232960833618014,-0.1345,0.04));
#49538=CARTESIAN_POINT('Ctrl Pts',(-0.238959938274539,-0.136099771858106,
0.285));
#49539=CARTESIAN_POINT('Ctrl Pts',(-0.23592730264851,-0.135291063657769,
0.288035430631166));
#49540=CARTESIAN_POINT('Ctrl Pts',(-0.232960833618014,-0.1345,0.291));
#49541=CARTESIAN_POINT('Origin',(-0.25197749411641,-0.153562177826491,0.04));
#49542=CARTESIAN_POINT('',(-0.237345829015656,-0.138895491103459,0.285));
#49543=CARTESIAN_POINT('',(-0.237345829015656,-0.138895491103459,0.1425));
#49544=CARTESIAN_POINT('Ctrl Pts',(-0.232960833618014,-0.1345,0.291));
#49545=CARTESIAN_POINT('Ctrl Pts',(-0.235129149356959,-0.136673505711123,
0.288035430631086));
#49546=CARTESIAN_POINT('Ctrl Pts',(-0.237345829015656,-0.138895491103459,
0.285));
#49547=CARTESIAN_POINT('Origin',(-0.264993319061626,-0.0964496804178386,
0.04));
#49548=CARTESIAN_POINT('',(-0.257858961475997,-0.095570685811709,0.04));
#49549=CARTESIAN_POINT('',(-0.25896307723613,-0.09253715269228,0.04));
#49550=CARTESIAN_POINT('Origin',(0.,0.,0.04));
#49551=CARTESIAN_POINT('',(-0.252777314991409,-0.0920034185546049,0.04));
#49552=CARTESIAN_POINT('',(-0.274815182128563,-0.107473790626574,0.04));
#49553=CARTESIAN_POINT('',(-0.252777314991409,-0.0920034185546049,0.04));
#49554=CARTESIAN_POINT('Origin',(-0.252777314991409,-0.0920034185546049,
0.04));
#49555=CARTESIAN_POINT('',(-0.25896307723613,-0.09253715269228,0.285));
#49556=CARTESIAN_POINT('',(-0.25896307723613,-0.09253715269228,0.1425));
#49557=CARTESIAN_POINT('',(-0.252777314991409,-0.0920034185546049,0.291));
#49558=CARTESIAN_POINT('',(-0.252777314991409,-0.0920034185546049,0.04));
#49559=CARTESIAN_POINT('Ctrl Pts',(-0.25896307723613,-0.09253715269228,
0.285));
#49560=CARTESIAN_POINT('Ctrl Pts',(-0.255836083454338,-0.0922673422366543,
0.288035430631132));
#49561=CARTESIAN_POINT('Ctrl Pts',(-0.252777314991409,-0.0920034185546049,
0.291));
#49562=CARTESIAN_POINT('Origin',(-0.274815182128563,-0.107473790626574,
0.04));
#49563=CARTESIAN_POINT('',(-0.257858961475997,-0.095570685811709,0.285));
#49564=CARTESIAN_POINT('',(-0.257858961475997,-0.095570685811709,0.1425));
#49565=CARTESIAN_POINT('Ctrl Pts',(-0.252777314991409,-0.0920034185546049,
0.291));
#49566=CARTESIAN_POINT('Ctrl Pts',(-0.255290114448016,-0.0937673797534821,
0.288035430631051));
#49567=CARTESIAN_POINT('Ctrl Pts',(-0.257858961475997,-0.0955706858117089,
0.285));
#49568=CARTESIAN_POINT('Origin',(-0.277715786349443,-0.0489687861020743,
0.04));
#49569=CARTESIAN_POINT('',(-0.27053717987482,-0.0493420135926707,0.04));
#49570=CARTESIAN_POINT('',(-0.271097754137541,-0.0461628389679573,0.04));
#49571=CARTESIAN_POINT('Origin',(0.,0.,0.04));
#49572=CARTESIAN_POINT('',(-0.264913285560284,-0.0467113597924042,0.04));
#49573=CARTESIAN_POINT('',(-0.289302749894933,-0.0581198666828298,0.04));
#49574=CARTESIAN_POINT('',(-0.264913285560284,-0.0467113597924042,0.04));
#49575=CARTESIAN_POINT('Origin',(-0.264913285560284,-0.0467113597924042,
0.04));
#49576=CARTESIAN_POINT('',(-0.271097754137541,-0.0461628389679573,0.285));
#49577=CARTESIAN_POINT('',(-0.271097754137541,-0.0461628389679573,0.1425));
#49578=CARTESIAN_POINT('',(-0.264913285560284,-0.0467113597924042,0.291));
#49579=CARTESIAN_POINT('',(-0.264913285560284,-0.0467113597924042,0.04));
#49580=CARTESIAN_POINT('Ctrl Pts',(-0.271097754137541,-0.0461628389679573,
0.285));
#49581=CARTESIAN_POINT('Ctrl Pts',(-0.267971414323669,-0.0464401243111981,
0.288035430631139));
#49582=CARTESIAN_POINT('Ctrl Pts',(-0.264913285560284,-0.0467113597924042,
0.291));
#49583=CARTESIAN_POINT('Origin',(-0.289302749894933,-0.0581198666828298,
0.04));
#49584=CARTESIAN_POINT('',(-0.27053717987482,-0.0493420135926707,0.285));
#49585=CARTESIAN_POINT('',(-0.27053717987482,-0.0493420135926707,0.1425));
#49586=CARTESIAN_POINT('Ctrl Pts',(-0.264913285560284,-0.0467113597924042,
0.291));
#49587=CARTESIAN_POINT('Ctrl Pts',(-0.2676942185945,-0.0480121794105537,
0.288035430631131));
#49588=CARTESIAN_POINT('Ctrl Pts',(-0.27053717987482,-0.0493420135926707,
0.285));
#49589=CARTESIAN_POINT('Origin',(-0.282,2.77555756156289E-17,0.04));
#49590=CARTESIAN_POINT('',(-0.274995262961565,-0.0016141092588829,0.04));
#49591=CARTESIAN_POINT('',(-0.275,-3.36777869765522E-17,0.04));
#49592=CARTESIAN_POINT('Origin',(0.,0.,0.04));
#49593=CARTESIAN_POINT('',(-0.269,4.16333634234434E-17,0.04));
#49594=CARTESIAN_POINT('',(-0.295,-0.00699999999999998,0.04));
#49595=CARTESIAN_POINT('',(-0.274995262961565,0.00161410925888296,0.04));
#49596=CARTESIAN_POINT('',(-0.269,4.16333634234434E-17,0.04));
#49597=CARTESIAN_POINT('Origin',(0.,0.,0.04));
#49598=CARTESIAN_POINT('Origin',(-0.269,4.16333634234434E-17,0.04));
#49599=CARTESIAN_POINT('',(-0.274995262961565,0.00161410925888297,0.285));
#49600=CARTESIAN_POINT('',(-0.274995262961565,0.00161410925888297,0.1425));
#49601=CARTESIAN_POINT('',(-0.269,4.16333634234434E-17,0.291));
#49602=CARTESIAN_POINT('',(-0.269,4.16333634234434E-17,0.04));
#49603=CARTESIAN_POINT('Ctrl Pts',(-0.274995262961565,0.00161410925888294,
0.285));
#49604=CARTESIAN_POINT('Ctrl Pts',(-0.271964569368884,0.000798153291622702,
0.288035430631116));
#49605=CARTESIAN_POINT('Ctrl Pts',(-0.269,4.16333634234434E-17,0.291));
#49606=CARTESIAN_POINT('Origin',(-0.295,-0.00699999999999998,0.04));
#49607=CARTESIAN_POINT('',(-0.274995262961565,-0.0016141092588829,0.285));
#49608=CARTESIAN_POINT('',(-0.274995262961565,-0.0016141092588829,0.1425));
#49609=CARTESIAN_POINT('Ctrl Pts',(-0.269,4.16333634234434E-17,0.291));
#49610=CARTESIAN_POINT('Ctrl Pts',(-0.271964569368901,-0.000798153291627193,
0.288035430631099));
#49611=CARTESIAN_POINT('Ctrl Pts',(-0.274995262961565,-0.00161410925888289,
0.285));
#49612=CARTESIAN_POINT('Origin',(-0.277715786349443,0.0489687861020745,
0.04));
#49613=CARTESIAN_POINT('',(-0.271097754137541,0.0461628389679575,0.04));
#49614=CARTESIAN_POINT('',(-0.27053717987482,0.0493420135926709,0.04));
#49615=CARTESIAN_POINT('Origin',(0.,0.,0.04));
#49616=CARTESIAN_POINT('',(-0.264913285560284,0.0467113597924044,0.04));
#49617=CARTESIAN_POINT('',(-0.29173382438227,0.0443325581406591,0.04));
#49618=CARTESIAN_POINT('',(-0.264913285560284,0.0467113597924044,0.04));
#49619=CARTESIAN_POINT('Origin',(-0.264913285560284,0.0467113597924044,
0.04));
#49620=CARTESIAN_POINT('',(-0.27053717987482,0.0493420135926709,0.285));
#49621=CARTESIAN_POINT('',(-0.27053717987482,0.0493420135926709,0.1425));
#49622=CARTESIAN_POINT('',(-0.264913285560284,0.0467113597924044,0.291));
#49623=CARTESIAN_POINT('',(-0.264913285560284,0.0467113597924044,0.04));
#49624=CARTESIAN_POINT('Ctrl Pts',(-0.27053717987482,0.0493420135926709,
0.285));
#49625=CARTESIAN_POINT('Ctrl Pts',(-0.267694218594536,0.0480121794105704,
0.288035430631093));
#49626=CARTESIAN_POINT('Ctrl Pts',(-0.264913285560284,0.0467113597924044,
0.291));
#49627=CARTESIAN_POINT('Origin',(-0.29173382438227,0.0443325581406591,0.04));
#49628=CARTESIAN_POINT('',(-0.271097754137541,0.0461628389679575,0.285));
#49629=CARTESIAN_POINT('',(-0.271097754137541,0.0461628389679575,0.1425));
#49630=CARTESIAN_POINT('Ctrl Pts',(-0.264913285560284,0.0467113597924044,
0.291));
#49631=CARTESIAN_POINT('Ctrl Pts',(-0.267971414323744,0.0464401243111915,
0.288035430631066));
#49632=CARTESIAN_POINT('Ctrl Pts',(-0.271097754137541,0.0461628389679575,
0.285));
#49633=CARTESIAN_POINT('Origin',(-0.264993319061626,0.0964496804178386,
0.04));
#49634=CARTESIAN_POINT('',(-0.25896307723613,0.09253715269228,0.04));
#49635=CARTESIAN_POINT('',(-0.257858961475997,0.095570685811709,0.04));
#49636=CARTESIAN_POINT('Origin',(0.,0.,0.04));
#49637=CARTESIAN_POINT('',(-0.252777314991409,0.0920034185546049,0.04));
#49638=CARTESIAN_POINT('',(-0.279603464135123,0.094318093935571,0.04));
#49639=CARTESIAN_POINT('',(-0.252777314991409,0.0920034185546049,0.04));
#49640=CARTESIAN_POINT('Origin',(-0.252777314991409,0.0920034185546049,
0.04));
#49641=CARTESIAN_POINT('',(-0.257858961475997,0.095570685811709,0.285));
#49642=CARTESIAN_POINT('',(-0.257858961475997,0.095570685811709,0.1425));
#49643=CARTESIAN_POINT('',(-0.252777314991409,0.0920034185546049,0.291));
#49644=CARTESIAN_POINT('',(-0.252777314991409,0.0920034185546049,0.04));
#49645=CARTESIAN_POINT('Ctrl Pts',(-0.257858961475997,0.095570685811709,
0.285));
#49646=CARTESIAN_POINT('Ctrl Pts',(-0.255290114447956,0.0937673797534397,
0.288035430631122));
#49647=CARTESIAN_POINT('Ctrl Pts',(-0.252777314991409,0.0920034185546049,
0.291));
#49648=CARTESIAN_POINT('Origin',(-0.279603464135123,0.094318093935571,0.04));
#49649=CARTESIAN_POINT('',(-0.25896307723613,0.09253715269228,0.285));
#49650=CARTESIAN_POINT('',(-0.25896307723613,0.09253715269228,0.1425));
#49651=CARTESIAN_POINT('Ctrl Pts',(-0.252777314991409,0.0920034185546049,
0.291));
#49652=CARTESIAN_POINT('Ctrl Pts',(-0.255836083454369,0.0922673422366571,
0.288035430631101));
#49653=CARTESIAN_POINT('Ctrl Pts',(-0.25896307723613,0.09253715269228,0.285));
#49654=CARTESIAN_POINT('Origin',(-0.244219163867212,0.141,0.04));
#49655=CARTESIAN_POINT('',(-0.238959938274539,0.136099771858106,0.04));
#49656=CARTESIAN_POINT('',(-0.237345829015656,0.138895491103459,0.04));
#49657=CARTESIAN_POINT('Origin',(0.,0.,0.04));
#49658=CARTESIAN_POINT('',(-0.232960833618014,0.1345,0.04));
#49659=CARTESIAN_POINT('',(-0.25897749411641,0.141437822173509,0.04));
#49660=CARTESIAN_POINT('',(-0.232960833618014,0.1345,0.04));
#49661=CARTESIAN_POINT('Origin',(-0.232960833618014,0.1345,0.04));
#49662=CARTESIAN_POINT('',(-0.237345829015656,0.138895491103459,0.285));
#49663=CARTESIAN_POINT('',(-0.237345829015656,0.138895491103459,0.1425));
#49664=CARTESIAN_POINT('',(-0.232960833618014,0.1345,0.291));
#49665=CARTESIAN_POINT('',(-0.232960833618014,0.1345,0.04));
#49666=CARTESIAN_POINT('Ctrl Pts',(-0.237345829015656,0.138895491103459,
0.285));
#49667=CARTESIAN_POINT('Ctrl Pts',(-0.23512914935695,0.136673505711114,
0.288035430631098));
#49668=CARTESIAN_POINT('Ctrl Pts',(-0.232960833618014,0.1345,0.291));
#49669=CARTESIAN_POINT('Origin',(-0.25897749411641,0.141437822173509,0.04));
#49670=CARTESIAN_POINT('',(-0.238959938274539,0.136099771858106,0.285));
#49671=CARTESIAN_POINT('',(-0.238959938274539,0.136099771858106,0.1425));
#49672=CARTESIAN_POINT('Ctrl Pts',(-0.232960833618014,0.1345,0.291));
#49673=CARTESIAN_POINT('Ctrl Pts',(-0.235927302648541,0.135291063657777,
0.288035430631136));
#49674=CARTESIAN_POINT('Ctrl Pts',(-0.238959938274539,0.136099771858106,
0.285));
#49675=CARTESIAN_POINT('Origin',(-0.216024532959552,0.181266105931604,0.04));
#49676=CARTESIAN_POINT('',(-0.211696122508039,0.175527068325832,0.04));
#49677=CARTESIAN_POINT('',(-0.209621063643459,0.17800002718254,0.04));
#49678=CARTESIAN_POINT('Origin',(0.,0.,0.04));
#49679=CARTESIAN_POINT('',(-0.206065955199005,0.172909867005679,0.04));
#49680=CARTESIAN_POINT('',(-0.230482623987904,0.184260033755696,0.04));
#49681=CARTESIAN_POINT('',(-0.206065955199005,0.172909867005679,0.04));
#49682=CARTESIAN_POINT('Origin',(-0.206065955199005,0.172909867005679,0.04));
#49683=CARTESIAN_POINT('',(-0.209621063643459,0.17800002718254,0.285));
#49684=CARTESIAN_POINT('',(-0.209621063643459,0.17800002718254,0.1425));
#49685=CARTESIAN_POINT('',(-0.206065955199005,0.172909867005679,0.291));
#49686=CARTESIAN_POINT('',(-0.206065955199005,0.172909867005679,0.04));
#49687=CARTESIAN_POINT('Ctrl Pts',(-0.209621063643459,0.17800002718254,
0.285));
#49688=CARTESIAN_POINT('Ctrl Pts',(-0.207823904043728,0.175426876357765,
0.288035430631226));
#49689=CARTESIAN_POINT('Ctrl Pts',(-0.206065955199005,0.172909867005679,
0.291));
#49690=CARTESIAN_POINT('Origin',(-0.230482623987904,0.184260033755696,0.04));
#49691=CARTESIAN_POINT('',(-0.211696122508039,0.175527068325832,0.285));
#49692=CARTESIAN_POINT('',(-0.211696122508039,0.175527068325832,0.1425));
#49693=CARTESIAN_POINT('Ctrl Pts',(-0.206065955199005,0.172909867005679,
0.291));
#49694=CARTESIAN_POINT('Ctrl Pts',(-0.208849990136858,0.174204034570293,
0.288035430631017));
#49695=CARTESIAN_POINT('Ctrl Pts',(-0.211696122508039,0.175527068325832,
0.285));
#49696=CARTESIAN_POINT('Origin',(-0.181266105931604,0.216024532959552,0.04));
#49697=CARTESIAN_POINT('',(-0.17800002718254,0.209621063643459,0.04));
#49698=CARTESIAN_POINT('',(-0.175527068325832,0.211696122508039,0.04));
#49699=CARTESIAN_POINT('Origin',(0.,0.,0.04));
#49700=CARTESIAN_POINT('',(-0.172909867005679,0.206065955199005,0.04));
#49701=CARTESIAN_POINT('',(-0.194984655959362,0.221483597452293,0.04));
#49702=CARTESIAN_POINT('',(-0.172909867005679,0.206065955199005,0.04));
#49703=CARTESIAN_POINT('Origin',(-0.172909867005679,0.206065955199005,0.04));
#49704=CARTESIAN_POINT('',(-0.175527068325832,0.211696122508039,0.285));
#49705=CARTESIAN_POINT('',(-0.175527068325832,0.211696122508039,0.1425));
#49706=CARTESIAN_POINT('',(-0.172909867005679,0.206065955199005,0.291));
#49707=CARTESIAN_POINT('',(-0.172909867005679,0.206065955199005,0.04));
#49708=CARTESIAN_POINT('Ctrl Pts',(-0.175527068325832,0.211696122508039,
0.285));
#49709=CARTESIAN_POINT('Ctrl Pts',(-0.174204034570238,0.208849990136741,
0.288035430631142));
#49710=CARTESIAN_POINT('Ctrl Pts',(-0.172909867005679,0.206065955199005,
0.291));
#49711=CARTESIAN_POINT('Origin',(-0.194984655959362,0.221483597452293,0.04));
#49712=CARTESIAN_POINT('',(-0.17800002718254,0.209621063643459,0.285));
#49713=CARTESIAN_POINT('',(-0.17800002718254,0.209621063643459,0.1425));
#49714=CARTESIAN_POINT('Ctrl Pts',(-0.172909867005679,0.206065955199005,
0.291));
#49715=CARTESIAN_POINT('Ctrl Pts',(-0.175426876357856,0.207823904043792,
0.288035430631119));
#49716=CARTESIAN_POINT('Ctrl Pts',(-0.17800002718254,0.209621063643459,
0.285));
#49717=CARTESIAN_POINT('Origin',(-0.141,0.244219163867212,0.04));
#49718=CARTESIAN_POINT('',(-0.138895491103459,0.237345829015656,0.04));
#49719=CARTESIAN_POINT('',(-0.136099771858106,0.238959938274539,0.04));
#49720=CARTESIAN_POINT('Origin',(0.,0.,0.04));
#49721=CARTESIAN_POINT('',(-0.1345,0.232960833618014,0.04));
#49722=CARTESIAN_POINT('',(-0.153562177826491,0.25197749411641,0.04));
#49723=CARTESIAN_POINT('',(-0.1345,0.232960833618014,0.04));
#49724=CARTESIAN_POINT('Origin',(-0.1345,0.232960833618014,0.04));
#49725=CARTESIAN_POINT('',(-0.136099771858106,0.238959938274539,0.285));
#49726=CARTESIAN_POINT('',(-0.136099771858106,0.238959938274539,0.1425));
#49727=CARTESIAN_POINT('',(-0.1345,0.232960833618014,0.291));
#49728=CARTESIAN_POINT('',(-0.1345,0.232960833618014,0.04));
#49729=CARTESIAN_POINT('Ctrl Pts',(-0.136099771858106,0.238959938274539,
0.285));
#49730=CARTESIAN_POINT('Ctrl Pts',(-0.135291063657772,0.235927302648521,
0.288035430631155));
#49731=CARTESIAN_POINT('Ctrl Pts',(-0.1345,0.232960833618014,0.291));
#49732=CARTESIAN_POINT('Origin',(-0.153562177826491,0.25197749411641,0.04));
#49733=CARTESIAN_POINT('',(-0.138895491103459,0.237345829015656,0.285));
#49734=CARTESIAN_POINT('',(-0.138895491103459,0.237345829015656,0.1425));
#49735=CARTESIAN_POINT('Ctrl Pts',(-0.1345,0.232960833618014,0.291));
#49736=CARTESIAN_POINT('Ctrl Pts',(-0.13667350571114,0.235129149356976,
0.288035430631063));
#49737=CARTESIAN_POINT('Ctrl Pts',(-0.138895491103459,0.237345829015656,
0.285));
#49738=CARTESIAN_POINT('Origin',(-0.0964496804178386,0.264993319061626,
0.04));
#49739=CARTESIAN_POINT('',(-0.095570685811709,0.257858961475997,0.04));
#49740=CARTESIAN_POINT('',(-0.09253715269228,0.25896307723613,0.04));
#49741=CARTESIAN_POINT('Origin',(0.,0.,0.04));
#49742=CARTESIAN_POINT('',(-0.0920034185546049,0.252777314991409,0.04));
#49743=CARTESIAN_POINT('',(-0.107473790626574,0.274815182128563,0.04));
#49744=CARTESIAN_POINT('',(-0.0920034185546049,0.252777314991409,0.04));
#49745=CARTESIAN_POINT('Origin',(-0.0920034185546049,0.252777314991409,
0.04));
#49746=CARTESIAN_POINT('',(-0.09253715269228,0.25896307723613,0.285));
#49747=CARTESIAN_POINT('',(-0.09253715269228,0.25896307723613,0.1425));
#49748=CARTESIAN_POINT('',(-0.0920034185546049,0.252777314991409,0.291));
#49749=CARTESIAN_POINT('',(-0.0920034185546049,0.252777314991409,0.04));
#49750=CARTESIAN_POINT('Ctrl Pts',(-0.09253715269228,0.25896307723613,0.285));
#49751=CARTESIAN_POINT('Ctrl Pts',(-0.0922673422366543,0.255836083454338,
0.288035430631132));
#49752=CARTESIAN_POINT('Ctrl Pts',(-0.0920034185546049,0.252777314991409,
0.291));
#49753=CARTESIAN_POINT('Origin',(-0.107473790626574,0.274815182128563,0.04));
#49754=CARTESIAN_POINT('',(-0.095570685811709,0.257858961475997,0.285));
#49755=CARTESIAN_POINT('',(-0.095570685811709,0.257858961475997,0.1425));
#49756=CARTESIAN_POINT('Ctrl Pts',(-0.0920034185546049,0.252777314991409,
0.291));
#49757=CARTESIAN_POINT('Ctrl Pts',(-0.0937673797534821,0.255290114448016,
0.288035430631051));
#49758=CARTESIAN_POINT('Ctrl Pts',(-0.0955706858117089,0.257858961475997,
0.285));
#49759=CARTESIAN_POINT('Origin',(-0.0489687861020744,0.277715786349443,
0.04));
#49760=CARTESIAN_POINT('',(-0.0493420135926708,0.27053717987482,0.04));
#49761=CARTESIAN_POINT('',(-0.0461628389679574,0.271097754137541,0.04));
#49762=CARTESIAN_POINT('Origin',(0.,0.,0.04));
#49763=CARTESIAN_POINT('',(-0.0467113597924043,0.264913285560284,0.04));
#49764=CARTESIAN_POINT('',(-0.0581198666828299,0.289302749894933,0.04));
#49765=CARTESIAN_POINT('',(-0.0467113597924043,0.264913285560284,0.04));
#49766=CARTESIAN_POINT('Origin',(-0.0467113597924043,0.264913285560284,
0.04));
#49767=CARTESIAN_POINT('',(-0.0461628389679574,0.271097754137541,0.285));
#49768=CARTESIAN_POINT('',(-0.0461628389679574,0.271097754137541,0.1425));
#49769=CARTESIAN_POINT('',(-0.0467113597924043,0.264913285560284,0.291));
#49770=CARTESIAN_POINT('',(-0.0467113597924043,0.264913285560284,0.04));
#49771=CARTESIAN_POINT('Ctrl Pts',(-0.0461628389679575,0.271097754137541,
0.285));
#49772=CARTESIAN_POINT('Ctrl Pts',(-0.0464401243112017,0.267971414323629,
0.288035430631178));
#49773=CARTESIAN_POINT('Ctrl Pts',(-0.0467113597924043,0.264913285560284,
0.291));
#49774=CARTESIAN_POINT('Origin',(-0.0581198666828299,0.289302749894933,
0.04));
#49775=CARTESIAN_POINT('',(-0.0493420135926708,0.27053717987482,0.285));
#49776=CARTESIAN_POINT('',(-0.0493420135926708,0.27053717987482,0.1425));
#49777=CARTESIAN_POINT('Ctrl Pts',(-0.0467113597924043,0.264913285560284,
0.291));
#49778=CARTESIAN_POINT('Ctrl Pts',(-0.0480121794105643,0.267694218594523,
0.288035430631107));
#49779=CARTESIAN_POINT('Ctrl Pts',(-0.0493420135926707,0.27053717987482,
0.285));
#49780=CARTESIAN_POINT('Origin',(1.38777878078145E-17,0.282,0.04));
#49781=CARTESIAN_POINT('',(-0.0016141092588829,0.274995262961565,0.04));
#49782=CARTESIAN_POINT('',(0.00161410925888293,0.274995262961565,0.04));
#49783=CARTESIAN_POINT('Origin',(0.,0.,0.04));
#49784=CARTESIAN_POINT('',(2.08166817117217E-17,0.269,0.04));
#49785=CARTESIAN_POINT('',(-0.00699999999999999,0.295,0.04));
#49786=CARTESIAN_POINT('',(2.08166817117217E-17,0.269,0.04));
#49787=CARTESIAN_POINT('Origin',(2.08166817117217E-17,0.269,0.04));
#49788=CARTESIAN_POINT('',(0.00161410925888295,0.274995262961565,0.285));
#49789=CARTESIAN_POINT('',(0.00161410925888295,0.274995262961565,0.1425));
#49790=CARTESIAN_POINT('',(2.08166817117217E-17,0.269,0.291));
#49791=CARTESIAN_POINT('',(2.08166817117217E-17,0.269,0.04));
#49792=CARTESIAN_POINT('Ctrl Pts',(0.00161410925888293,0.274995262961565,
0.285));
#49793=CARTESIAN_POINT('Ctrl Pts',(0.000798153291618306,0.271964569368868,
0.288035430631132));
#49794=CARTESIAN_POINT('Ctrl Pts',(2.08166817117217E-17,0.269,0.291));
#49795=CARTESIAN_POINT('Origin',(-0.00699999999999999,0.295,0.04));
#49796=CARTESIAN_POINT('',(-0.00161410925888292,0.274995262961565,0.285));
#49797=CARTESIAN_POINT('',(-0.00161410925888292,0.274995262961565,0.1425));
#49798=CARTESIAN_POINT('Ctrl Pts',(2.08166817117217E-17,0.269,0.291));
#49799=CARTESIAN_POINT('Ctrl Pts',(-0.000798153291634971,0.27196456936893,
0.28803543063107));
#49800=CARTESIAN_POINT('Ctrl Pts',(-0.00161410925888289,0.274995262961565,
0.285));
#49801=CARTESIAN_POINT('Origin',(0.0489687861020744,0.277715786349443,0.04));
#49802=CARTESIAN_POINT('',(0.0461628389679574,0.271097754137541,0.04));
#49803=CARTESIAN_POINT('',(0.0493420135926708,0.27053717987482,0.04));
#49804=CARTESIAN_POINT('Origin',(0.,0.,0.04));
#49805=CARTESIAN_POINT('',(0.0467113597924043,0.264913285560284,0.04));
#49806=CARTESIAN_POINT('',(0.044332558140659,0.29173382438227,0.04));
#49807=CARTESIAN_POINT('',(0.0467113597924043,0.264913285560284,0.04));
#49808=CARTESIAN_POINT('Origin',(0.0467113597924043,0.264913285560284,0.04));
#49809=CARTESIAN_POINT('',(0.0493420135926708,0.27053717987482,0.285));
#49810=CARTESIAN_POINT('',(0.0493420135926708,0.27053717987482,0.1425));
#49811=CARTESIAN_POINT('',(0.0467113597924043,0.264913285560284,0.291));
#49812=CARTESIAN_POINT('',(0.0467113597924043,0.264913285560284,0.04));
#49813=CARTESIAN_POINT('Ctrl Pts',(0.0493420135926708,0.27053717987482,
0.285));
#49814=CARTESIAN_POINT('Ctrl Pts',(0.048012179410518,0.267694218594424,
0.288035430631212));
#49815=CARTESIAN_POINT('Ctrl Pts',(0.0467113597924043,0.264913285560284,
0.291));
#49816=CARTESIAN_POINT('Origin',(0.044332558140659,0.29173382438227,0.04));
#49817=CARTESIAN_POINT('',(0.0461628389679575,0.271097754137541,0.285));
#49818=CARTESIAN_POINT('',(0.0461628389679575,0.271097754137541,0.1425));
#49819=CARTESIAN_POINT('Ctrl Pts',(0.0467113597924043,0.264913285560284,
0.291));
#49820=CARTESIAN_POINT('Ctrl Pts',(0.0464401243111968,0.267971414323684,
0.288035430631124));
#49821=CARTESIAN_POINT('Ctrl Pts',(0.0461628389679575,0.271097754137541,
0.285));
#49822=CARTESIAN_POINT('Origin',(0.0964496804178386,0.264993319061626,0.04));
#49823=CARTESIAN_POINT('',(0.09253715269228,0.25896307723613,0.04));
#49824=CARTESIAN_POINT('',(0.095570685811709,0.257858961475997,0.04));
#49825=CARTESIAN_POINT('Origin',(0.,0.,0.04));
#49826=CARTESIAN_POINT('',(0.0920034185546049,0.252777314991409,0.04));
#49827=CARTESIAN_POINT('',(0.094318093935571,0.279603464135123,0.04));
#49828=CARTESIAN_POINT('',(0.0920034185546049,0.252777314991409,0.04));
#49829=CARTESIAN_POINT('Origin',(0.0920034185546049,0.252777314991409,0.04));
#49830=CARTESIAN_POINT('',(0.095570685811709,0.257858961475997,0.285));
#49831=CARTESIAN_POINT('',(0.095570685811709,0.257858961475997,0.1425));
#49832=CARTESIAN_POINT('',(0.0920034185546049,0.252777314991409,0.291));
#49833=CARTESIAN_POINT('',(0.0920034185546049,0.252777314991409,0.04));
#49834=CARTESIAN_POINT('Ctrl Pts',(0.095570685811709,0.257858961475997,
0.285));
#49835=CARTESIAN_POINT('Ctrl Pts',(0.0937673797534397,0.255290114447956,
0.288035430631122));
#49836=CARTESIAN_POINT('Ctrl Pts',(0.0920034185546049,0.252777314991409,
0.291));
#49837=CARTESIAN_POINT('Origin',(0.094318093935571,0.279603464135123,0.04));
#49838=CARTESIAN_POINT('',(0.09253715269228,0.25896307723613,0.285));
#49839=CARTESIAN_POINT('',(0.09253715269228,0.25896307723613,0.1425));
#49840=CARTESIAN_POINT('Ctrl Pts',(0.0920034185546049,0.252777314991409,
0.291));
#49841=CARTESIAN_POINT('Ctrl Pts',(0.0922673422366571,0.255836083454369,
0.288035430631101));
#49842=CARTESIAN_POINT('Ctrl Pts',(0.09253715269228,0.25896307723613,0.285));
#49843=CARTESIAN_POINT('Origin',(0.141,0.244219163867212,0.04));
#49844=CARTESIAN_POINT('',(0.136099771858106,0.238959938274539,0.04));
#49845=CARTESIAN_POINT('',(0.138895491103459,0.237345829015656,0.04));
#49846=CARTESIAN_POINT('Origin',(0.,0.,0.04));
#49847=CARTESIAN_POINT('',(0.1345,0.232960833618014,0.04));
#49848=CARTESIAN_POINT('',(0.141437822173509,0.258977494116409,0.04));
#49849=CARTESIAN_POINT('',(0.1345,0.232960833618014,0.04));
#49850=CARTESIAN_POINT('Origin',(0.1345,0.232960833618014,0.04));
#49851=CARTESIAN_POINT('',(0.138895491103459,0.237345829015656,0.285));
#49852=CARTESIAN_POINT('',(0.138895491103459,0.237345829015656,0.1425));
#49853=CARTESIAN_POINT('',(0.1345,0.232960833618014,0.291));
#49854=CARTESIAN_POINT('',(0.1345,0.232960833618014,0.04));
#49855=CARTESIAN_POINT('Ctrl Pts',(0.138895491103459,0.237345829015656,
0.285));
#49856=CARTESIAN_POINT('Ctrl Pts',(0.136673505711127,0.235129149356963,
0.288035430631081));
#49857=CARTESIAN_POINT('Ctrl Pts',(0.1345,0.232960833618014,0.291));
#49858=CARTESIAN_POINT('Origin',(0.141437822173509,0.258977494116409,0.04));
#49859=CARTESIAN_POINT('',(0.136099771858106,0.238959938274539,0.285));
#49860=CARTESIAN_POINT('',(0.136099771858106,0.238959938274539,0.1425));
#49861=CARTESIAN_POINT('Ctrl Pts',(0.1345,0.232960833618014,0.291));
#49862=CARTESIAN_POINT('Ctrl Pts',(0.1352910636578,0.235927302648627,0.28803543063105));
#49863=CARTESIAN_POINT('Ctrl Pts',(0.136099771858106,0.238959938274539,
0.285));
#49864=CARTESIAN_POINT('Origin',(0.181266105931604,0.216024532959552,0.04));
#49865=CARTESIAN_POINT('',(0.175527068325832,0.211696122508039,0.04));
#49866=CARTESIAN_POINT('',(0.17800002718254,0.209621063643459,0.04));
#49867=CARTESIAN_POINT('Origin',(0.,0.,0.04));
#49868=CARTESIAN_POINT('',(0.172909867005679,0.206065955199005,0.04));
#49869=CARTESIAN_POINT('',(0.184260033755696,0.230482623987904,0.04));
#49870=CARTESIAN_POINT('',(0.172909867005679,0.206065955199005,0.04));
#49871=CARTESIAN_POINT('Origin',(0.172909867005679,0.206065955199005,0.04));
#49872=CARTESIAN_POINT('',(0.17800002718254,0.209621063643459,0.285));
#49873=CARTESIAN_POINT('',(0.17800002718254,0.209621063643459,0.1425));
#49874=CARTESIAN_POINT('',(0.172909867005679,0.206065955199005,0.291));
#49875=CARTESIAN_POINT('',(0.172909867005679,0.206065955199005,0.04));
#49876=CARTESIAN_POINT('Ctrl Pts',(0.17800002718254,0.209621063643459,0.285));
#49877=CARTESIAN_POINT('Ctrl Pts',(0.175426876357847,0.207823904043786,
0.28803543063113));
#49878=CARTESIAN_POINT('Ctrl Pts',(0.172909867005679,0.206065955199005,
0.291));
#49879=CARTESIAN_POINT('Origin',(0.184260033755696,0.230482623987904,0.04));
#49880=CARTESIAN_POINT('',(0.175527068325832,0.211696122508039,0.285));
#49881=CARTESIAN_POINT('',(0.175527068325832,0.211696122508039,0.1425));
#49882=CARTESIAN_POINT('Ctrl Pts',(0.172909867005679,0.206065955199005,
0.291));
#49883=CARTESIAN_POINT('Ctrl Pts',(0.174204034570257,0.208849990136781,
0.288035430631099));
#49884=CARTESIAN_POINT('Ctrl Pts',(0.175527068325832,0.211696122508039,
0.285));
#49885=CARTESIAN_POINT('Origin',(0.216024532959552,0.181266105931604,0.04));
#49886=CARTESIAN_POINT('',(0.209621063643459,0.17800002718254,0.04));
#49887=CARTESIAN_POINT('',(0.211696122508039,0.175527068325832,0.04));
#49888=CARTESIAN_POINT('Origin',(0.,0.,0.04));
#49889=CARTESIAN_POINT('',(0.206065955199005,0.172909867005679,0.04));
#49890=CARTESIAN_POINT('',(0.221483597452293,0.194984655959362,0.04));
#49891=CARTESIAN_POINT('',(0.206065955199005,0.172909867005679,0.04));
#49892=CARTESIAN_POINT('Origin',(0.206065955199005,0.172909867005679,0.04));
#49893=CARTESIAN_POINT('',(0.211696122508039,0.175527068325832,0.285));
#49894=CARTESIAN_POINT('',(0.211696122508039,0.175527068325832,0.1425));
#49895=CARTESIAN_POINT('',(0.206065955199005,0.172909867005679,0.291));
#49896=CARTESIAN_POINT('',(0.206065955199005,0.172909867005679,0.04));
#49897=CARTESIAN_POINT('Ctrl Pts',(0.211696122508039,0.175527068325832,
0.285));
#49898=CARTESIAN_POINT('Ctrl Pts',(0.208849990136656,0.174204034570199,
0.288035430631232));
#49899=CARTESIAN_POINT('Ctrl Pts',(0.206065955199005,0.172909867005679,
0.291));
#49900=CARTESIAN_POINT('Origin',(0.221483597452293,0.194984655959362,0.04));
#49901=CARTESIAN_POINT('',(0.209621063643459,0.17800002718254,0.285));
#49902=CARTESIAN_POINT('',(0.209621063643459,0.17800002718254,0.1425));
#49903=CARTESIAN_POINT('Ctrl Pts',(0.206065955199005,0.172909867005679,
0.291));
#49904=CARTESIAN_POINT('Ctrl Pts',(0.207823904043843,0.175426876357928,
0.288035430631034));
#49905=CARTESIAN_POINT('Ctrl Pts',(0.209621063643459,0.17800002718254,0.285));
#49906=CARTESIAN_POINT('Origin',(0.244219163867212,0.141,0.04));
#49907=CARTESIAN_POINT('',(0.237345829015656,0.138895491103459,0.04));
#49908=CARTESIAN_POINT('',(0.238959938274539,0.136099771858106,0.04));
#49909=CARTESIAN_POINT('Origin',(0.,0.,0.04));
#49910=CARTESIAN_POINT('',(0.232960833618014,0.1345,0.04));
#49911=CARTESIAN_POINT('',(0.25197749411641,0.153562177826491,0.04));
#49912=CARTESIAN_POINT('',(0.232960833618014,0.1345,0.04));
#49913=CARTESIAN_POINT('Origin',(0.232960833618014,0.1345,0.04));
#49914=CARTESIAN_POINT('',(0.238959938274539,0.136099771858106,0.285));
#49915=CARTESIAN_POINT('',(0.238959938274539,0.136099771858106,0.1425));
#49916=CARTESIAN_POINT('',(0.232960833618014,0.1345,0.291));
#49917=CARTESIAN_POINT('',(0.232960833618014,0.1345,0.04));
#49918=CARTESIAN_POINT('Ctrl Pts',(0.238959938274539,0.136099771858106,
0.285));
#49919=CARTESIAN_POINT('Ctrl Pts',(0.235927302648562,0.135291063657783,
0.288035430631114));
#49920=CARTESIAN_POINT('Ctrl Pts',(0.232960833618014,0.1345,0.291));
#49921=CARTESIAN_POINT('Origin',(0.25197749411641,0.153562177826491,0.04));
#49922=CARTESIAN_POINT('',(0.237345829015656,0.138895491103459,0.285));
#49923=CARTESIAN_POINT('',(0.237345829015656,0.138895491103459,0.1425));
#49924=CARTESIAN_POINT('Ctrl Pts',(0.232960833618014,0.1345,0.291));
#49925=CARTESIAN_POINT('Ctrl Pts',(0.235129149356992,0.136673505711156,
0.288035430631041));
#49926=CARTESIAN_POINT('Ctrl Pts',(0.237345829015656,0.138895491103459,
0.285));
#49927=CARTESIAN_POINT('Origin',(0.264993319061626,0.0964496804178386,0.04));
#49928=CARTESIAN_POINT('',(0.257858961475997,0.095570685811709,0.04));
#49929=CARTESIAN_POINT('',(0.25896307723613,0.09253715269228,0.04));
#49930=CARTESIAN_POINT('Origin',(0.,0.,0.04));
#49931=CARTESIAN_POINT('',(0.252777314991409,0.0920034185546049,0.04));
#49932=CARTESIAN_POINT('',(0.274815182128563,0.107473790626574,0.04));
#49933=CARTESIAN_POINT('',(0.252777314991409,0.0920034185546049,0.04));
#49934=CARTESIAN_POINT('Origin',(0.252777314991409,0.0920034185546049,0.04));
#49935=CARTESIAN_POINT('',(0.25896307723613,0.09253715269228,0.285));
#49936=CARTESIAN_POINT('',(0.25896307723613,0.09253715269228,0.1425));
#49937=CARTESIAN_POINT('',(0.252777314991409,0.0920034185546049,0.291));
#49938=CARTESIAN_POINT('',(0.252777314991409,0.0920034185546049,0.04));
#49939=CARTESIAN_POINT('Ctrl Pts',(0.25896307723613,0.09253715269228,0.285));
#49940=CARTESIAN_POINT('Ctrl Pts',(0.255836083454338,0.0922673422366543,
0.288035430631132));
#49941=CARTESIAN_POINT('Ctrl Pts',(0.252777314991409,0.0920034185546049,
0.291));
#49942=CARTESIAN_POINT('Origin',(0.274815182128563,0.107473790626574,0.04));
#49943=CARTESIAN_POINT('',(0.257858961475997,0.095570685811709,0.285));
#49944=CARTESIAN_POINT('',(0.257858961475997,0.095570685811709,0.1425));
#49945=CARTESIAN_POINT('Ctrl Pts',(0.252777314991409,0.0920034185546049,
0.291));
#49946=CARTESIAN_POINT('Ctrl Pts',(0.255290114448016,0.0937673797534821,
0.288035430631051));
#49947=CARTESIAN_POINT('Ctrl Pts',(0.257858961475997,0.0955706858117089,
0.285));
#49948=CARTESIAN_POINT('Origin',(0.277715786349443,0.0489687861020744,0.04));
#49949=CARTESIAN_POINT('',(0.27053717987482,0.0493420135926708,0.04));
#49950=CARTESIAN_POINT('',(0.271097754137541,0.0461628389679574,0.04));
#49951=CARTESIAN_POINT('Origin',(0.,0.,0.04));
#49952=CARTESIAN_POINT('',(0.264913285560284,0.0467113597924043,0.04));
#49953=CARTESIAN_POINT('',(0.289302749894933,0.0581198666828299,0.04));
#49954=CARTESIAN_POINT('',(0.264913285560284,0.0467113597924043,0.04));
#49955=CARTESIAN_POINT('Origin',(0.264913285560284,0.0467113597924043,0.04));
#49956=CARTESIAN_POINT('',(0.271097754137541,0.0461628389679574,0.285));
#49957=CARTESIAN_POINT('',(0.271097754137541,0.0461628389679574,0.1425));
#49958=CARTESIAN_POINT('',(0.264913285560284,0.0467113597924043,0.291));
#49959=CARTESIAN_POINT('',(0.264913285560284,0.0467113597924043,0.04));
#49960=CARTESIAN_POINT('Ctrl Pts',(0.271097754137541,0.0461628389679574,
0.285));
#49961=CARTESIAN_POINT('Ctrl Pts',(0.267971414323704,0.0464401243111951,
0.288035430631105));
#49962=CARTESIAN_POINT('Ctrl Pts',(0.264913285560284,0.0467113597924043,
0.291));
#49963=CARTESIAN_POINT('Origin',(0.289302749894933,0.0581198666828299,0.04));
#49964=CARTESIAN_POINT('',(0.27053717987482,0.0493420135926708,0.285));
#49965=CARTESIAN_POINT('',(0.27053717987482,0.0493420135926708,0.1425));
#49966=CARTESIAN_POINT('Ctrl Pts',(0.264913285560284,0.0467113597924043,
0.291));
#49967=CARTESIAN_POINT('Ctrl Pts',(0.26769421859449,0.0480121794105489,
0.288035430631142));
#49968=CARTESIAN_POINT('Ctrl Pts',(0.27053717987482,0.0493420135926708,
0.285));
#49969=CARTESIAN_POINT('Origin',(0.,0.,0.1425));
#49970=CARTESIAN_POINT('Origin',(0.,0.,0.285));
#49971=CARTESIAN_POINT('Origin',(0.,0.,0.285));
#49972=CARTESIAN_POINT('Origin',(0.,0.,0.285));
#49973=CARTESIAN_POINT('Origin',(0.,0.,0.285));
#49974=CARTESIAN_POINT('Origin',(0.,0.,0.285));
#49975=CARTESIAN_POINT('Origin',(0.,0.,0.285));
#49976=CARTESIAN_POINT('Origin',(0.,0.,0.285));
#49977=CARTESIAN_POINT('Origin',(0.,0.,0.285));
#49978=CARTESIAN_POINT('Origin',(0.,0.,0.285));
#49979=CARTESIAN_POINT('Origin',(0.,0.,0.285));
#49980=CARTESIAN_POINT('Origin',(0.,0.,0.285));
#49981=CARTESIAN_POINT('Origin',(0.,0.,0.285));
#49982=CARTESIAN_POINT('Origin',(0.,0.,0.285));
#49983=CARTESIAN_POINT('Origin',(0.,0.,0.285));
#49984=CARTESIAN_POINT('Origin',(0.,0.,0.285));
#49985=CARTESIAN_POINT('Origin',(0.,0.,0.285));
#49986=CARTESIAN_POINT('Origin',(0.,0.,0.285));
#49987=CARTESIAN_POINT('',(-0.275,-3.36777869765522E-17,0.));
#49988=CARTESIAN_POINT('',(-0.275,-3.36777869765522E-17,0.1425));
#49989=CARTESIAN_POINT('Origin',(0.,0.,0.));
#49990=CARTESIAN_POINT('Origin',(0.,0.,0.285));
#49991=CARTESIAN_POINT('Origin',(0.,0.,0.285));
#49992=CARTESIAN_POINT('Origin',(0.,0.,0.285));
#49993=CARTESIAN_POINT('Origin',(0.,0.,0.285));
#49994=CARTESIAN_POINT('Origin',(0.,0.,0.285));
#49995=CARTESIAN_POINT('Origin',(0.,0.,0.285));
#49996=CARTESIAN_POINT('Origin',(0.,0.,0.285));
#49997=CARTESIAN_POINT('Origin',(0.,0.,0.285));
#49998=CARTESIAN_POINT('Origin',(0.,0.,0.285));
#49999=CARTESIAN_POINT('Origin',(0.,0.,0.285));
#50000=CARTESIAN_POINT('Origin',(0.,0.,0.285));
#50001=CARTESIAN_POINT('Origin',(0.,0.,0.285));
#50002=CARTESIAN_POINT('Origin',(0.,0.,0.285));
#50003=CARTESIAN_POINT('Origin',(0.,0.,0.285));
#50004=CARTESIAN_POINT('Origin',(0.,0.,0.285));
#50005=CARTESIAN_POINT('Origin',(0.,0.,0.285));
#50006=CARTESIAN_POINT('Origin',(0.,0.,0.285));
#50007=CARTESIAN_POINT('',(0.274995262961565,0.00161410925888293,0.285));
#50008=CARTESIAN_POINT('Origin',(0.,0.,0.285));
#50009=CARTESIAN_POINT('',(0.274995262961565,0.00161410925888293,0.04));
#50010=CARTESIAN_POINT('',(0.274995262961565,0.00161410925888293,0.1425));
#50011=CARTESIAN_POINT('',(0.274995262961565,-0.00161410925888293,0.04));
#50012=CARTESIAN_POINT('Origin',(0.,0.,0.04));
#50013=CARTESIAN_POINT('',(0.274995262961565,-0.00161410925888293,0.285));
#50014=CARTESIAN_POINT('',(0.274995262961565,-0.00161410925888293,0.1425));
#50015=CARTESIAN_POINT('Origin',(0.,0.,0.285));
#50016=CARTESIAN_POINT('Origin',(0.269,0.,0.04));
#50017=CARTESIAN_POINT('',(0.269,0.,0.04));
#50018=CARTESIAN_POINT('',(0.269,0.,0.04));
#50019=CARTESIAN_POINT('',(0.269,0.,0.291));
#50020=CARTESIAN_POINT('',(0.269,0.,0.04));
#50021=CARTESIAN_POINT('Ctrl Pts',(0.274995262961565,-0.00161410925888293,
0.285));
#50022=CARTESIAN_POINT('Ctrl Pts',(0.271964569368838,-0.000798153291610108,
0.288035430631162));
#50023=CARTESIAN_POINT('Ctrl Pts',(0.269,0.,0.291));
#50024=CARTESIAN_POINT('Origin',(0.295,0.007,0.04));
#50025=CARTESIAN_POINT('Ctrl Pts',(0.269,0.,0.291));
#50026=CARTESIAN_POINT('Ctrl Pts',(0.27196456936891,0.000798153291629561,
0.28803543063109));
#50027=CARTESIAN_POINT('Ctrl Pts',(0.274995262961565,0.00161410925888293,
0.285));
#50028=CARTESIAN_POINT('',(0.295,0.007,0.04));
#50029=CARTESIAN_POINT('Origin',(0.282,0.,0.04));
#50030=CARTESIAN_POINT('Origin',(0.,0.,0.2925));
#50031=CARTESIAN_POINT('',(-0.26,-3.18408167778312E-17,0.3));
#50032=CARTESIAN_POINT('Origin',(0.,0.,0.3));
#50033=CARTESIAN_POINT('',(-0.2675,-3.27593018771917E-17,0.2925));
#50034=CARTESIAN_POINT('Origin',(0.,0.,0.134415608175648));
#50035=CARTESIAN_POINT('',(0.,0.,0.0978312163512968));
#50036=CARTESIAN_POINT('',(-0.113891921086774,1.39477376607661E-17,0.17));
#50037=CARTESIAN_POINT('',(-0.0577350269189626,-7.07050159149938E-18,0.134415608175648));
#50038=CARTESIAN_POINT('Origin',(0.,0.,0.17));
#50039=CARTESIAN_POINT('Origin',(0.,0.144337567297406,0.3));
#50040=CARTESIAN_POINT('',(8.83812698937423E-18,0.144337567297406,0.3));
#50041=CARTESIAN_POINT('',(0.125,0.0721687836487032,0.3));
#50042=CARTESIAN_POINT('',(0.03125,0.126295371385231,0.3));
#50043=CARTESIAN_POINT('',(1.38777878078145E-17,0.144337567297406,0.17));
#50044=CARTESIAN_POINT('',(8.83812698937423E-18,0.144337567297406,0.3));
#50045=CARTESIAN_POINT('',(0.125,0.0721687836487032,0.17));
#50046=CARTESIAN_POINT('',(0.125,0.0721687836487032,0.17));
#50047=CARTESIAN_POINT('',(0.125,0.0721687836487032,0.3));
#50048=CARTESIAN_POINT('Origin',(-0.125,0.0721687836487032,0.3));
#50049=CARTESIAN_POINT('',(-0.125,0.0721687836487032,0.3));
#50050=CARTESIAN_POINT('',(-0.09375,0.090210979560879,0.3));
#50051=CARTESIAN_POINT('',(-0.125,0.0721687836487032,0.17));
#50052=CARTESIAN_POINT('',(-0.125,0.0721687836487032,0.3));
#50053=CARTESIAN_POINT('',(8.83812698937423E-18,0.144337567297406,0.17));
#50054=CARTESIAN_POINT('Origin',(-0.125,-0.0721687836487032,0.3));
#50055=CARTESIAN_POINT('',(-0.125,-0.0721687836487032,0.3));
#50056=CARTESIAN_POINT('',(-0.125,-0.0360843918243516,0.3));
#50057=CARTESIAN_POINT('',(-0.125,-0.0721687836487032,0.17));
#50058=CARTESIAN_POINT('',(-0.125,-0.0721687836487032,0.3));
#50059=CARTESIAN_POINT('',(-0.125,0.0721687836487032,0.17));
#50060=CARTESIAN_POINT('Origin',(-2.77555756156289E-17,-0.144337567297406,
0.3));
#50061=CARTESIAN_POINT('',(-2.65143809681227E-17,-0.144337567297406,0.3));
#50062=CARTESIAN_POINT('',(-0.03125,-0.126295371385231,0.3));
#50063=CARTESIAN_POINT('',(-2.77555756156289E-17,-0.144337567297406,0.17));
#50064=CARTESIAN_POINT('',(-2.65143809681227E-17,-0.144337567297406,0.3));
#50065=CARTESIAN_POINT('',(-0.125,-0.0721687836487032,0.17));
#50066=CARTESIAN_POINT('Origin',(0.125,-0.0721687836487033,0.3));
#50067=CARTESIAN_POINT('',(0.125,-0.0721687836487033,0.3));
#50068=CARTESIAN_POINT('',(0.09375,-0.0902109795608791,0.3));
#50069=CARTESIAN_POINT('',(0.125,-0.0721687836487033,0.17));
#50070=CARTESIAN_POINT('',(0.125,-0.0721687836487033,0.3));
#50071=CARTESIAN_POINT('',(-2.65143809681227E-17,-0.144337567297406,0.17));
#50072=CARTESIAN_POINT('Origin',(0.125,0.0721687836487032,0.3));
#50073=CARTESIAN_POINT('',(0.125,0.0360843918243516,0.3));
#50074=CARTESIAN_POINT('',(0.125,-0.0721687836487033,0.17));
#50075=CARTESIAN_POINT('Origin',(0.,0.,0.17));
#50076=CARTESIAN_POINT('Origin',(0.114,0.,-3.));
#50077=CARTESIAN_POINT('',(-0.114,-1.39609735102798E-17,-3.));
#50078=CARTESIAN_POINT('Origin',(0.,0.,-3.));
#50079=CARTESIAN_POINT('Origin',(0.,0.,-2.982));
#50080=CARTESIAN_POINT('',(-0.132,-1.61653377487451E-17,-2.982));
#50081=CARTESIAN_POINT('Origin',(0.,0.,-1.487));
#50082=CARTESIAN_POINT('Origin',(0.,0.,-0.0136500000000002));
#50083=CARTESIAN_POINT('Origin',(0.,0.,-0.005));
#50084=CARTESIAN_POINT('',(-0.16,-1.95943487863577E-17,-2.60208521396521E-18));
#50085=CARTESIAN_POINT('Origin',(0.,0.,0.));
#50086=CARTESIAN_POINT('',(-0.155,-1.8982025386784E-17,-0.005));
#50087=CARTESIAN_POINT('Origin',(0.275,0.,0.));
#50088=CARTESIAN_POINT('Origin',(0.,0.,0.3));
#53630=UNCERTAINTY_MEASURE_WITH_UNIT(LENGTH_MEASURE(0.001),#53651,
'DISTANCE_ACCURACY_VALUE',
'Maximum model space distance between geometric entities at asserted c
onnectivities');
#53632=UNCERTAINTY_MEASURE_WITH_UNIT(LENGTH_MEASURE(0.001),#53651,
'DISTANCE_ACCURACY_VALUE',
'Maximum model space distance between geometric entities at asserted c
onnectivities');
#53648=(
GEOMETRIC_REPRESENTATION_CONTEXT(3)
GLOBAL_UNCERTAINTY_ASSIGNED_CONTEXT((#53630))
GLOBAL_UNIT_ASSIGNED_CONTEXT((#53651,#53653,#53654))
REPRESENTATION_CONTEXT('','3D')
);
#53650=(
GEOMETRIC_REPRESENTATION_CONTEXT(3)
GLOBAL_UNCERTAINTY_ASSIGNED_CONTEXT((#53632))
GLOBAL_UNIT_ASSIGNED_CONTEXT((#53651,#53653,#53654))
REPRESENTATION_CONTEXT('','3D')
);
#53651=(
LENGTH_UNIT()
NAMED_UNIT(*)
SI_UNIT(.CENTI.,.METRE.)
);
#53653=(
NAMED_UNIT(*)
PLANE_ANGLE_UNIT()
SI_UNIT($,.RADIAN.)
);
#53654=(
NAMED_UNIT(*)
SI_UNIT($,.STERADIAN.)
SOLID_ANGLE_UNIT()
);
#53670=SHAPE_DEFINITION_REPRESENTATION(#53687,#53738);
#53687=PRODUCT_DEFINITION_SHAPE('',$,#53756);
#53738=SHAPE_REPRESENTATION('',(#25038),#53648);
#53740=PRODUCT_DEFINITION_CONTEXT('part definition',#53793,'design');
#53756=PRODUCT_DEFINITION('2026-10-18-22-45-09-197',
'15_ISO_4762_M3x30_A2',#53773,#53740);
#53773=PRODUCT_DEFINITION_FORMATION('',$,#53810);
#53793=APPLICATION_CONTEXT(
'Core Data for Automotive Mechanical Design Process');
#53794=PRODUCT_CONTEXT('part definition',#53793,'mechanical');
#53810=PRODUCT('2026-10-18-22-45-09-197','15_ISO_4762_M3x30_A2',$,(#53794));
#53959=COLOUR_RGB('Black',0.12,0.14,0.17);
#53960=FILL_AREA_STYLE_COLOUR('',#53959);
#53961=FILL_AREA_STYLE('',(#53960));
#53962=SURFACE_STYLE_FILL_AREA(#53961);
#53963=SURFACE_SIDE_STYLE('',(#53962));
#53964=SURFACE_STYLE_USAGE(.BOTH.,#53963);
#53965=PRESENTATION_STYLE_ASSIGNMENT((#53964));
ENDSEC;
END-ISO-10303-21;
